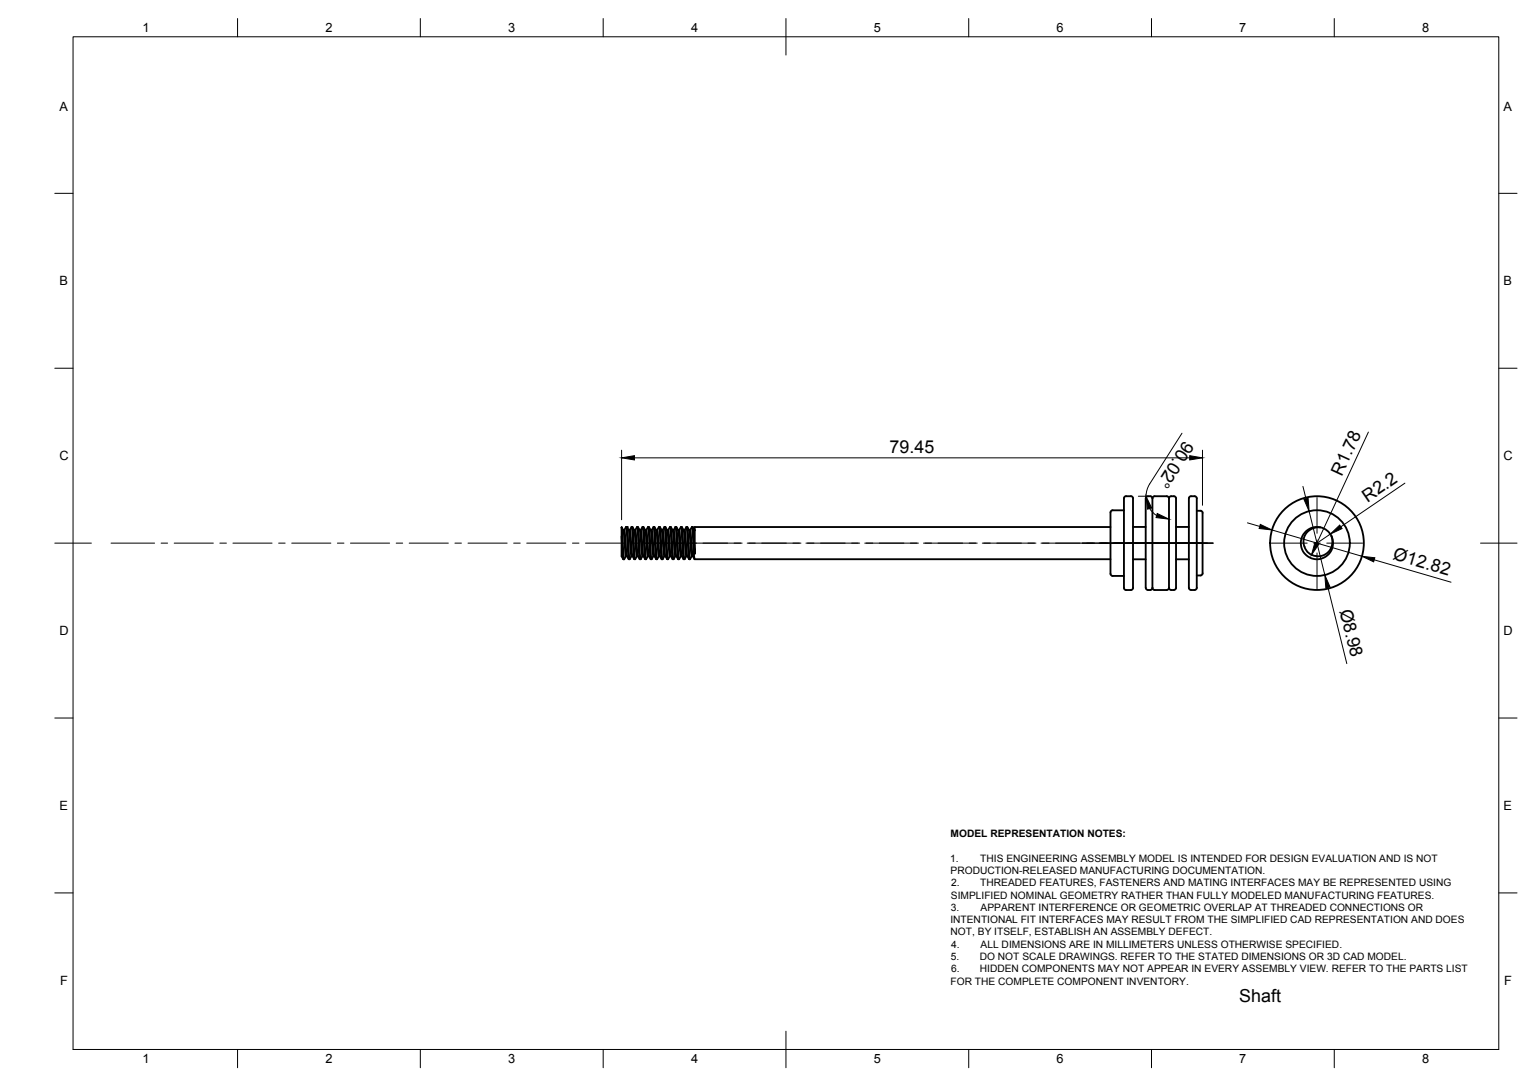
ISO-10303-21;
HEADER;
/* Generated by software containing ST-Developer
 * from STEP Tools, Inc. (www.steptools.com) 
 */

FILE_DESCRIPTION(
/* description */ (''),
/* implementation_level */ '2;1');

FILE_NAME(
/* name */ 'Shaft.step',
/* time_stamp */ '2026-10-06T13:05:37-07:00',
/* author */ (''),
/* organization */ (''),
/* preprocessor_version */ 'ST-DEVELOPER v20.2',
/* originating_system */ 'Autodesk Translation Framework v15.15.0.0',
/* authorisation */ '');

FILE_SCHEMA (('AUTOMOTIVE_DESIGN { 1 0 10303 214 3 1 1 }'));
ENDSEC;

DATA;
#10=MECHANICAL_DESIGN_GEOMETRIC_PRESENTATION_REPRESENTATION('',(#137),#28055);
#58=B_SPLINE_SURFACE_WITH_KNOTS('',3,3,((#14364,#14365,#14366,#14367,#14368,
#14369,#14370,#14371,#14372,#14373,#14374,#14375,#14376,#14377,#14378,#14379,
#14380,#14381,#14382,#14383,#14384,#14385,#14386,#14387,#14388,#14389,#14390,
#14391,#14392,#14393,#14394,#14395,#14396,#14397,#14398,#14399,#14400,#14401,
#14402,#14403,#14404,#14405,#14406,#14407,#14408,#14409,#14410,#14411,#14412,
#14413,#14414,#14415,#14416,#14417,#14418,#14419,#14420,#14421,#14422,#14423,
#14424,#14425,#14426,#14427,#14428,#14429,#14430,#14431,#14432,#14433,#14434,
#14435,#14436,#14437,#14438,#14439,#14440,#14441,#14442,#14443,#14444,#14445,
#14446,#14447,#14448,#14449,#14450,#14451,#14452),(#14453,#14454,#14455,
#14456,#14457,#14458,#14459,#14460,#14461,#14462,#14463,#14464,#14465,#14466,
#14467,#14468,#14469,#14470,#14471,#14472,#14473,#14474,#14475,#14476,#14477,
#14478,#14479,#14480,#14481,#14482,#14483,#14484,#14485,#14486,#14487,#14488,
#14489,#14490,#14491,#14492,#14493,#14494,#14495,#14496,#14497,#14498,#14499,
#14500,#14501,#14502,#14503,#14504,#14505,#14506,#14507,#14508,#14509,#14510,
#14511,#14512,#14513,#14514,#14515,#14516,#14517,#14518,#14519,#14520,#14521,
#14522,#14523,#14524,#14525,#14526,#14527,#14528,#14529,#14530,#14531,#14532,
#14533,#14534,#14535,#14536,#14537,#14538,#14539,#14540,#14541),(#14542,
#14543,#14544,#14545,#14546,#14547,#14548,#14549,#14550,#14551,#14552,#14553,
#14554,#14555,#14556,#14557,#14558,#14559,#14560,#14561,#14562,#14563,#14564,
#14565,#14566,#14567,#14568,#14569,#14570,#14571,#14572,#14573,#14574,#14575,
#14576,#14577,#14578,#14579,#14580,#14581,#14582,#14583,#14584,#14585,#14586,
#14587,#14588,#14589,#14590,#14591,#14592,#14593,#14594,#14595,#14596,#14597,
#14598,#14599,#14600,#14601,#14602,#14603,#14604,#14605,#14606,#14607,#14608,
#14609,#14610,#14611,#14612,#14613,#14614,#14615,#14616,#14617,#14618,#14619,
#14620,#14621,#14622,#14623,#14624,#14625,#14626,#14627,#14628,#14629,#14630),
(#14631,#14632,#14633,#14634,#14635,#14636,#14637,#14638,#14639,#14640,
#14641,#14642,#14643,#14644,#14645,#14646,#14647,#14648,#14649,#14650,#14651,
#14652,#14653,#14654,#14655,#14656,#14657,#14658,#14659,#14660,#14661,#14662,
#14663,#14664,#14665,#14666,#14667,#14668,#14669,#14670,#14671,#14672,#14673,
#14674,#14675,#14676,#14677,#14678,#14679,#14680,#14681,#14682,#14683,#14684,
#14685,#14686,#14687,#14688,#14689,#14690,#14691,#14692,#14693,#14694,#14695,
#14696,#14697,#14698,#14699,#14700,#14701,#14702,#14703,#14704,#14705,#14706,
#14707,#14708,#14709,#14710,#14711,#14712,#14713,#14714,#14715,#14716,#14717,
#14718,#14719)),.UNSPECIFIED.,.F.,.F.,.F.,(4,4),(4,1,1,1,1,1,1,1,1,1,1,
1,1,1,1,1,1,1,1,1,1,1,1,1,1,1,1,1,1,1,1,1,1,1,1,1,1,1,1,1,1,1,1,1,1,1,1,
1,1,1,1,1,1,1,1,1,1,1,1,1,1,1,1,1,1,1,1,1,1,1,1,1,1,1,1,1,1,1,1,1,1,1,1,
1,1,1,4),(-0.000373179544599254,0.0497114942005783),(13.3942556087771,14.3924503130856,
15.3906450173941,16.3888397217026,17.3870344260111,18.3852291303196,19.3834238346281,
20.3816185389366,21.3798132432451,22.3780079475536,23.3762026518621,24.3743973561706,
25.3725920604791,26.3707867647876,27.3689814690961,28.3671761734046,29.365370877713,
30.3635655820215,31.36176028633,32.3599549906385,33.358149694947,34.3563443992555,
35.354539103564,36.3527338078725,37.350928512181,38.3491232164895,39.347317920798,
40.3455126251065,41.343707329415,42.3419020337235,43.340096738032,44.3382914423405,
45.336486146649,46.3346808509575,47.332875555266,48.3310702595745,49.329264963883,
50.3274596681915,51.3256543725,52.3238490768085,53.322043781117,54.3202384854255,
55.318433189734,56.3166278940425,57.314822598351,58.3130173026595,59.311212006968,
60.3094067112765,61.307601415585,62.3057961198935,63.303990824202,64.3021855285105,
65.300380232819,66.2985749371275,67.296769641436,68.2949643457444,69.2931590500529,
70.2913537543614,71.2895484586699,72.2877431629784,73.2859378672869,74.2841325715954,
75.2823272759039,76.2805219802124,77.2787166845209,78.2769113888294,79.2751060931379,
80.2733007974464,81.2714955017549,82.2696902060634,83.2678849103719,84.2660796146804,
85.2642743189889,86.2624690232974,87.2606637276059,88.2588584319144,89.2570531362229,
90.2552478405314,91.2534425448399,92.2516372491484,93.2498319534569,94.2480266577654,
95.2462213620739,96.2444160663824,97.2426107706909,98.2408054749994,99.2393733588525),
 .UNSPECIFIED.);
#59=B_SPLINE_SURFACE_WITH_KNOTS('',3,3,((#14976,#14977,#14978,#14979,#14980,
#14981,#14982,#14983,#14984,#14985,#14986,#14987,#14988,#14989,#14990,#14991,
#14992,#14993,#14994,#14995,#14996,#14997,#14998,#14999,#15000,#15001,#15002,
#15003,#15004,#15005,#15006,#15007,#15008,#15009,#15010,#15011,#15012,#15013,
#15014,#15015,#15016,#15017,#15018,#15019,#15020,#15021,#15022,#15023,#15024,
#15025,#15026,#15027,#15028,#15029,#15030,#15031,#15032,#15033,#15034,#15035,
#15036,#15037,#15038,#15039,#15040,#15041,#15042,#15043,#15044,#15045,#15046,
#15047,#15048,#15049,#15050,#15051,#15052,#15053,#15054,#15055,#15056,#15057,
#15058,#15059,#15060,#15061,#15062,#15063,#15064),(#15065,#15066,#15067,
#15068,#15069,#15070,#15071,#15072,#15073,#15074,#15075,#15076,#15077,#15078,
#15079,#15080,#15081,#15082,#15083,#15084,#15085,#15086,#15087,#15088,#15089,
#15090,#15091,#15092,#15093,#15094,#15095,#15096,#15097,#15098,#15099,#15100,
#15101,#15102,#15103,#15104,#15105,#15106,#15107,#15108,#15109,#15110,#15111,
#15112,#15113,#15114,#15115,#15116,#15117,#15118,#15119,#15120,#15121,#15122,
#15123,#15124,#15125,#15126,#15127,#15128,#15129,#15130,#15131,#15132,#15133,
#15134,#15135,#15136,#15137,#15138,#15139,#15140,#15141,#15142,#15143,#15144,
#15145,#15146,#15147,#15148,#15149,#15150,#15151,#15152,#15153),(#15154,
#15155,#15156,#15157,#15158,#15159,#15160,#15161,#15162,#15163,#15164,#15165,
#15166,#15167,#15168,#15169,#15170,#15171,#15172,#15173,#15174,#15175,#15176,
#15177,#15178,#15179,#15180,#15181,#15182,#15183,#15184,#15185,#15186,#15187,
#15188,#15189,#15190,#15191,#15192,#15193,#15194,#15195,#15196,#15197,#15198,
#15199,#15200,#15201,#15202,#15203,#15204,#15205,#15206,#15207,#15208,#15209,
#15210,#15211,#15212,#15213,#15214,#15215,#15216,#15217,#15218,#15219,#15220,
#15221,#15222,#15223,#15224,#15225,#15226,#15227,#15228,#15229,#15230,#15231,
#15232,#15233,#15234,#15235,#15236,#15237,#15238,#15239,#15240,#15241,#15242),
(#15243,#15244,#15245,#15246,#15247,#15248,#15249,#15250,#15251,#15252,
#15253,#15254,#15255,#15256,#15257,#15258,#15259,#15260,#15261,#15262,#15263,
#15264,#15265,#15266,#15267,#15268,#15269,#15270,#15271,#15272,#15273,#15274,
#15275,#15276,#15277,#15278,#15279,#15280,#15281,#15282,#15283,#15284,#15285,
#15286,#15287,#15288,#15289,#15290,#15291,#15292,#15293,#15294,#15295,#15296,
#15297,#15298,#15299,#15300,#15301,#15302,#15303,#15304,#15305,#15306,#15307,
#15308,#15309,#15310,#15311,#15312,#15313,#15314,#15315,#15316,#15317,#15318,
#15319,#15320,#15321,#15322,#15323,#15324,#15325,#15326,#15327,#15328,#15329,
#15330,#15331)),.UNSPECIFIED.,.F.,.F.,.F.,(4,4),(4,1,1,1,1,1,1,1,1,1,1,
1,1,1,1,1,1,1,1,1,1,1,1,1,1,1,1,1,1,1,1,1,1,1,1,1,1,1,1,1,1,1,1,1,1,1,1,
1,1,1,1,1,1,1,1,1,1,1,1,1,1,1,1,1,1,1,1,1,1,1,1,1,1,1,1,1,1,1,1,1,1,1,1,
1,1,1,4),(-0.000317322289268298,0.0497654761150975),(16.7016191235447,17.7001869884391,
18.6983816927476,19.6965763970561,20.6947711013646,21.6929658056731,22.6911605099816,
23.6893552142901,24.6875499185986,25.6857446229071,26.6839393272156,27.6821340315241,
28.6803287358326,29.6785234401411,30.6767181444496,31.6749128487581,32.6731075530666,
33.6713022573751,34.6694969616836,35.6676916659921,36.6658863703006,37.6640810746091,
38.6622757789176,39.6604704832261,40.6586651875346,41.6568598918431,42.6550545961516,
43.65324930046,44.6514440047685,45.6496387090771,46.6478334133855,47.646028117694,
48.6442228220025,49.642417526311,50.6406122306195,51.638806934928,52.6370016392365,
53.635196343545,54.6333910478535,55.631585752162,56.6297804564705,57.627975160779,
58.6261698650875,59.624364569396,60.6225592737045,61.620753978013,62.6189486823215,
63.61714338663,64.6153380909385,65.613532795247,66.6117274995555,67.609922203864,
68.6081169081725,69.606311612481,70.6045063167895,71.602701021098,72.6008957254065,
73.599090429715,74.5972851340235,75.595479838332,76.5936745426405,77.591869246949,
78.5900639512575,79.588258655566,80.5864533598745,81.584648064183,82.5828427684915,
83.5810374728,84.5792321771085,85.577426881417,86.5756215857255,87.573816290034,
88.5720109943425,89.570205698651,90.5684004029595,91.566595107268,92.5647898115765,
93.562984515885,94.5611792201935,95.559373924502,96.5575686288105,97.555763333119,
98.5539580374275,99.552152741736,100.550347446044,101.548542150353,102.546736854661),
 .UNSPECIFIED.);
#98=TOROIDAL_SURFACE('',#3875,6.10845002480549,0.3);
#99=TOROIDAL_SURFACE('',#3881,6.107959450045,0.3);
#100=TOROIDAL_SURFACE('',#3887,4.18902817623056,0.3);
#101=TOROIDAL_SURFACE('',#3894,6.1096023907077,0.3);
#102=TOROIDAL_SURFACE('',#3901,6.10941276264524,0.3);
#103=TOROIDAL_SURFACE('',#3906,6.1087216021292,0.3);
#104=TOROIDAL_SURFACE('',#3914,6.1086273903848,0.3);
#105=TOROIDAL_SURFACE('',#3916,6.10778208446569,0.3);
#106=TOROIDAL_SURFACE('',#3921,6.10767319978801,0.3);
#107=TOROIDAL_SURFACE('',#3926,6.1069775362949,0.3);
#108=TOROIDAL_SURFACE('',#3934,6.10683442041659,0.3);
#109=TOROIDAL_SURFACE('',#3939,4.12329516333974,0.3);
#117=SHAPE_REPRESENTATION_RELATIONSHIP('SRR','None',#28094,#127);
#127=ADVANCED_BREP_SHAPE_REPRESENTATION('',(#147),#28046);
#137=STYLED_ITEM('',(#28152),#147);
#147=MANIFOLD_SOLID_BREP('Body1',#3678);
#164=CONICAL_SURFACE('',#3879,6.40820475053297,0.000295609290233083);
#165=CONICAL_SURFACE('',#3898,6.40950758978419,0.000295609290232241);
#166=CONICAL_SURFACE('',#3910,6.40867450936473,0.000295609290232273);
#167=CONICAL_SURFACE('',#3919,6.40772765523458,0.000295609290232245);
#168=CONICAL_SURFACE('',#3930,6.40690599146347,0.000295609290233429);
#181=FACE_BOUND('',#632,.T.);
#182=FACE_BOUND('',#635,.T.);
#183=FACE_BOUND('',#640,.T.);
#184=FACE_BOUND('',#648,.T.);
#185=FACE_BOUND('',#652,.T.);
#186=FACE_BOUND('',#655,.T.);
#187=FACE_BOUND('',#659,.T.);
#188=FACE_BOUND('',#665,.T.);
#189=FACE_BOUND('',#669,.T.);
#190=FACE_BOUND('',#672,.T.);
#209=PLANE('',#3872);
#210=PLANE('',#3883);
#211=PLANE('',#3885);
#212=PLANE('',#3886);
#213=PLANE('',#3893);
#214=PLANE('',#3900);
#215=PLANE('',#3904);
#216=PLANE('',#3912);
#217=PLANE('',#3924);
#218=PLANE('',#3932);
#219=PLANE('',#3937);
#220=PLANE('',#3943);
#280=CIRCLE('',#3853,1.77625);
#281=CIRCLE('',#3867,2.204);
#282=CIRCLE('',#3868,2.204);
#283=CIRCLE('',#3869,2.204);
#284=CIRCLE('',#3871,1.77625);
#285=CIRCLE('',#3873,6.107959450045);
#286=CIRCLE('',#3874,6.10778208446569);
#287=CIRCLE('',#3876,6.10845002480549);
#288=CIRCLE('',#3877,0.3);
#289=CIRCLE('',#3878,6.40845001169777);
#290=CIRCLE('',#3880,6.40795943693727);
#291=CIRCLE('',#3882,0.3);
#292=CIRCLE('',#3884,6.1086273903848);
#293=CIRCLE('',#3888,4.18902817623056);
#294=CIRCLE('',#3889,0.3);
#295=CIRCLE('',#3890,4.48902817623056);
#296=CIRCLE('',#3892,4.48902817623056);
#297=CIRCLE('',#3895,6.1096023907077);
#298=CIRCLE('',#3896,0.3);
#299=CIRCLE('',#3897,6.40960237759997);
#300=CIRCLE('',#3899,6.40941274953751);
#301=CIRCLE('',#3902,0.3);
#302=CIRCLE('',#3903,6.10941276264524);
#303=CIRCLE('',#3905,2.21164758166987);
#304=CIRCLE('',#3907,6.1087216021292);
#305=CIRCLE('',#3908,0.3);
#306=CIRCLE('',#3909,6.40872158902147);
#307=CIRCLE('',#3911,6.40862737727707);
#308=CIRCLE('',#3913,2.21164758166987);
#309=CIRCLE('',#3915,0.3);
#310=CIRCLE('',#3917,0.3);
#311=CIRCLE('',#3918,6.40778207135796);
#312=CIRCLE('',#3920,6.40767318668028);
#313=CIRCLE('',#3922,0.3);
#314=CIRCLE('',#3923,6.10767319978801);
#315=CIRCLE('',#3925,2.21164758166987);
#316=CIRCLE('',#3927,6.1069775362949);
#317=CIRCLE('',#3928,0.3);
#318=CIRCLE('',#3929,6.40697752318717);
#319=CIRCLE('',#3931,6.40683440730886);
#320=CIRCLE('',#3933,2.21164758166987);
#321=CIRCLE('',#3935,0.3);
#322=CIRCLE('',#3936,6.10683442041659);
#323=CIRCLE('',#3938,4.42329516333974);
#324=CIRCLE('',#3940,4.42329516333974);
#325=CIRCLE('',#3941,0.3);
#326=CIRCLE('',#3942,4.12329516333974);
#404=FACE_OUTER_BOUND('',#618,.T.);
#405=FACE_OUTER_BOUND('',#619,.T.);
#406=FACE_OUTER_BOUND('',#620,.T.);
#407=FACE_OUTER_BOUND('',#621,.T.);
#408=FACE_OUTER_BOUND('',#622,.T.);
#409=FACE_OUTER_BOUND('',#623,.T.);
#410=FACE_OUTER_BOUND('',#624,.T.);
#411=FACE_OUTER_BOUND('',#625,.T.);
#412=FACE_OUTER_BOUND('',#626,.T.);
#413=FACE_OUTER_BOUND('',#627,.T.);
#414=FACE_OUTER_BOUND('',#628,.T.);
#415=FACE_OUTER_BOUND('',#629,.T.);
#416=FACE_OUTER_BOUND('',#630,.T.);
#417=FACE_OUTER_BOUND('',#631,.T.);
#418=FACE_OUTER_BOUND('',#633,.T.);
#419=FACE_OUTER_BOUND('',#634,.T.);
#420=FACE_OUTER_BOUND('',#636,.T.);
#421=FACE_OUTER_BOUND('',#637,.T.);
#422=FACE_OUTER_BOUND('',#638,.T.);
#423=FACE_OUTER_BOUND('',#639,.T.);
#424=FACE_OUTER_BOUND('',#641,.T.);
#425=FACE_OUTER_BOUND('',#642,.T.);
#426=FACE_OUTER_BOUND('',#643,.T.);
#427=FACE_OUTER_BOUND('',#644,.T.);
#428=FACE_OUTER_BOUND('',#645,.T.);
#429=FACE_OUTER_BOUND('',#646,.T.);
#430=FACE_OUTER_BOUND('',#647,.T.);
#431=FACE_OUTER_BOUND('',#649,.T.);
#432=FACE_OUTER_BOUND('',#650,.T.);
#433=FACE_OUTER_BOUND('',#651,.T.);
#434=FACE_OUTER_BOUND('',#653,.T.);
#435=FACE_OUTER_BOUND('',#654,.T.);
#436=FACE_OUTER_BOUND('',#656,.T.);
#437=FACE_OUTER_BOUND('',#657,.T.);
#438=FACE_OUTER_BOUND('',#658,.T.);
#439=FACE_OUTER_BOUND('',#660,.T.);
#440=FACE_OUTER_BOUND('',#661,.T.);
#441=FACE_OUTER_BOUND('',#662,.T.);
#442=FACE_OUTER_BOUND('',#663,.T.);
#443=FACE_OUTER_BOUND('',#664,.T.);
#444=FACE_OUTER_BOUND('',#666,.T.);
#445=FACE_OUTER_BOUND('',#667,.T.);
#446=FACE_OUTER_BOUND('',#668,.T.);
#447=FACE_OUTER_BOUND('',#670,.T.);
#448=FACE_OUTER_BOUND('',#671,.T.);
#449=FACE_OUTER_BOUND('',#673,.T.);
#450=FACE_OUTER_BOUND('',#674,.T.);
#451=FACE_OUTER_BOUND('',#675,.T.);
#452=FACE_OUTER_BOUND('',#676,.T.);
#453=FACE_OUTER_BOUND('',#677,.T.);
#618=EDGE_LOOP('',(#2404,#2405,#2406,#2407,#2408));
#619=EDGE_LOOP('',(#2409,#2410,#2411,#2412,#2413));
#620=EDGE_LOOP('',(#2414,#2415,#2416,#2417,#2418,#2419));
#621=EDGE_LOOP('',(#2420,#2421,#2422,#2423,#2424,#2425));
#622=EDGE_LOOP('',(#2426,#2427,#2428,#2429,#2430));
#623=EDGE_LOOP('',(#2431,#2432,#2433,#2434,#2435));
#624=EDGE_LOOP('',(#2436,#2437,#2438,#2439,#2440));
#625=EDGE_LOOP('',(#2441,#2442,#2443,#2444,#2445));
#626=EDGE_LOOP('',(#2446,#2447,#2448,#2449,#2450));
#627=EDGE_LOOP('',(#2451,#2452,#2453,#2454,#2455));
#628=EDGE_LOOP('',(#2456,#2457,#2458,#2459,#2460));
#629=EDGE_LOOP('',(#2461,#2462,#2463,#2464,#2465));
#630=EDGE_LOOP('',(#2466,#2467,#2468,#2469,#2470,#2471));
#631=EDGE_LOOP('',(#2472));
#632=EDGE_LOOP('',(#2473,#2474,#2475,#2476,#2477,#2478,#2479,#2480,#2481,
#2482,#2483,#2484,#2485,#2486,#2487,#2488,#2489,#2490,#2491,#2492,#2493,
#2494,#2495,#2496,#2497,#2498,#2499,#2500,#2501,#2502,#2503));
#633=EDGE_LOOP('',(#2504,#2505,#2506,#2507,#2508,#2509));
#634=EDGE_LOOP('',(#2510));
#635=EDGE_LOOP('',(#2511));
#636=EDGE_LOOP('',(#2512,#2513,#2514,#2515));
#637=EDGE_LOOP('',(#2516,#2517,#2518,#2519));
#638=EDGE_LOOP('',(#2520,#2521,#2522,#2523));
#639=EDGE_LOOP('',(#2524));
#640=EDGE_LOOP('',(#2525));
#641=EDGE_LOOP('',(#2526,#2527,#2528,#2529,#2530,#2531,#2532,#2533,#2534,
#2535,#2536,#2537,#2538,#2539,#2540,#2541,#2542,#2543,#2544,#2545,#2546,
#2547,#2548,#2549,#2550,#2551,#2552,#2553,#2554,#2555,#2556,#2557,#2558,
#2559,#2560,#2561,#2562,#2563,#2564));
#642=EDGE_LOOP('',(#2565,#2566,#2567,#2568));
#643=EDGE_LOOP('',(#2569,#2570,#2571,#2572,#2573,#2574,#2575,#2576,#2577,
#2578,#2579,#2580,#2581,#2582,#2583,#2584,#2585,#2586,#2587,#2588,#2589,
#2590,#2591,#2592,#2593,#2594,#2595,#2596,#2597,#2598,#2599,#2600,#2601,
#2602,#2603,#2604,#2605,#2606,#2607,#2608));
#644=EDGE_LOOP('',(#2609,#2610,#2611,#2612));
#645=EDGE_LOOP('',(#2613,#2614,#2615,#2616));
#646=EDGE_LOOP('',(#2617,#2618,#2619,#2620));
#647=EDGE_LOOP('',(#2621));
#648=EDGE_LOOP('',(#2622));
#649=EDGE_LOOP('',(#2623,#2624,#2625,#2626));
#650=EDGE_LOOP('',(#2627,#2628,#2629,#2630));
#651=EDGE_LOOP('',(#2631));
#652=EDGE_LOOP('',(#2632));
#653=EDGE_LOOP('',(#2633,#2634,#2635,#2636));
#654=EDGE_LOOP('',(#2637));
#655=EDGE_LOOP('',(#2638));
#656=EDGE_LOOP('',(#2639,#2640,#2641,#2642));
#657=EDGE_LOOP('',(#2643,#2644,#2645,#2646));
#658=EDGE_LOOP('',(#2647));
#659=EDGE_LOOP('',(#2648));
#660=EDGE_LOOP('',(#2649,#2650,#2651,#2652));
#661=EDGE_LOOP('',(#2653,#2654,#2655,#2656));
#662=EDGE_LOOP('',(#2657,#2658,#2659,#2660));
#663=EDGE_LOOP('',(#2661,#2662,#2663,#2664));
#664=EDGE_LOOP('',(#2665));
#665=EDGE_LOOP('',(#2666));
#666=EDGE_LOOP('',(#2667,#2668,#2669,#2670));
#667=EDGE_LOOP('',(#2671,#2672,#2673,#2674));
#668=EDGE_LOOP('',(#2675));
#669=EDGE_LOOP('',(#2676));
#670=EDGE_LOOP('',(#2677,#2678,#2679,#2680));
#671=EDGE_LOOP('',(#2681));
#672=EDGE_LOOP('',(#2682));
#673=EDGE_LOOP('',(#2683,#2684,#2685,#2686));
#674=EDGE_LOOP('',(#2687));
#675=EDGE_LOOP('',(#2688,#2689,#2690,#2691));
#676=EDGE_LOOP('',(#2692,#2693,#2694,#2695));
#677=EDGE_LOOP('',(#2696,#2697,#2698,#2699));
#840=LINE('',#5074,#998);
#841=LINE('',#5346,#999);
#842=LINE('',#5736,#1000);
#843=LINE('',#5862,#1001);
#844=LINE('',#6173,#1002);
#845=LINE('',#6561,#1003);
#846=LINE('',#6960,#1004);
#847=LINE('',#7347,#1005);
#848=LINE('',#7748,#1006);
#849=LINE('',#8143,#1007);
#850=LINE('',#8552,#1008);
#851=LINE('',#8955,#1009);
#852=LINE('',#9337,#1010);
#853=LINE('',#14357,#1011);
#854=LINE('',#15429,#1012);
#855=LINE('',#15440,#1013);
#856=LINE('',#15458,#1014);
#857=LINE('',#15471,#1015);
#858=LINE('',#15488,#1016);
#859=LINE('',#15508,#1017);
#860=LINE('',#15510,#1018);
#861=LINE('',#15512,#1019);
#998=VECTOR('',#4239,1.77625);
#999=VECTOR('',#4244,1.77625);
#1000=VECTOR('',#4247,1.77625);
#1001=VECTOR('',#4250,1.77625);
#1002=VECTOR('',#4253,1.77625);
#1003=VECTOR('',#4256,1.77625);
#1004=VECTOR('',#4259,1.77625);
#1005=VECTOR('',#4262,1.77625);
#1006=VECTOR('',#4265,1.77625);
#1007=VECTOR('',#4268,1.77625);
#1008=VECTOR('',#4271,1.77625);
#1009=VECTOR('',#4274,1.77625);
#1010=VECTOR('',#4277,1.77625);
#1011=VECTOR('',#4306,6.40820475053297);
#1012=VECTOR('',#4331,4.48902817623056);
#1013=VECTOR('',#4346,6.40950758978419);
#1014=VECTOR('',#4371,6.40867450936473);
#1015=VECTOR('',#4390,6.40772765523458);
#1016=VECTOR('',#4413,6.40690599146347);
#1017=VECTOR('',#4442,4.42329516333974);
#1018=VECTOR('',#4445,2.21164758166987);
#1019=VECTOR('',#4448,2.21164758166987);
#1141=B_SPLINE_CURVE_WITH_KNOTS('',3,(#5076,#5077,#5078,#5079,#5080,#5081,
#5082,#5083,#5084,#5085,#5086,#5087,#5088,#5089,#5090,#5091,#5092,#5093,
#5094,#5095,#5096,#5097,#5098,#5099,#5100,#5101,#5102,#5103,#5104,#5105,
#5106,#5107,#5108,#5109,#5110,#5111,#5112,#5113,#5114,#5115,#5116,#5117,
#5118,#5119,#5120,#5121,#5122,#5123,#5124,#5125,#5126,#5127,#5128,#5129,
#5130,#5131,#5132,#5133,#5134,#5135,#5136,#5137,#5138,#5139,#5140,#5141,
#5142,#5143,#5144,#5145,#5146,#5147,#5148,#5149,#5150,#5151,#5152,#5153,
#5154,#5155,#5156,#5157,#5158,#5159,#5160,#5161,#5162,#5163,#5164,#5165,
#5166,#5167,#5168,#5169,#5170,#5171,#5172,#5173,#5174,#5175,#5176,#5177,
#5178,#5179,#5180,#5181,#5182,#5183,#5184,#5185,#5186,#5187,#5188,#5189,
#5190,#5191,#5192,#5193,#5194,#5195,#5196,#5197,#5198,#5199,#5200,#5201,
#5202,#5203,#5204,#5205,#5206,#5207,#5208,#5209,#5210,#5211,#5212,#5213,
#5214,#5215,#5216,#5217,#5218,#5219,#5220,#5221,#5222,#5223),
 .UNSPECIFIED.,.F.,.F.,(4,2,2,2,2,2,2,2,2,2,2,2,2,2,2,2,2,2,2,2,2,2,2,2,
2,2,2,2,2,2,2,2,2,2,2,2,2,2,2,2,2,2,2,2,2,2,2,2,2,2,2,2,2,2,2,2,2,2,2,2,
2,2,2,2,2,2,2,2,2,2,2,2,2,4),(-0.835356566537246,-0.834179578002919,-0.832057305629885,
-0.82934175770569,-0.823544728796445,-0.815449054574031,-0.790979904521206,
-0.758630520976316,-0.751247845401951,-0.746562671739766,-0.7427957472337,
-0.738457675321842,-0.730730673891037,-0.705406951032464,-0.667022076483651,
-0.660027153413853,-0.657302375275477,-0.655127611169892,-0.652797944555009,
-0.648926745100182,-0.632840827180127,-0.581115393054966,-0.57367752973655,
-0.568973506689807,-0.565200732382815,-0.560865809230101,-0.55317110435513,
-0.528123923872481,-0.491328745297315,-0.482817000286532,-0.479581086366103,
-0.477413245958042,-0.475106128977813,-0.471268591582215,-0.455353920220774,
-0.406196234245469,-0.39585526201539,-0.391035642446638,-0.38727899810539,
-0.3830778783461,-0.375924745588849,-0.367161529927778,-0.347550182457797,
-0.318343151462567,-0.305702905197989,-0.302000513660807,-0.299719364921067,
-0.297497437811916,-0.294122055897232,-0.283819597360589,-0.265015419181205,
-0.224003622448924,-0.216331810091993,-0.211947796786676,-0.20854279480949,
-0.204038955946528,-0.195556237330191,-0.184620571805917,-0.155613520886967,
-0.130863977628998,-0.12539325974147,-0.12272421983817,-0.12056335417637,
-0.117801735198089,-0.111949409671634,-0.0861381627528235,-0.0532557845040427,
-0.0423421159714301,-0.0374256406153841,-0.0335867130961813,-0.0300163926963186,
-0.0258468770318152,-0.0165211006533095,-0.000528019587408642),
 .UNSPECIFIED.);
#1142=B_SPLINE_CURVE_WITH_KNOTS('',3,(#5225,#5226,#5227,#5228,#5229,#5230,
#5231),.UNSPECIFIED.,.F.,.F.,(4,3,4),(15.4636264665944,15.5857948670228,
15.7079632674512),.UNSPECIFIED.);
#1143=B_SPLINE_CURVE_WITH_KNOTS('',3,(#5234,#5235,#5236,#5237,#5238,#5239,
#5240,#5241,#5242,#5243,#5244,#5245,#5246,#5247,#5248,#5249,#5250,#5251,
#5252,#5253,#5254,#5255,#5256,#5257,#5258,#5259,#5260,#5261,#5262,#5263,
#5264,#5265,#5266,#5267,#5268,#5269,#5270,#5271,#5272,#5273,#5274,#5275,
#5276,#5277,#5278,#5279,#5280,#5281,#5282,#5283,#5284,#5285,#5286,#5287,
#5288,#5289,#5290,#5291,#5292,#5293,#5294,#5295,#5296,#5297,#5298,#5299,
#5300,#5301,#5302,#5303,#5304,#5305,#5306,#5307,#5308,#5309,#5310,#5311,
#5312,#5313,#5314,#5315,#5316,#5317,#5318,#5319,#5320,#5321,#5322,#5323,
#5324,#5325,#5326,#5327,#5328,#5329,#5330,#5331,#5332,#5333,#5334,#5335,
#5336,#5337,#5338,#5339,#5340,#5341,#5342),.UNSPECIFIED.,.F.,.F.,(4,3,3,
3,3,3,3,3,3,3,3,3,3,3,3,3,3,3,3,3,3,3,3,3,3,3,3,3,3,3,3,3,3,3,3,3,4),(16.7019922841306,
16.8124544772726,16.9234210411684,17.033796869599,17.1441744311209,17.2545854631975,
17.3659858445079,17.4766375907132,17.5884122895762,17.7001869884391,17.8072802155964,
17.9186679002403,18.0254288144202,18.1321132984658,18.2387615669814,18.3454137772225,
18.4521802784855,18.5590147146697,18.6660336585631,18.6983816927476,18.8065090728564,
18.9177674883813,19.025595407644,19.1333563054358,19.2410888397907,19.3488316227747,
19.4566913005886,19.5646218816293,19.6727314597256,19.6965763970561,19.8047706499335,
19.912813978709,20.0207451306855,20.1286177204737,20.2364557658273,20.3443346961532,
20.3930532338378),.UNSPECIFIED.);
#1144=B_SPLINE_CURVE_WITH_KNOTS('',3,(#5347,#5348,#5349,#5350,#5351,#5352,
#5353,#5354,#5355,#5356,#5357,#5358,#5359,#5360,#5361,#5362,#5363,#5364,
#5365,#5366,#5367,#5368,#5369,#5370,#5371,#5372,#5373,#5374,#5375,#5376,
#5377,#5378,#5379,#5380,#5381,#5382,#5383,#5384,#5385,#5386,#5387,#5388,
#5389,#5390,#5391,#5392,#5393,#5394,#5395,#5396,#5397,#5398,#5399,#5400,
#5401,#5402,#5403,#5404,#5405,#5406,#5407,#5408,#5409,#5410,#5411,#5412,
#5413,#5414,#5415,#5416,#5417,#5418,#5419,#5420,#5421,#5422,#5423,#5424,
#5425,#5426,#5427,#5428,#5429,#5430,#5431,#5432,#5433,#5434,#5435,#5436,
#5437,#5438,#5439,#5440,#5441,#5442,#5443,#5444,#5445,#5446,#5447,#5448,
#5449,#5450,#5451,#5452,#5453,#5454,#5455,#5456,#5457,#5458,#5459,#5460,
#5461,#5462,#5463,#5464,#5465,#5466,#5467,#5468,#5469,#5470,#5471,#5472,
#5473,#5474,#5475,#5476,#5477,#5478,#5479,#5480,#5481,#5482,#5483,#5484,
#5485,#5486,#5487,#5488,#5489,#5490,#5491,#5492,#5493,#5494,#5495,#5496,
#5497,#5498,#5499,#5500,#5501,#5502,#5503,#5504,#5505,#5506,#5507,#5508,
#5509,#5510,#5511,#5512,#5513,#5514,#5515,#5516,#5517,#5518,#5519,#5520,
#5521,#5522,#5523,#5524,#5525,#5526,#5527,#5528,#5529,#5530,#5531,#5532,
#5533,#5534,#5535,#5536,#5537,#5538,#5539,#5540),.UNSPECIFIED.,.F.,.F.,
(4,2,2,2,2,2,2,2,2,2,2,2,2,2,2,2,2,2,2,2,2,2,2,2,2,2,2,2,2,2,2,2,2,2,2,
2,2,2,2,2,2,2,2,2,2,2,2,2,2,2,2,2,2,2,2,2,2,2,2,2,2,2,2,2,2,2,2,2,2,2,2,
2,2,2,2,2,2,2,2,2,2,2,2,2,2,2,2,2,2,2,2,2,2,2,2,2,4),(-1.95454507750439,
-1.92969887688555,-1.90700587487671,-1.90284449273311,-1.90045698570642,
-1.89829258749123,-1.89520508387779,-1.88936360059004,-1.85017890081121,
-1.82470793213726,-1.81696215744342,-1.81262184818882,-1.80885764965132,
-1.80418199299687,-1.79682683246125,-1.76279416764177,-1.73956966484566,
-1.73169570283323,-1.72601764868932,-1.72332439775519,-1.72120226710614,
-1.71856614706167,-1.7131897934261,-1.68420858229177,-1.66980886534623,
-1.65294595377729,-1.64134625560956,-1.63629734544878,-1.63249199363362,
-1.62836280128111,-1.62163051869468,-1.59092369606964,-1.5680581423284,
-1.55098317581711,-1.54705937226041,-1.54472310228857,-1.54256020421295,
-1.53987248019897,-1.53309414208251,-1.49446663046274,-1.46909648525411,
-1.46136459634652,-1.45702729073491,-1.45326306026007,-1.44858395184908,
-1.44121641047095,-1.40788434579373,-1.3841471969067,-1.37618087956058,
-1.37045355392296,-1.3677512422959,-1.36562903738565,-1.3630016479163,-1.35767008544244,
-1.3177711925292,-1.29148760005246,-1.28363221952914,-1.27926932868241,
-1.27550681445262,-1.27086060774184,-1.26360717745568,-1.22625306573836,
-1.2053446946898,-1.19438739470466,-1.19094604449721,-1.18871382456224,
-1.18643941074527,-1.18280332363237,-1.17100933713551,-1.13755203671263,
-1.12000271682831,-1.10834732008514,-1.10366159282688,-1.09980654930369,
-1.09585161550517,-1.08996582836221,-1.07189826280532,-1.03983979736194,
-1.01808202486886,-1.01388329213852,-1.01148758987828,-1.00932756295218,
-1.00626130276856,-0.998311944972997,-0.985704858969611,-0.961762341328657,
-0.933727639097285,-0.927057916080415,-0.922943834088199,-0.919137263230214,
-0.914064099371912,-0.902299995493179,-0.885082792620805,-0.873876918369987,
-0.842062810475459,-0.836793926929779,-0.835356566537246),.UNSPECIFIED.);
#1145=B_SPLINE_CURVE_WITH_KNOTS('',3,(#5542,#5543,#5544,#5545,#5546,#5547,
#5548,#5549,#5550,#5551,#5552,#5553,#5554,#5555,#5556,#5557,#5558,#5559,
#5560,#5561,#5562,#5563,#5564,#5565,#5566,#5567,#5568,#5569,#5570,#5571,
#5572,#5573,#5574,#5575,#5576,#5577,#5578,#5579,#5580,#5581,#5582,#5583,
#5584,#5585,#5586,#5587,#5588,#5589,#5590),.UNSPECIFIED.,.F.,.F.,(4,3,3,
3,3,3,3,3,3,3,3,3,3,3,3,3,4),(20.3930532338378,20.5010566943853,20.6092613750708,
20.6947711013646,20.8026970972416,20.9139806857955,21.0216059003609,21.1291641701826,
21.2366944839657,21.3442357847572,21.4518963786598,21.5596290516459,21.6675442181706,
21.6929658056731,21.8250574021607,21.9552551911513,21.9911485745994),
 .UNSPECIFIED.);
#1146=B_SPLINE_CURVE_WITH_KNOTS('',3,(#5591,#5592,#5593,#5594,#5595,#5596,
#5597,#5598,#5599,#5600,#5601,#5602,#5603,#5604,#5605,#5606,#5607,#5608,
#5609,#5610,#5611,#5612,#5613,#5614,#5615,#5616,#5617,#5618,#5619,#5620,
#5621,#5622,#5623,#5624,#5625,#5626,#5627,#5628,#5629,#5630,#5631,#5632,
#5633,#5634,#5635,#5636,#5637,#5638,#5639,#5640,#5641,#5642,#5643,#5644,
#5645,#5646,#5647,#5648,#5649,#5650,#5651,#5652,#5653,#5654,#5655,#5656,
#5657,#5658,#5659,#5660,#5661,#5662,#5663,#5664,#5665,#5666,#5667,#5668,
#5669,#5670,#5671,#5672,#5673,#5674,#5675,#5676,#5677,#5678,#5679,#5680,
#5681,#5682,#5683,#5684,#5685,#5686,#5687,#5688,#5689,#5690,#5691,#5692,
#5693,#5694,#5695,#5696,#5697,#5698,#5699,#5700,#5701,#5702,#5703,#5704,
#5705,#5706,#5707,#5708,#5709,#5710,#5711,#5712,#5713,#5714,#5715,#5716,
#5717,#5718,#5719,#5720,#5721,#5722,#5723,#5724,#5725,#5726,#5727,#5728,
#5729,#5730,#5731,#5732),.UNSPECIFIED.,.F.,.F.,(4,3,3,3,3,3,3,3,3,3,3,3,
3,3,3,3,3,3,3,3,3,3,3,3,3,3,3,3,3,3,3,3,3,3,3,3,3,3,3,3,3,3,3,3,3,3,3,4),
(21.9911485751285,22.0981765274336,22.2051623507136,22.3121457608551,22.4192405673634,
22.5263967550779,22.6337465274261,22.6911605099816,22.7992205091258,22.9104873472713,
23.0182513855477,23.1259498862704,23.2336216180078,23.3413053050867,23.4491088121582,
23.5569848760485,23.6650428436122,23.6893552142901,23.7973810979624,23.9086522005419,
24.0163805862326,24.1240429630528,24.2316781568489,24.3393249487448,24.4470912677292,
24.5549299286194,24.6629505155869,24.6875499185986,24.7955941221079,24.9068629347078,
25.0146102076539,25.1222916298659,25.2299459967969,25.3376120593305,25.4453976697339,
25.5532556566589,25.6612954465704,25.6857446229071,25.7937879777517,25.904155195045,
26.0119016507377,26.1195817394621,26.2272342594645,26.3396071236228,26.4473901517118,
26.5552467306643,26.6632787454227,26.6767257160977),.UNSPECIFIED.);
#1147=B_SPLINE_CURVE_WITH_KNOTS('',3,(#5738,#5739,#5740,#5741,#5742,#5743,
#5744,#5745,#5746),.UNSPECIFIED.,.F.,.F.,(4,1,1,1,1,1,4),(28.274333882308,
28.3671761734046,29.365370877713,30.3635655820215,31.36176028633,32.3599549906385,
32.9594405895371),.UNSPECIFIED.);
#1148=B_SPLINE_CURVE_WITH_KNOTS('',3,(#5747,#5748,#5749,#5750,#5751,#5752,
#5753,#5754,#5755,#5756,#5757,#5758,#5759,#5760,#5761,#5762,#5763,#5764,
#5765,#5766,#5767,#5768,#5769,#5770,#5771,#5772,#5773,#5774,#5775,#5776,
#5777,#5778,#5779,#5780,#5781,#5782,#5783,#5784,#5785,#5786,#5787,#5788,
#5789,#5790,#5791,#5792,#5793,#5794,#5795,#5796),.UNSPECIFIED.,.F.,.F.,
(4,2,2,2,2,2,2,2,2,2,2,2,2,2,2,2,2,2,2,2,2,2,2,2,4),(-2.23915986394093,
-2.20592704873654,-2.18032577745133,-2.17256259015734,-2.16821888680587,
-2.16445526260495,-2.15978487840366,-2.15244732829037,-2.1175945351571,
-2.09496188142004,-2.08719720497901,-2.08157791702537,-2.07889578751457,
-2.07677406554045,-2.0741280407893,-2.06869901710893,-2.04323247885477,
-2.02010812726836,-1.99943956922362,-1.99331541844904,-1.98931322858529,
-1.98549354859668,-1.98011485708538,-1.96718673212748,-1.95454507750439),
 .UNSPECIFIED.);
#1149=B_SPLINE_CURVE_WITH_KNOTS('',3,(#5798,#5799,#5800,#5801,#5802,#5803,
#5804,#5805,#5806,#5807,#5808,#5809,#5810,#5811,#5812,#5813,#5814,#5815,
#5816,#5817,#5818,#5819,#5820,#5821,#5822,#5823,#5824,#5825,#5826,#5827,
#5828,#5829,#5830,#5831,#5832,#5833,#5834,#5835,#5836,#5837,#5838,#5839,
#5840,#5841,#5842,#5843,#5844,#5845,#5846,#5847,#5848,#5849),
 .UNSPECIFIED.,.F.,.F.,(4,3,3,3,3,3,3,3,3,3,3,3,3,3,3,3,3,4),(26.6767257160977,
26.6839393272156,26.7919782863231,26.9032477544733,27.0109896752984,27.1186657202993,
27.2263146935872,27.3339753546827,27.4417555868768,27.5496082029795,27.6576426811105,
27.6821340315241,27.7919683102848,27.9016171368834,28.0110886501516,28.1204564526687,
28.2297536032295,28.274333882308),.UNSPECIFIED.);
#1150=B_SPLINE_CURVE_WITH_KNOTS('',3,(#5850,#5851,#5852,#5853,#5854,#5855,
#5856,#5857,#5858),.UNSPECIFIED.,.F.,.F.,(4,1,1,1,1,1,4),(28.2743402347403,
28.6803287358326,29.6785234401411,30.6767181444496,31.6749128487581,32.6731075530666,
32.9608271762519),.UNSPECIFIED.);
#1151=B_SPLINE_CURVE_WITH_KNOTS('',3,(#5864,#5865,#5866,#5867,#5868,#5869,
#5870,#5871,#5872,#5873,#5874,#5875,#5876,#5877,#5878,#5879,#5880,#5881,
#5882,#5883,#5884,#5885,#5886,#5887,#5888,#5889,#5890,#5891,#5892,#5893,
#5894,#5895,#5896,#5897,#5898,#5899,#5900,#5901,#5902,#5903,#5904,#5905,
#5906,#5907,#5908,#5909,#5910,#5911,#5912,#5913,#5914,#5915,#5916,#5917,
#5918,#5919,#5920,#5921,#5922,#5923,#5924,#5925,#5926,#5927,#5928,#5929,
#5930,#5931,#5932,#5933,#5934,#5935,#5936,#5937,#5938,#5939,#5940,#5941,
#5942,#5943,#5944,#5945,#5946,#5947,#5948,#5949,#5950,#5951,#5952,#5953,
#5954,#5955,#5956,#5957,#5958,#5959,#5960,#5961,#5962,#5963,#5964,#5965,
#5966,#5967,#5968,#5969,#5970,#5971,#5972,#5973,#5974,#5975,#5976,#5977,
#5978,#5979,#5980,#5981,#5982,#5983,#5984,#5985,#5986,#5987,#5988,#5989,
#5990,#5991,#5992,#5993,#5994,#5995,#5996,#5997,#5998,#5999,#6000,#6001,
#6002,#6003,#6004,#6005),.UNSPECIFIED.,.F.,.F.,(4,3,3,3,3,3,3,3,3,3,3,3,
3,3,3,3,3,3,3,3,3,3,3,3,3,3,3,3,3,3,3,3,3,3,3,3,3,3,3,3,3,3,3,3,3,3,3,4),
(34.5575193977698,34.6637962689209,34.7699803795124,34.8761126116981,34.9822337650756,
35.088455256206,35.194732459932,35.3011944966565,35.354539103564,35.4625799721229,
35.5738492015916,35.681593103219,35.7892711499964,35.8969221428487,36.0045848381315,
36.112367113131,36.2202217794645,36.3282583002447,36.3527338078725,36.4607746770588,
36.5720439064491,36.6797878087295,36.7874658561678,36.8951168496875,37.0027795456435,
37.1105618213201,37.2184164883337,37.3264530097926,37.350928512181,37.4589693811155,
37.5702386105372,37.6779825125593,37.7856605597373,37.8933115529956,38.000974248689,
38.1087565241035,38.216611190855,38.324647712054,38.3491232164895,38.4608178024709,
38.568667102327,38.6764084850113,38.7840808451954,38.8917229858393,38.9994241461165,
39.1071616534688,39.2150320522313,39.2426799043403),.UNSPECIFIED.);
#1152=B_SPLINE_CURVE_WITH_KNOTS('',3,(#6006,#6007,#6008,#6009,#6010,#6011),
 .UNSPECIFIED.,.F.,.F.,(4,1,1,4),(32.9594405895371,33.358149694947,34.3563443992555,
34.5575191894877),.UNSPECIFIED.);
#1153=B_SPLINE_CURVE_WITH_KNOTS('',3,(#6013,#6014,#6015,#6016,#6017),
 .UNSPECIFIED.,.F.,.F.,(4,1,4),(32.9608271762519,33.6713022573751,34.5575102647709),
 .UNSPECIFIED.);
#1154=B_SPLINE_CURVE_WITH_KNOTS('',3,(#6018,#6019,#6020,#6021,#6022,#6023,
#6024,#6025,#6026,#6027,#6028,#6029,#6030,#6031,#6032,#6033,#6034,#6035,
#6036,#6037,#6038,#6039,#6040,#6041,#6042,#6043,#6044,#6045,#6046,#6047,
#6048,#6049,#6050,#6051,#6052,#6053,#6054,#6055,#6056,#6057,#6058,#6059,
#6060,#6061,#6062,#6063,#6064,#6065,#6066,#6067,#6068,#6069,#6070,#6071,
#6072,#6073,#6074,#6075,#6076,#6077,#6078,#6079,#6080,#6081,#6082,#6083,
#6084,#6085,#6086,#6087,#6088,#6089,#6090,#6091,#6092,#6093,#6094,#6095,
#6096,#6097,#6098,#6099,#6100,#6101,#6102,#6103,#6104,#6105,#6106,#6107,
#6108,#6109,#6110,#6111,#6112,#6113,#6114,#6115,#6116,#6117,#6118,#6119,
#6120,#6121,#6122,#6123,#6124,#6125,#6126,#6127,#6128,#6129,#6130,#6131,
#6132,#6133,#6134,#6135,#6136,#6137,#6138,#6139,#6140,#6141,#6142,#6143,
#6144,#6145,#6146,#6147,#6148,#6149,#6150,#6151,#6152,#6153,#6154,#6155,
#6156,#6157,#6158,#6159,#6160,#6161,#6162,#6163,#6164,#6165,#6166,#6167,
#6168,#6169),.UNSPECIFIED.,.F.,.F.,(4,2,2,2,2,2,2,2,2,2,2,2,2,2,2,2,2,2,
2,2,2,2,2,2,2,2,2,2,2,2,2,2,2,2,2,2,2,2,2,2,2,2,2,2,2,2,2,2,2,2,2,2,2,2,
2,2,2,2,2,2,2,2,2,2,2,2,2,2,2,2,2,2,2,2,2,4),(-2.23888494972284,-2.22991776855793,
-2.22447064320661,-2.22191829216988,-2.21989477343009,-2.21776847377992,
-2.21502874476971,-2.20893402279126,-2.18787843436243,-2.16966634347861,
-2.14385238080136,-2.13606038366673,-2.13171077947681,-2.12794768118234,
-2.12328524358438,-2.11390205737419,-2.07246864712722,-2.05027458125105,
-2.04489827929598,-2.04226229222838,-2.04035089005686,-2.03776646712269,
-2.0328105326407,-1.99791659798478,-1.96864883524523,-1.95927121403217,
-1.95460974539526,-1.95084658102242,-1.94649595728929,-1.93891035281729,
-1.89754680244139,-1.87904083706616,-1.86884897296706,-1.86549209633338,
-1.86327753791409,-1.86098243262719,-1.85724781425568,-1.84435404247657,
-1.80361547729748,-1.78470675362083,-1.77873969519656,-1.77476942506272,
-1.77092850577831,-1.76629564503759,-1.75480186338448,-1.71587013709037,
-1.69449471669221,-1.6892066322397,-1.68658769916922,-1.68467704547633,
-1.68207654389007,-1.67688276164301,-1.64448591367606,-1.63262573013931,
-1.61610562983729,-1.60466923401097,-1.59964695878773,-1.59584552599926,
-1.59170494698949,-1.5849177429812,-1.554669575998,-1.53244795233212,-1.51446840999572,
-1.51049555511708,-1.50814869586371,-1.50599106650872,-1.50332518743687,
-1.49656138600397,-1.45787430738769,-1.43249347062081,-1.42475990429867,
-1.42042205696215,-1.41665756715559,-1.4119784002815,-1.4046112824739,-1.40437359183403),
 .UNSPECIFIED.);
#1155=B_SPLINE_CURVE_WITH_KNOTS('',3,(#6175,#6176,#6177,#6178,#6179,#6180,
#6181,#6182,#6183,#6184,#6185,#6186,#6187,#6188,#6189,#6190,#6191,#6192,
#6193,#6194,#6195,#6196,#6197,#6198,#6199,#6200,#6201,#6202,#6203,#6204,
#6205,#6206,#6207,#6208,#6209,#6210,#6211,#6212,#6213,#6214,#6215,#6216,
#6217,#6218,#6219,#6220,#6221,#6222,#6223,#6224,#6225,#6226,#6227,#6228,
#6229,#6230,#6231,#6232,#6233,#6234,#6235,#6236,#6237,#6238,#6239,#6240,
#6241,#6242,#6243,#6244,#6245,#6246,#6247,#6248,#6249,#6250,#6251,#6252,
#6253,#6254,#6255,#6256,#6257,#6258,#6259,#6260,#6261,#6262,#6263,#6264,
#6265,#6266,#6267,#6268,#6269,#6270,#6271,#6272,#6273,#6274,#6275,#6276,
#6277,#6278,#6279,#6280,#6281,#6282,#6283,#6284,#6285,#6286,#6287,#6288,
#6289,#6290,#6291,#6292,#6293,#6294,#6295,#6296,#6297,#6298,#6299,#6300,
#6301,#6302,#6303,#6304,#6305,#6306,#6307,#6308,#6309,#6310,#6311,#6312,
#6313,#6314,#6315,#6316,#6317,#6318,#6319,#6320,#6321,#6322),
 .UNSPECIFIED.,.F.,.F.,(4,2,2,2,2,2,2,2,2,2,2,2,2,2,2,2,2,2,2,2,2,2,2,2,
2,2,2,2,2,2,2,2,2,2,2,2,2,2,2,2,2,2,2,2,2,2,2,2,2,2,2,2,2,2,2,2,2,2,2,2,
2,2,2,2,2,2,2,2,2,2,2,2,2,4),(-0.835099924428374,-0.810230319348001,-0.804896130565269,
-0.802268377014195,-0.800146299250092,-0.797444671956707,-0.791720718154825,
-0.783761495584802,-0.76005780011584,-0.726728468131525,-0.719363533194796,
-0.714685219878248,-0.71092110576457,-0.70658334156592,-0.69884901195783,
-0.673458960429975,-0.634756499650488,-0.627989293535211,-0.625322962005017,
-0.623165325271974,-0.620818865337488,-0.616847515854485,-0.59888758745142,
-0.576676092912076,-0.54644768251051,-0.539660204241827,-0.535519716308051,
-0.531718510580919,-0.526696749457739,-0.515262844600596,-0.498745486707646,
-0.487103824026872,-0.454413034292759,-0.449239542055546,-0.446643067818346,
-0.444732272546319,-0.442109216499667,-0.436799720433161,-0.415227032788622,
-0.375690485550125,-0.364600414407815,-0.359688848510703,-0.355891171960493,
-0.35173917187912,-0.344896737736136,-0.336636791651806,-0.318863385154281,
-0.284112077379857,-0.273620116100306,-0.270127168635037,-0.268106390492079,
-0.265898441440772,-0.262574397053666,-0.252664479586328,-0.234986866661226,
-0.19213003390502,-0.184740608673265,-0.180432716329455,-0.176701275542952,
-0.171998743506043,-0.16240040782514,-0.138024613707217,-0.10870919764151,
-0.0962332329690868,-0.0925351436016178,-0.0902480445649851,-0.0880276089129058,
-0.0846416658687451,-0.074190627067205,-0.0548973537364689,-0.0155466790190831,
-0.00753311737622712,-0.00341159348289976,-0.000525934153839705),
 .UNSPECIFIED.);
#1156=B_SPLINE_CURVE_WITH_KNOTS('',3,(#6323,#6324,#6325,#6326,#6327,#6328,
#6329,#6330,#6331,#6332,#6333,#6334,#6335,#6336,#6337,#6338,#6339,#6340,
#6341,#6342,#6343,#6344,#6345,#6346,#6347,#6348,#6349,#6350,#6351,#6352,
#6353,#6354,#6355,#6356,#6357,#6358,#6359,#6360,#6361,#6362,#6363,#6364,
#6365,#6366,#6367,#6368,#6369,#6370,#6371),.UNSPECIFIED.,.F.,.F.,(4,3,3,
3,3,3,3,3,3,3,3,3,3,3,3,3,4),(39.2426799043403,39.347317920798,39.4553587897862,
39.5666280192012,39.6743719212775,39.7820499685097,39.8897009618222,39.9973636575694,
40.1051459330372,40.2130005998416,40.3210371210927,40.3455126251065,40.4593059977434,
40.5727552393315,40.6859938246744,40.798974097679,40.8407044963078),
 .UNSPECIFIED.);
#1157=B_SPLINE_CURVE_WITH_KNOTS('',3,(#6372,#6373,#6374,#6375,#6376,#6377,
#6378,#6379,#6380,#6381,#6382,#6383,#6384,#6385,#6386,#6387,#6388,#6389,
#6390,#6391,#6392,#6393,#6394,#6395,#6396,#6397,#6398,#6399,#6400,#6401,
#6402,#6403,#6404,#6405,#6406,#6407,#6408,#6409,#6410,#6411,#6412,#6413,
#6414,#6415,#6416,#6417,#6418,#6419,#6420,#6421,#6422,#6423,#6424,#6425,
#6426,#6427,#6428,#6429,#6430,#6431,#6432,#6433,#6434,#6435,#6436,#6437,
#6438,#6439,#6440,#6441,#6442,#6443,#6444,#6445,#6446,#6447,#6448,#6449,
#6450,#6451,#6452,#6453,#6454,#6455,#6456,#6457,#6458,#6459,#6460,#6461,
#6462,#6463,#6464,#6465,#6466,#6467,#6468,#6469,#6470,#6471,#6472,#6473,
#6474,#6475,#6476,#6477,#6478,#6479,#6480,#6481,#6482,#6483,#6484,#6485,
#6486,#6487,#6488,#6489,#6490,#6491,#6492,#6493,#6494,#6495,#6496,#6497,
#6498,#6499,#6500,#6501,#6502,#6503,#6504,#6505,#6506,#6507,#6508,#6509,
#6510,#6511,#6512,#6513,#6514,#6515,#6516,#6517,#6518,#6519,#6520,#6521,
#6522,#6523,#6524,#6525,#6526,#6527,#6528,#6529,#6530,#6531,#6532,#6533,
#6534,#6535,#6536,#6537,#6538,#6539,#6540,#6541,#6542,#6543,#6544,#6545,
#6546,#6547,#6548,#6549,#6550,#6551,#6552,#6553,#6554,#6555,#6556,#6557),
 .UNSPECIFIED.,.F.,.F.,(4,2,2,2,2,2,2,2,2,2,2,2,2,2,2,2,2,2,2,2,2,2,2,2,
2,2,2,2,2,2,2,2,2,2,2,2,2,2,2,2,2,2,2,2,2,2,2,2,2,2,2,2,2,2,2,2,2,2,2,2,
2,2,2,2,2,2,2,2,2,2,2,2,2,2,2,2,2,2,2,2,2,2,2,2,2,2,2,2,2,2,2,2,4),(-1.40437359183403,
-1.37123442544774,-1.34752963779357,-1.33956894550668,-1.33384453706723,
-1.33114265739486,-1.32902037709875,-1.32639236697421,-1.32105767193388,
-1.28990184687834,-1.27710833130175,-1.26053819930053,-1.24907775154556,
-1.24405147443566,-1.24024940402294,-1.23611045005564,-1.22933132030553,
-1.1991424444891,-1.17718888992443,-1.16481053221377,-1.15695984650571,
-1.15390650964041,-1.15174763436364,-1.14934515565329,-1.14511413330171,
-1.1199654897537,-1.07619341358872,-1.06892966170554,-1.06464923613406,
-1.0612555821067,-1.05667875748375,-1.04774607909163,-1.0360187374714,-1.00243054455778,
-0.981420876710011,-0.977242959541184,-0.974851927051027,-0.972688952611354,
-0.969609890907095,-0.96158130833031,-0.948791070416998,-0.911037219829708,
-0.895295885708175,-0.889507924932764,-0.88596636520286,-0.882113005965861,
-0.876761106568744,-0.863143851728035,-0.841650542388842,-0.80749697430888,
-0.800992055473671,-0.798368262274408,-0.796220606248343,-0.793852062063708,
-0.789778743192625,-0.769603171631479,-0.724976386629526,-0.714953988896045,
-0.710174271931691,-0.706401887754161,-0.702133000275573,-0.694731715330455,
-0.662688812809577,-0.627098897825888,-0.622213482154788,-0.619643997664196,
-0.617538915753009,-0.614779745974369,-0.608740756103967,-0.600182111874869,
-0.572873372681339,-0.544179070275189,-0.536835062276827,-0.532162650611676,
-0.528398714254533,-0.524056114345843,-0.5162990981695,-0.490744904305246,
-0.451146436953167,-0.445598441642736,-0.44288337641325,-0.44071350468291,
-0.438389667197007,-0.434523083461308,-0.418400108311522,-0.366386013304921,
-0.358997698073502,-0.354312637345431,-0.350548095703286,-0.346215342549465,
-0.338505260339425,-0.310188566919195,-0.285073042962578),.UNSPECIFIED.);
#1158=B_SPLINE_CURVE_WITH_KNOTS('',3,(#6562,#6563,#6564,#6565,#6566,#6567,
#6568,#6569,#6570,#6571,#6572,#6573,#6574,#6575,#6576,#6577,#6578,#6579,
#6580,#6581,#6582,#6583,#6584,#6585,#6586,#6587,#6588,#6589,#6590,#6591,
#6592,#6593,#6594,#6595,#6596,#6597,#6598,#6599,#6600,#6601,#6602,#6603,
#6604,#6605,#6606,#6607,#6608,#6609,#6610,#6611,#6612,#6613,#6614,#6615,
#6616,#6617,#6618,#6619,#6620,#6621,#6622,#6623,#6624,#6625,#6626,#6627,
#6628,#6629,#6630,#6631,#6632,#6633,#6634,#6635,#6636,#6637,#6638,#6639,
#6640,#6641,#6642,#6643,#6644,#6645,#6646,#6647,#6648,#6649,#6650,#6651,
#6652,#6653,#6654,#6655,#6656,#6657,#6658,#6659,#6660,#6661,#6662,#6663,
#6664,#6665,#6666,#6667,#6668,#6669,#6670,#6671,#6672,#6673,#6674,#6675,
#6676,#6677,#6678,#6679,#6680,#6681,#6682,#6683,#6684,#6685,#6686,#6687,
#6688,#6689,#6690,#6691,#6692,#6693,#6694,#6695,#6696,#6697,#6698,#6699,
#6700,#6701,#6702,#6703,#6704,#6705,#6706,#6707,#6708,#6709,#6710,#6711,
#6712,#6713,#6714,#6715,#6716,#6717,#6718,#6719,#6720,#6721,#6722,#6723,
#6724,#6725,#6726,#6727,#6728,#6729,#6730,#6731,#6732,#6733,#6734,#6735,
#6736,#6737,#6738,#6739,#6740,#6741,#6742,#6743,#6744,#6745,#6746,#6747,
#6748,#6749,#6750,#6751),.UNSPECIFIED.,.F.,.F.,(4,2,2,2,2,2,2,2,2,2,2,2,
2,2,2,2,2,2,2,2,2,2,2,2,2,2,2,2,2,2,2,2,2,2,2,2,2,2,2,2,2,2,2,2,2,2,2,2,
2,2,2,2,2,2,2,2,2,2,2,2,2,2,2,2,2,2,2,2,2,2,2,2,2,2,2,2,2,2,2,2,2,2,2,2,
2,2,2,2,2,2,2,2,2,2,4),(-1.95419705041876,-1.95099509657436,-1.94335603423285,
-1.89991425942924,-1.87506559070961,-1.87085029414465,-1.86845141700778,
-1.86629169624077,-1.86323154906988,-1.85589494163826,-1.80915527702303,
-1.78941037574571,-1.78336666657204,-1.77938126023139,-1.77555177097439,
-1.77011478780303,-1.75687520202681,-1.71971687152613,-1.69894795789413,
-1.69372753446967,-1.69112204521488,-1.68899928354412,-1.6862729303428,
-1.68061920244923,-1.64560251554659,-1.62383557245409,-1.61010952998578,
-1.60474301590359,-1.60088747043224,-1.59734954579938,-1.59158053314671,
-1.57599794538798,-1.53805844930273,-1.5252395640355,-1.51719964584465,
-1.51411912755031,-1.51195609974106,-1.50956606370411,-1.50539209599044,
-1.48448455657626,-1.45085051616374,-1.43911885055448,-1.43018312798703,
-1.42560600193481,-1.42221257001728,-1.41793303258227,-1.41067227172661,
-1.36685718427406,-1.34377191808452,-1.33830282624568,-1.33564914858626,
-1.33352753047315,-1.3308533889611,-1.32527638798234,-1.28500681146791,
-1.25934693277238,-1.25157594831113,-1.24723074868244,-1.24346741272986,
-1.23879943896024,-1.2314698664428,-1.1962869213581,-1.17389058740369,-1.16617028239694,
-1.16057494815006,-1.15789737507523,-1.15577576095328,-1.15312549402477,
-1.14767412692595,-1.11976092188052,-1.08198674324006,-1.07476016775468,
-1.07012217598063,-1.06636070172582,-1.06199273348142,-1.05411036107367,
-1.02761652170471,-1.00975943176876,-0.986126109116485,-0.981905770012072,
-0.979505779977728,-0.977346392827614,-0.974288562634894,-0.966405257133201,
-0.953952236184314,-0.930399287942635,-0.901801161853786,-0.89511851665121,
-0.891000170280617,-0.887191963350469,-0.882119951237423,-0.870373676231296,
-0.853196610132522,-0.841453580091553,-0.835099924428374),.UNSPECIFIED.);
#1159=B_SPLINE_CURVE_WITH_KNOTS('',3,(#6753,#6754,#6755,#6756,#6757,#6758,
#6759,#6760,#6761,#6762,#6763,#6764,#6765,#6766,#6767,#6768,#6769,#6770,
#6771,#6772,#6773,#6774,#6775,#6776,#6777,#6778,#6779,#6780,#6781,#6782,
#6783,#6784,#6785,#6786,#6787,#6788,#6789,#6790,#6791,#6792,#6793,#6794,
#6795,#6796,#6797,#6798,#6799,#6800,#6801,#6802,#6803,#6804,#6805,#6806,
#6807,#6808),.UNSPECIFIED.,.F.,.F.,(4,2,2,2,2,2,2,2,2,2,2,2,2,2,2,2,2,2,
2,2,2,2,2,2,2,2,2,4),(-0.285073042962578,-0.279553666108781,-0.268860677228453,
-0.265344191924806,-0.263318928126342,-0.261115262971523,-0.257812524684666,
-0.248081258600964,-0.230913628765321,-0.187069317157601,-0.179816393831322,
-0.175538464730903,-0.172144677675042,-0.167564926100631,-0.1586163724922,
-0.1468608393431,-0.113089336365138,-0.0923072130143463,-0.0881367138826751,
-0.0857473423440587,-0.0835838714087559,-0.0805013269290881,-0.072447874665844,
-0.0595990213919607,-0.0169573151041265,-0.00623282049412229,-0.002812104231931,
-0.000526075114705878),.UNSPECIFIED.);
#1160=B_SPLINE_CURVE_WITH_KNOTS('',3,(#6809,#6810,#6811,#6812,#6813,#6814,
#6815,#6816,#6817,#6818,#6819,#6820,#6821,#6822,#6823,#6824,#6825,#6826,
#6827,#6828,#6829,#6830,#6831,#6832,#6833,#6834,#6835,#6836,#6837,#6838,
#6839,#6840,#6841,#6842,#6843,#6844,#6845,#6846,#6847,#6848,#6849,#6850,
#6851,#6852,#6853,#6854,#6855,#6856,#6857,#6858,#6859,#6860,#6861,#6862,
#6863,#6864,#6865,#6866,#6867,#6868,#6869,#6870,#6871,#6872,#6873,#6874,
#6875,#6876,#6877,#6878,#6879,#6880,#6881,#6882,#6883,#6884,#6885,#6886,
#6887,#6888,#6889,#6890,#6891,#6892,#6893,#6894,#6895,#6896,#6897,#6898,
#6899,#6900,#6901,#6902,#6903,#6904,#6905,#6906,#6907,#6908,#6909,#6910,
#6911,#6912,#6913,#6914,#6915,#6916,#6917,#6918,#6919,#6920,#6921,#6922,
#6923,#6924,#6925,#6926,#6927,#6928,#6929,#6930,#6931,#6932,#6933,#6934,
#6935,#6936,#6937,#6938,#6939,#6940,#6941,#6942,#6943,#6944,#6945,#6946,
#6947,#6948,#6949,#6950,#6951,#6952,#6953,#6954,#6955,#6956),
 .UNSPECIFIED.,.F.,.F.,(4,2,2,2,2,2,2,2,2,2,2,2,2,2,2,2,2,2,2,2,2,2,2,2,
2,2,2,2,2,2,2,2,2,2,2,2,2,2,2,2,2,2,2,2,2,2,2,2,2,2,2,2,2,2,2,2,2,2,2,2,
2,2,2,2,2,2,2,2,2,2,2,2,2,4),(-2.23857561374812,-2.23666385583856,-2.2340934120843,
-2.23009258721063,-2.22419325848768,-2.20619608151607,-2.19090605687411,
-2.17043683124224,-2.15225191817315,-2.14826971816482,-2.14592139942912,
-2.14376573100267,-2.14110559550224,-2.13449203871347,-2.09568856819996,
-2.07029326499371,-2.06255934505371,-2.05822247095775,-2.05445947610837,
-2.04978301278047,-2.04242188441953,-2.00865447681867,-1.98525790756218,
-1.97735400463938,-1.97166046700269,-1.96896494610926,-1.96684359883701,
-1.96421168899267,-1.95885368261893,-1.92912983707482,-1.89155161913244,
-1.88436917889393,-1.8801467846608,-1.87636772192449,-1.87151344137471,
-1.86352917809948,-1.81252018407983,-1.79646904009444,-1.7926075584725,
-1.79028526412203,-1.78811549736986,-1.78539927151285,-1.77844064281174,
-1.74003635299827,-1.71471290957797,-1.70698834410922,-1.70265308793857,
-1.69888948105043,-1.6942096348079,-1.68683780154111,-1.65393798808469,
-1.62989527272789,-1.62187564888924,-1.61612027753882,-1.6134131074963,
-1.61129123618027,-1.60866939319371,-1.60336428715806,-1.57241511393776,
-1.54749150698952,-1.53258949837975,-1.52706691580707,-1.52318358899077,
-1.51967589277267,-1.51497195103688,-1.50319238607423,-1.46462085528223,
-1.44336862512482,-1.43809465985453,-1.43547879772472,-1.43356863123409,
-1.43096621393663,-1.42576103694743,-1.40411156028844),.UNSPECIFIED.);
#1161=B_SPLINE_CURVE_WITH_KNOTS('',3,(#6962,#6963,#6964,#6965,#6966,#6967,
#6968,#6969,#6970,#6971,#6972,#6973,#6974,#6975,#6976,#6977,#6978,#6979,
#6980,#6981,#6982,#6983,#6984,#6985,#6986,#6987,#6988,#6989,#6990,#6991,
#6992,#6993,#6994,#6995,#6996,#6997,#6998,#6999,#7000,#7001,#7002,#7003,
#7004,#7005,#7006,#7007,#7008,#7009,#7010,#7011,#7012,#7013,#7014,#7015,
#7016,#7017,#7018,#7019,#7020,#7021,#7022,#7023,#7024,#7025,#7026,#7027,
#7028,#7029,#7030,#7031,#7032,#7033,#7034,#7035,#7036,#7037,#7038,#7039,
#7040,#7041,#7042,#7043,#7044,#7045,#7046,#7047,#7048,#7049,#7050,#7051,
#7052,#7053,#7054,#7055,#7056,#7057,#7058,#7059,#7060,#7061,#7062,#7063,
#7064,#7065,#7066,#7067,#7068,#7069,#7070,#7071,#7072,#7073,#7074,#7075,
#7076,#7077,#7078,#7079,#7080,#7081,#7082,#7083,#7084,#7085,#7086,#7087,
#7088,#7089,#7090,#7091,#7092,#7093,#7094,#7095,#7096,#7097),
 .UNSPECIFIED.,.F.,.F.,(4,2,2,2,2,2,2,2,2,2,2,2,2,2,2,2,2,2,2,2,2,2,2,2,
2,2,2,2,2,2,2,2,2,2,2,2,2,2,2,2,2,2,2,2,2,2,2,2,2,2,2,2,2,2,2,2,2,2,2,2,
2,2,2,2,2,2,2,4),(-0.83510473565426,-0.807059091250157,-0.794248944238828,
-0.788888281898605,-0.785072276945066,-0.781065979555653,-0.774919202696639,
-0.753969699442934,-0.731087482698737,-0.705729883148012,-0.700270175960026,
-0.697618575084768,-0.69549732017242,-0.692822002462581,-0.687237232275534,
-0.679536961050213,-0.657240309233987,-0.621967947033965,-0.614643791100851,
-0.609977772140206,-0.606215108268336,-0.601869681911633,-0.594095560427073,
-0.568407118507129,-0.527431822374366,-0.522306693016003,-0.519720011857097,
-0.517809058982425,-0.515176404745292,-0.509816001002867,-0.487766096186353,
-0.446763188010461,-0.437032466896656,-0.43230609171582,-0.428538863753342,
-0.424236117433176,-0.41666977793013,-0.385854931560725,-0.351305194221669,
-0.345096691777328,-0.34233722111936,-0.340209517527547,-0.337667515641714,
-0.332765712758342,-0.303531750266518,-0.266259382527087,-0.259006079374804,
-0.254360551254719,-0.250598995790071,-0.246237674293427,-0.238386499891509,
-0.212124957649786,-0.172168692303313,-0.166846565800831,-0.164221259453316,
-0.162099263379596,-0.15939533519259,-0.153658354972325,-0.145674488158747,
-0.121830870754642,-0.0886967464382455,-0.0813294240915939,-0.0766505948237803,
-0.0728866835996491,-0.0685498339497959,-0.0608190313853347,-0.0354526272559785,
-0.000526495403762602),.UNSPECIFIED.);
#1162=B_SPLINE_CURVE_WITH_KNOTS('',3,(#7098,#7099,#7100,#7101,#7102,#7103,
#7104,#7105,#7106,#7107,#7108,#7109,#7110,#7111,#7112,#7113,#7114,#7115,
#7116,#7117,#7118,#7119,#7120,#7121,#7122,#7123,#7124,#7125,#7126,#7127,
#7128,#7129,#7130,#7131,#7132,#7133,#7134,#7135,#7136,#7137,#7138,#7139,
#7140,#7141,#7142,#7143,#7144,#7145,#7146,#7147,#7148,#7149,#7150,#7151,
#7152,#7153),.UNSPECIFIED.,.F.,.F.,(4,2,2,2,2,2,2,2,2,2,2,2,2,2,2,2,2,2,
2,2,2,2,2,2,2,2,2,4),(-2.23859886574399,-2.23016997570174,-2.22724347696598,
-2.22509778038061,-2.22304729674188,-2.22064081803864,-2.21638940119625,
-2.19887690410067,-2.16438742506128,-2.1449527001157,-2.13893733858008,
-2.13495785335683,-2.13112475931472,-2.12652164794244,-2.11536814953201,
-2.07614378249324,-2.05467230085902,-2.04937433483211,-2.0467537992826,
-2.04484343810543,-2.04224546994443,-2.03722372250726,-2.00306363251165,
-1.97305660076362,-1.96376339585746,-1.95911833261462,-1.95535679587401,
-1.95419705041876),.UNSPECIFIED.);
#1163=B_SPLINE_CURVE_WITH_KNOTS('',3,(#7154,#7155,#7156,#7157,#7158,#7159,
#7160,#7161,#7162,#7163,#7164,#7165,#7166,#7167,#7168,#7169,#7170,#7171,
#7172,#7173,#7174,#7175,#7176,#7177,#7178,#7179,#7180,#7181,#7182,#7183,
#7184,#7185,#7186,#7187,#7188,#7189,#7190,#7191,#7192,#7193,#7194,#7195,
#7196,#7197,#7198,#7199,#7200,#7201,#7202,#7203,#7204,#7205,#7206,#7207,
#7208,#7209,#7210,#7211,#7212,#7213,#7214,#7215,#7216,#7217,#7218,#7219,
#7220,#7221,#7222,#7223,#7224,#7225,#7226,#7227,#7228,#7229,#7230,#7231,
#7232,#7233,#7234,#7235,#7236,#7237,#7238,#7239,#7240,#7241,#7242,#7243,
#7244,#7245,#7246,#7247,#7248,#7249,#7250,#7251,#7252,#7253,#7254,#7255,
#7256,#7257,#7258,#7259,#7260,#7261,#7262,#7263,#7264,#7265,#7266,#7267,
#7268,#7269,#7270,#7271,#7272,#7273,#7274,#7275,#7276,#7277,#7278,#7279,
#7280,#7281,#7282,#7283,#7284,#7285,#7286,#7287,#7288,#7289,#7290,#7291,
#7292,#7293,#7294,#7295,#7296,#7297,#7298,#7299,#7300,#7301,#7302,#7303,
#7304,#7305,#7306,#7307,#7308,#7309,#7310,#7311,#7312,#7313,#7314,#7315,
#7316,#7317,#7318,#7319,#7320,#7321,#7322,#7323,#7324,#7325,#7326,#7327,
#7328,#7329,#7330,#7331,#7332,#7333,#7334,#7335,#7336,#7337,#7338,#7339,
#7340,#7341,#7342,#7343),.UNSPECIFIED.,.F.,.F.,(4,2,2,2,2,2,2,2,2,2,2,2,
2,2,2,2,2,2,2,2,2,2,2,2,2,2,2,2,2,2,2,2,2,2,2,2,2,2,2,2,2,2,2,2,2,2,2,2,
2,2,2,2,2,2,2,2,2,2,2,2,2,2,2,2,2,2,2,2,2,2,2,2,2,2,2,2,2,2,2,2,2,2,2,2,
2,2,2,2,2,2,2,2,2,2,4),(-1.40411156028844,-1.39349542557748,-1.36935987545478,
-1.35473797928305,-1.34925131297417,-1.34537445729729,-1.34186020981609,
-1.33712872630781,-1.32517580104704,-1.28678083561332,-1.27108739193897,
-1.26481221899932,-1.26002549128862,-1.25750686692788,-1.25537609341367,
-1.25258406971052,-1.24618619485546,-1.20692794327319,-1.18144655746937,
-1.17370009162669,-1.16936012333648,-1.16559662849119,-1.16092238061841,
-1.15357054764298,-1.11942673560362,-1.08784664187256,-1.08254616461267,
-1.07992503533727,-1.07780287823297,-1.07509426121558,-1.0693320686284,
-1.06130086376561,-1.03718984474042,-1.00441413216787,-0.997041813059222,
-0.992361495680813,-0.988597433613231,-0.984261566797749,-0.976535753034919,
-0.951206572032963,-0.912829974784523,-0.905819434608511,-0.903095179753961,
-0.900923137884646,-0.898603804428527,-0.894757087456774,-0.878940018869739,
-0.83075013623136,-0.819907281922897,-0.815037208524472,-0.811245612843338,
-0.807073897687486,-0.800135930020867,-0.764276356933327,-0.732100216115735,
-0.726880331832764,-0.724274918542289,-0.722364713349845,-0.719751555505083,
-0.714492055170275,-0.693372844261857,-0.655183432209298,-0.64304735200466,
-0.638290363807922,-0.634769988408522,-0.630898851688508,-0.625444407383234,
-0.611070142823161,-0.587610459950588,-0.554188019843694,-0.549050425734941,
-0.546461192345198,-0.544550262122613,-0.541920076882484,-0.536572921944452,
-0.514648747427636,-0.474039109303757,-0.464077047169949,-0.4592416762617,
-0.455463939474107,-0.451229172488678,-0.443990541578409,-0.435104383296082,
-0.415083011447363,-0.384841681837122,-0.373635655274898,-0.370061264147062,
-0.367801128323677,-0.365558213430779,-0.362064012666355,-0.350585761782471,
-0.327888579904079,-0.293170013073975,-0.285831970878823,-0.285021347106446),
 .UNSPECIFIED.);
#1164=B_SPLINE_CURVE_WITH_KNOTS('',3,(#7348,#7349,#7350,#7351,#7352,#7353,
#7354,#7355,#7356,#7357,#7358,#7359,#7360,#7361,#7362,#7363,#7364,#7365,
#7366,#7367,#7368,#7369,#7370,#7371,#7372,#7373,#7374,#7375,#7376,#7377,
#7378,#7379,#7380,#7381,#7382,#7383,#7384,#7385,#7386,#7387,#7388,#7389,
#7390,#7391,#7392,#7393,#7394,#7395,#7396,#7397,#7398,#7399,#7400,#7401,
#7402,#7403,#7404,#7405,#7406,#7407,#7408,#7409,#7410,#7411,#7412,#7413,
#7414,#7415,#7416,#7417,#7418,#7419,#7420,#7421,#7422,#7423,#7424,#7425,
#7426,#7427,#7428,#7429,#7430,#7431,#7432,#7433,#7434,#7435,#7436,#7437,
#7438,#7439,#7440,#7441,#7442,#7443,#7444,#7445,#7446,#7447,#7448,#7449,
#7450,#7451,#7452,#7453,#7454,#7455,#7456,#7457,#7458,#7459,#7460,#7461,
#7462,#7463,#7464,#7465,#7466,#7467,#7468,#7469,#7470,#7471,#7472,#7473,
#7474,#7475,#7476,#7477,#7478,#7479,#7480,#7481,#7482,#7483,#7484,#7485,
#7486,#7487,#7488,#7489,#7490,#7491,#7492,#7493,#7494,#7495,#7496,#7497,
#7498,#7499,#7500,#7501,#7502,#7503,#7504,#7505,#7506,#7507,#7508,#7509,
#7510,#7511,#7512,#7513,#7514,#7515,#7516,#7517,#7518,#7519,#7520,#7521,
#7522,#7523,#7524,#7525,#7526,#7527,#7528,#7529,#7530,#7531,#7532,#7533,
#7534,#7535,#7536,#7537,#7538,#7539,#7540,#7541,#7542,#7543,#7544,#7545,
#7546,#7547),.UNSPECIFIED.,.F.,.F.,(4,2,2,2,2,2,2,2,2,2,2,2,2,2,2,2,2,2,
2,2,2,2,2,2,2,2,2,2,2,2,2,2,2,2,2,2,2,2,2,2,2,2,2,2,2,2,2,2,2,2,2,2,2,2,
2,2,2,2,2,2,2,2,2,2,2,2,2,2,2,2,2,2,2,2,2,2,2,2,2,2,2,2,2,2,2,2,2,2,2,2,
2,2,2,2,2,2,2,2,2,4),(-1.95389506130437,-1.94961407086964,-1.94435265691815,
-1.9417394763262,-1.93982967560218,-1.93722540144905,-1.93217238412767,
-1.89841999475128,-1.88910996699134,-1.87181659205363,-1.86001599820056,
-1.85493622470532,-1.8511276740487,-1.84701417635579,-1.84035134606648,
-1.81268413208584,-1.78850716862925,-1.77582103745545,-1.76783848349445,
-1.76476668612379,-1.76260547966791,-1.76021256979286,-1.75602354976164,
-1.73457015197743,-1.70139011953736,-1.68973132370297,-1.68083751565559,
-1.67626915432287,-1.67287722664734,-1.66859303510394,-1.66130810579235,
-1.61768751473044,-1.6003961500096,-1.59062264733991,-1.5873153830201,-1.58511126646256,
-1.58308774125901,-1.57957835825508,-1.5689401084213,-1.53829815592585,
-1.50969215678852,-1.50214984669414,-1.49785244116081,-1.49408511785598,
-1.48935228332671,-1.47958438212244,-1.43860450025514,-1.4165581110702,
-1.41119840668634,-1.4085660720675,-1.40665535200453,-1.40406895956547,
-1.39894437893211,-1.35800115287627,-1.33232428381637,-1.32455198038943,
-1.32020713893897,-1.31644471811796,-1.31177866222187,-1.30445369728431,
-1.26915912477824,-1.24685262501099,-1.23915004915792,-1.23356460720518,
-1.23088926696933,-1.22876815160177,-1.22611691801824,-1.22065857037651,
-1.19528125124984,-1.17267928575953,-1.15154607074122,-1.14538494328039,
-1.14137584354151,-1.13756178738194,-1.13221168315488,-1.11948299799636,
-1.0995854202924,-1.0696506914718,-1.05804258353884,-1.05442601881422,-1.05215697126489,
-1.04992271780096,-1.04646843229878,-1.03537755616004,-1.01401815355054,
-0.977397958580947,-0.970116091790745,-0.965462467500581,-0.961700727744027,
-0.957346288875495,-0.949527612400665,-0.923506871345019,-0.883134127625715,
-0.87789155775808,-0.875281862505312,-0.873372002991157,-0.870763717472937,
-0.865528363713152,-0.84462382045794,-0.83510473565426),.UNSPECIFIED.);
#1165=B_SPLINE_CURVE_WITH_KNOTS('',3,(#7549,#7550,#7551,#7552,#7553,#7554,
#7555,#7556,#7557,#7558,#7559,#7560,#7561,#7562,#7563,#7564,#7565,#7566,
#7567,#7568,#7569,#7570,#7571,#7572,#7573,#7574,#7575,#7576,#7577,#7578,
#7579,#7580,#7581,#7582,#7583,#7584,#7585,#7586,#7587,#7588,#7589,#7590,
#7591,#7592,#7593,#7594,#7595,#7596,#7597,#7598,#7599,#7600,#7601,#7602,
#7603,#7604),.UNSPECIFIED.,.F.,.F.,(4,2,2,2,2,2,2,2,2,2,2,2,2,2,2,2,2,2,
2,2,2,2,2,2,2,2,2,4),(-0.285021347106446,-0.281161663193334,-0.277398373222973,
-0.273055360378498,-0.26529436340703,-0.239706237843135,-0.199900284683521,
-0.193933541577183,-0.191187489861275,-0.189063723903572,-0.186474581453647,
-0.181337663102854,-0.161304723832711,-0.115050076035869,-0.107866320922798,
-0.103240961868744,-0.0994803599945839,-0.0951028654889191,-0.0871730377536201,
-0.0603159778932275,-0.0331866955665843,-0.018623391917416,-0.0147530662472885,
-0.0124287244048125,-0.0104203730523619,-0.00822868690897723,-0.00481396187852919,
-0.000525490636961181),.UNSPECIFIED.);
#1166=B_SPLINE_CURVE_WITH_KNOTS('',3,(#7605,#7606,#7607,#7608,#7609,#7610,
#7611,#7612,#7613,#7614,#7615,#7616,#7617,#7618,#7619,#7620,#7621,#7622,
#7623,#7624,#7625,#7626,#7627,#7628,#7629,#7630,#7631,#7632,#7633,#7634,
#7635,#7636,#7637,#7638,#7639,#7640,#7641,#7642,#7643,#7644,#7645,#7646,
#7647,#7648,#7649,#7650,#7651,#7652,#7653,#7654,#7655,#7656,#7657,#7658,
#7659,#7660,#7661,#7662,#7663,#7664,#7665,#7666,#7667,#7668,#7669,#7670,
#7671,#7672,#7673,#7674,#7675,#7676,#7677,#7678,#7679,#7680,#7681,#7682,
#7683,#7684,#7685,#7686,#7687,#7688,#7689,#7690,#7691,#7692,#7693,#7694,
#7695,#7696,#7697,#7698,#7699,#7700,#7701,#7702,#7703,#7704,#7705,#7706,
#7707,#7708,#7709,#7710,#7711,#7712,#7713,#7714,#7715,#7716,#7717,#7718,
#7719,#7720,#7721,#7722,#7723,#7724,#7725,#7726,#7727,#7728,#7729,#7730,
#7731,#7732,#7733,#7734,#7735,#7736,#7737,#7738,#7739,#7740,#7741,#7742,
#7743,#7744),.UNSPECIFIED.,.F.,.F.,(4,2,2,2,2,2,2,2,2,2,2,2,2,2,2,2,2,2,
2,2,2,2,2,2,2,2,2,2,2,2,2,2,2,2,2,2,2,2,2,2,2,2,2,2,2,2,2,2,2,2,2,2,2,2,
2,2,2,2,2,2,2,2,2,2,2,2,2,2,2,4),(-2.23873337236619,-2.20260153586138,-2.18290354736451,
-2.17410529702119,-2.16692151586359,-2.16269877503993,-2.15891966849369,
-2.15406570341143,-2.14361974126213,-2.10338553776005,-2.08158050601579,
-2.07624669828436,-2.07361939563287,-2.07170894832296,-2.0691179794163,
-2.06397009729765,-2.03082745801115,-2.00722841399602,-1.99280304483619,
-1.98734252780382,-1.98347075456529,-1.97995221815648,-1.97520141296699,
-1.96311026933505,-1.92485882536148,-1.90920460026644,-1.90293934496288,
-1.89815850660555,-1.89564126320214,-1.89351057571928,-1.89071729755099,
-1.88431088936225,-1.84997724502122,-1.81924544384307,-1.81169873693335,
-1.80740023942076,-1.80363277032895,-1.79890083745404,-1.78913895509525,
-1.7481469466383,-1.72609562974091,-1.72073516954654,-1.71810258222976,
-1.71619173394012,-1.71360526029047,-1.70848079994277,-1.66753023018797,
-1.64185225415164,-1.63407947481888,-1.62973435244094,-1.62597168549879,
-1.62130532605614,-1.61397990297146,-1.5786737489019,-1.55637030653304,
-1.54866800941179,-1.54308260875925,-1.54040716761905,-1.53828591523418,
-1.53563445127925,-1.53017546094156,-1.50476967412082,-1.48213862790443,
-1.46805288800406,-1.45783577156451,-1.45302172687808,-1.44924644613653,
-1.44499963097781,-1.437702390342,-1.40420841399148),.UNSPECIFIED.);
#1167=B_SPLINE_CURVE_WITH_KNOTS('',3,(#7750,#7751,#7752,#7753,#7754,#7755,
#7756,#7757,#7758,#7759,#7760,#7761,#7762,#7763,#7764,#7765,#7766,#7767,
#7768,#7769,#7770,#7771,#7772,#7773,#7774,#7775,#7776,#7777,#7778,#7779,
#7780,#7781,#7782,#7783,#7784,#7785,#7786,#7787,#7788,#7789,#7790,#7791,
#7792,#7793,#7794,#7795,#7796,#7797,#7798,#7799,#7800,#7801,#7802,#7803,
#7804,#7805,#7806,#7807,#7808,#7809,#7810,#7811,#7812,#7813,#7814,#7815,
#7816,#7817,#7818,#7819,#7820,#7821,#7822,#7823,#7824,#7825,#7826,#7827,
#7828,#7829,#7830,#7831,#7832,#7833,#7834,#7835,#7836,#7837,#7838,#7839,
#7840,#7841,#7842,#7843,#7844,#7845,#7846,#7847,#7848,#7849,#7850,#7851,
#7852,#7853,#7854,#7855,#7856,#7857,#7858,#7859,#7860,#7861,#7862,#7863,
#7864,#7865,#7866,#7867,#7868,#7869,#7870,#7871,#7872,#7873,#7874,#7875,
#7876,#7877,#7878,#7879,#7880,#7881,#7882,#7883,#7884,#7885,#7886,#7887,
#7888,#7889,#7890,#7891),.UNSPECIFIED.,.F.,.F.,(4,2,2,2,2,2,2,2,2,2,2,2,
2,2,2,2,2,2,2,2,2,2,2,2,2,2,2,2,2,2,2,2,2,2,2,2,2,2,2,2,2,2,2,2,2,2,2,2,
2,2,2,2,2,2,2,2,2,2,2,2,2,2,2,2,2,2,2,2,2,2,4),(-0.834941232871745,-0.819338014613434,
-0.780419456840186,-0.773876897628689,-0.771228350000444,-0.769075182262562,
-0.76672028489106,-0.762709008813453,-0.743935227528527,-0.719696160537062,
-0.692151444314202,-0.685491273255296,-0.681377889244008,-0.677568419768757,
-0.672485879720932,-0.660671654104035,-0.643348347957285,-0.634390608508764,
-0.600233948948421,-0.595207024521789,-0.592607904272523,-0.590697485827355,
-0.588077895921618,-0.582785190975061,-0.561363093112121,-0.522274883487837,
-0.511014445225283,-0.506393652155711,-0.502556064184696,-0.49858242784488,
-0.492596844588132,-0.473488659060427,-0.431526252182873,-0.41984652524168,
-0.416222493416279,-0.413951549150567,-0.411718154216969,-0.408269305484565,
-0.397234586843687,-0.376066447351619,-0.339149533468926,-0.331878451887984,
-0.327227489186553,-0.323465256407915,-0.319107300980184,-0.311273966591775,
-0.285149694537114,-0.244944364750276,-0.239667356677667,-0.237050648384628,
-0.234928128784792,-0.23221401927413,-0.226422854751299,-0.218337265924506,
-0.193916179048666,-0.161693698825526,-0.154241741883327,-0.149538166080894,
-0.145772111928063,-0.14169416235255,-0.134597951492617,-0.125762832492979,
-0.105932740980304,-0.0761709353257024,-0.0643122292258017,-0.0606708060663044,
-0.0583959850014676,-0.056165596692382,-0.0527316363869023,-0.041839504113066,
-0.000526393493502488),.UNSPECIFIED.);
#1168=B_SPLINE_CURVE_WITH_KNOTS('',3,(#7892,#7893,#7894,#7895,#7896,#7897,
#7898,#7899,#7900,#7901,#7902,#7903,#7904,#7905,#7906,#7907,#7908,#7909,
#7910,#7911,#7912,#7913,#7914,#7915,#7916,#7917,#7918,#7919,#7920,#7921,
#7922,#7923,#7924,#7925,#7926,#7927,#7928,#7929,#7930,#7931,#7932,#7933,
#7934,#7935,#7936,#7937,#7938,#7939,#7940,#7941),.UNSPECIFIED.,.F.,.F.,
(4,2,2,2,2,2,2,2,2,2,2,2,2,2,2,2,2,2,2,2,2,2,2,2,4),(-2.23848733616259,
-2.22485318200342,-2.21633320517607,-2.21215613460426,-2.20862493584771,
-2.20485000070879,-2.20003279176477,-2.19217956066984,-2.16197540421594,
-2.12745580410469,-2.12212413723587,-2.11949737154508,-2.11758708314289,
-2.11499597865043,-2.10984679614268,-2.07674844291394,-2.05312696383485,
-2.03869388648012,-2.03323263556511,-2.02936094762936,-2.02584288805889,
-2.02109333083917,-2.00900968516074,-1.97075663324338,-1.95389506130437),
 .UNSPECIFIED.);
#1169=B_SPLINE_CURVE_WITH_KNOTS('',3,(#7942,#7943,#7944,#7945,#7946,#7947,
#7948,#7949,#7950,#7951,#7952,#7953,#7954,#7955,#7956,#7957,#7958,#7959,
#7960,#7961,#7962,#7963,#7964,#7965,#7966,#7967,#7968,#7969,#7970,#7971,
#7972,#7973,#7974,#7975,#7976,#7977,#7978,#7979,#7980,#7981,#7982,#7983,
#7984,#7985,#7986,#7987,#7988,#7989,#7990,#7991,#7992,#7993,#7994,#7995,
#7996,#7997,#7998,#7999,#8000,#8001,#8002,#8003,#8004,#8005,#8006,#8007,
#8008,#8009,#8010,#8011,#8012,#8013,#8014,#8015,#8016,#8017,#8018,#8019,
#8020,#8021,#8022,#8023,#8024,#8025,#8026,#8027,#8028,#8029,#8030,#8031,
#8032,#8033,#8034,#8035,#8036,#8037,#8038,#8039,#8040,#8041,#8042,#8043,
#8044,#8045,#8046,#8047,#8048,#8049,#8050,#8051,#8052,#8053,#8054,#8055,
#8056,#8057,#8058,#8059,#8060,#8061,#8062,#8063,#8064,#8065,#8066,#8067,
#8068,#8069,#8070,#8071,#8072,#8073,#8074,#8075,#8076,#8077,#8078,#8079,
#8080,#8081,#8082,#8083,#8084,#8085,#8086,#8087,#8088,#8089,#8090,#8091,
#8092,#8093,#8094,#8095,#8096,#8097,#8098,#8099,#8100,#8101,#8102,#8103,
#8104,#8105,#8106,#8107,#8108,#8109,#8110,#8111,#8112,#8113,#8114,#8115,
#8116,#8117,#8118,#8119,#8120,#8121,#8122,#8123,#8124,#8125,#8126,#8127,
#8128,#8129,#8130,#8131,#8132,#8133,#8134,#8135,#8136,#8137,#8138,#8139),
 .UNSPECIFIED.,.F.,.F.,(4,2,2,2,2,2,2,2,2,2,2,2,2,2,2,2,2,2,2,2,2,2,2,2,
2,2,2,2,2,2,2,2,2,2,2,2,2,2,2,2,2,2,2,2,2,2,2,2,2,2,2,2,2,2,2,2,2,2,2,2,
2,2,2,2,2,2,2,2,2,2,2,2,2,2,2,2,2,2,2,2,2,2,2,2,2,2,2,2,2,2,2,2,2,2,2,2,
2,2,4),(-1.40420841399148,-1.39355085824773,-1.37068095745477,-1.36523429056841,
-1.36258503480482,-1.36046356537884,-1.35778535404069,-1.3521859982408,
-1.31194709694592,-1.28629339955214,-1.27852358256444,-1.27417885925728,
-1.27041584373649,-1.26574815358256,-1.25841880912706,-1.22324735169539,
-1.20084496528604,-1.19312375741313,-1.18752804544374,-1.18485054075049,
-1.18272911148411,-1.18007925110546,-1.17462928826426,-1.14659570558973,
-1.11979609484233,-1.10454601711322,-1.09881849975883,-1.09528795179867,
-1.09142627359652,-1.08602448626551,-1.07204197353568,-1.04961711990649,
-1.01439200502626,-1.00946749841059,-1.00688989526563,-1.00478570579984,
-1.00203736967785,-0.996057649487697,-0.987612828446478,-0.961027674378112,
-0.928995314272646,-0.922189678648912,-0.91804561900955,-0.914245962646039,
-0.909233395123018,-0.897854058863521,-0.881449779753469,-0.873478405681935,
-0.839723164020809,-0.832837778243438,-0.830132965077558,-0.827965937935453,
-0.825638057805196,-0.821751750741515,-0.805301727632524,-0.763004484872936,
-0.748692243702467,-0.743093060912541,-0.739584695251194,-0.735701591510242,
-0.730181270271251,-0.715299877918116,-0.690435483761497,-0.659378742363925,
-0.65405622901202,-0.651430864811441,-0.64930889866142,-0.646605118362785,
-0.640868842698541,-0.632886296918339,-0.609050309072773,-0.57590377349962,
-0.568536528569407,-0.563857748232123,-0.560093882171785,-0.555757095735888,
-0.548026454118691,-0.522661168402109,-0.484088335858775,-0.477248979051107,
-0.474551509223608,-0.472386317805916,-0.470055037896324,-0.466153132787228,
-0.449443075236179,-0.408967283228258,-0.393484502618362,-0.387727799103882,
-0.384192099958015,-0.380334802546535,-0.374958047900295,-0.361158432775706,
-0.33920333043169,-0.303099337412899,-0.298273233190325,-0.295716508079725,
-0.293590177778295,-0.290802973593218,-0.285157208614073),.UNSPECIFIED.);
#1170=B_SPLINE_CURVE_WITH_KNOTS('',3,(#8144,#8145,#8146,#8147,#8148,#8149,
#8150,#8151,#8152,#8153,#8154,#8155,#8156,#8157,#8158,#8159,#8160,#8161,
#8162,#8163,#8164,#8165,#8166,#8167,#8168,#8169,#8170,#8171,#8172,#8173,
#8174,#8175,#8176,#8177,#8178,#8179,#8180,#8181,#8182,#8183,#8184,#8185,
#8186,#8187,#8188,#8189,#8190,#8191,#8192,#8193,#8194,#8195,#8196,#8197,
#8198,#8199,#8200,#8201,#8202,#8203,#8204,#8205,#8206,#8207,#8208,#8209,
#8210,#8211,#8212,#8213,#8214,#8215,#8216,#8217,#8218,#8219,#8220,#8221,
#8222,#8223,#8224,#8225,#8226,#8227,#8228,#8229,#8230,#8231,#8232,#8233,
#8234,#8235,#8236,#8237,#8238,#8239,#8240,#8241,#8242,#8243,#8244,#8245,
#8246,#8247,#8248,#8249,#8250,#8251,#8252,#8253,#8254,#8255,#8256,#8257,
#8258,#8259,#8260,#8261,#8262,#8263,#8264,#8265,#8266,#8267,#8268,#8269,
#8270,#8271,#8272,#8273,#8274,#8275,#8276,#8277,#8278,#8279,#8280,#8281,
#8282,#8283,#8284,#8285,#8286,#8287,#8288,#8289,#8290,#8291,#8292,#8293,
#8294,#8295,#8296,#8297,#8298,#8299,#8300,#8301,#8302,#8303,#8304,#8305,
#8306,#8307,#8308,#8309,#8310,#8311,#8312,#8313,#8314,#8315,#8316,#8317,
#8318,#8319,#8320,#8321,#8322,#8323,#8324,#8325,#8326,#8327,#8328,#8329,
#8330,#8331,#8332,#8333,#8334,#8335,#8336,#8337,#8338,#8339,#8340,#8341),
 .UNSPECIFIED.,.F.,.F.,(4,2,2,2,2,2,2,2,2,2,2,2,2,2,2,2,2,2,2,2,2,2,2,2,
2,2,2,2,2,2,2,2,2,2,2,2,2,2,2,2,2,2,2,2,2,2,2,2,2,2,2,2,2,2,2,2,2,2,2,2,
2,2,2,2,2,2,2,2,2,2,2,2,2,2,2,2,2,2,2,2,2,2,2,2,2,2,2,2,2,2,2,2,2,2,2,2,
2,2,4),(-1.95382075976061,-1.93845052981756,-1.93070666029189,-1.9263675316077,
-1.92260441862345,-1.91793019017277,-1.91057744168998,-1.87653626945298,
-1.8533311845946,-1.84546181664684,-1.83978665309728,-1.83709442962286,
-1.83497298814602,-1.83233759939909,-1.82696219477251,-1.7979812412323,
-1.78360878890008,-1.76673997215926,-1.75513850476569,-1.75009033008937,
-1.74628608926052,-1.74215864511806,-1.7354304806649,-1.70570588671948,
-1.68167068743024,-1.664781094057,-1.66086882214523,-1.65853550021191,-1.65637184638938,
-1.65367981029778,-1.64687273748103,-1.60829409006462,-1.58293891903977,
-1.5752100522226,-1.57087391298388,-1.56711038473087,-1.5624317303758,-1.55506400416146,
-1.52187827217161,-1.49804835775141,-1.49006645882824,-1.4843311693325,
-1.48162771641708,-1.47950594603847,-1.47688072266254,-1.47155818798291,
-1.43163605391564,-1.40818843102222,-1.39862940882099,-1.39393482962389,
-1.39017024089405,-1.38584575380967,-1.37837749865787,-1.3361049276215,
-1.3181039628199,-1.30808392023966,-1.30474738504513,-1.30253728859641,
-1.30023722684789,-1.29647817865237,-1.28329662560233,-1.25451791384796,
-1.22774616453828,-1.21982779866319,-1.215452848043,-1.21169235392893,-1.20706448124509,
-1.1998714580494,-1.16155001968581,-1.1412710393405,-1.13050817446906,-1.12708839749912,
-1.12486126850819,-1.12285967406226,-1.11946664468586,-1.10894779060463,
-1.08944157058243,-1.04989373171123,-1.04211574409565,-1.0377242011372,
-1.03396476539228,-1.02935756144726,-1.02026350460516,-0.986049149790715,
-0.956172483798929,-0.950819091201227,-0.948187847482847,-0.946066168697338,
-0.943369124946128,-0.937668613180446,-0.92975293161244,-0.906289133856426,
-0.872640417009587,-0.865281885519018,-0.860605785529775,-0.856842305984083,
-0.85250400955929,-0.844765207762263,-0.834941232871745),.UNSPECIFIED.);
#1171=B_SPLINE_CURVE_WITH_KNOTS('',3,(#8343,#8344,#8345,#8346,#8347,#8348,
#8349,#8350,#8351,#8352,#8353,#8354,#8355,#8356,#8357,#8358,#8359,#8360,
#8361,#8362,#8363,#8364,#8365,#8366,#8367,#8368,#8369,#8370,#8371,#8372,
#8373,#8374,#8375,#8376,#8377,#8378,#8379,#8380,#8381,#8382,#8383,#8384,
#8385,#8386,#8387,#8388,#8389,#8390,#8391,#8392,#8393,#8394,#8395,#8396),
 .UNSPECIFIED.,.F.,.F.,(4,2,2,2,2,2,2,2,2,2,2,2,2,2,2,2,2,2,2,2,2,2,2,2,
2,2,4),(-0.285157208614073,-0.284605315737705,-0.275737691792264,-0.246338366236847,
-0.217633348387182,-0.210948205204423,-0.206829394393677,-0.203021468104304,
-0.197950906522848,-0.186213318125285,-0.169054758634776,-0.157029278777212,
-0.126021054712905,-0.120709481011801,-0.118086144868309,-0.11596398705953,
-0.113257637150128,-0.107508001161571,-0.0995005129755145,-0.0681711636269896,
-0.041713286785829,-0.0341178041145199,-0.0297652273629336,-0.0260024939904901,
-0.0223858321731088,-0.0178186478765722,-0.000525515565460478),
 .UNSPECIFIED.);
#1172=B_SPLINE_CURVE_WITH_KNOTS('',3,(#8397,#8398,#8399,#8400,#8401,#8402,
#8403,#8404,#8405,#8406,#8407,#8408,#8409,#8410,#8411,#8412,#8413,#8414,
#8415,#8416,#8417,#8418,#8419,#8420,#8421,#8422,#8423,#8424,#8425,#8426,
#8427,#8428,#8429,#8430,#8431,#8432,#8433,#8434,#8435,#8436,#8437,#8438,
#8439,#8440,#8441,#8442,#8443,#8444,#8445,#8446,#8447,#8448,#8449,#8450,
#8451,#8452,#8453,#8454,#8455,#8456,#8457,#8458,#8459,#8460,#8461,#8462,
#8463,#8464,#8465,#8466,#8467,#8468,#8469,#8470,#8471,#8472,#8473,#8474,
#8475,#8476,#8477,#8478,#8479,#8480,#8481,#8482,#8483,#8484,#8485,#8486,
#8487,#8488,#8489,#8490,#8491,#8492,#8493,#8494,#8495,#8496,#8497,#8498,
#8499,#8500,#8501,#8502,#8503,#8504,#8505,#8506,#8507,#8508,#8509,#8510,
#8511,#8512,#8513,#8514,#8515,#8516,#8517,#8518,#8519,#8520,#8521,#8522,
#8523,#8524,#8525,#8526,#8527,#8528,#8529,#8530,#8531,#8532,#8533,#8534,
#8535,#8536,#8537,#8538,#8539,#8540,#8541,#8542,#8543,#8544,#8545,#8546,
#8547,#8548),.UNSPECIFIED.,.F.,.F.,(4,2,2,2,2,2,2,2,2,2,2,2,2,2,2,2,2,2,
2,2,2,2,2,2,2,2,2,2,2,2,2,2,2,2,2,2,2,2,2,2,2,2,2,2,2,2,2,2,2,2,2,2,2,2,
2,2,2,2,2,2,2,2,2,2,2,2,2,2,2,2,2,2,2,2,2,4),(-2.23842674530037,-2.20180201490224,
-2.18966994179993,-2.18192756901689,-2.17889073702879,-2.1767349235105,
-2.17432599390694,-2.17006282288876,-2.14365978257604,-2.12285723952658,
-2.10716807487443,-2.09953432254986,-2.09323023706848,-2.09302700584519,
-2.09282456983365,-2.09262050856384,-2.09241219277337,-2.08866215051524,
-2.08482843299966,-2.08022266103576,-2.06905290959127,-2.02984685376578,
-2.00837808613535,-2.00308041128917,-2.00045994455024,-1.99854960340612,
-1.99595162979262,-1.99092979930649,-1.95674749436908,-1.94783644870737,
-1.93052176089478,-1.91871064319739,-1.91362873843839,-1.90981944432645,
-1.90570596167661,-1.89904502981321,-1.87151371487476,-1.84723891346056,
-1.83451667686,-1.82651825573437,-1.8234438934767,-1.82128203565596,-1.81888972428875,
-1.81470447929034,-1.79340993024457,-1.76009267369779,-1.74841109768661,
-1.7395040000213,-1.73493266790465,-1.73154005437192,-1.72725699531547,
-1.71997897385422,-1.67629271449942,-1.65902775150732,-1.64926296056025,
-1.64595642957898,-1.6437522395154,-1.64144330613434,-1.63764372435906,
-1.62428903489381,-1.58405022798349,-1.56522856919212,-1.55927063913065,
-1.55530274281241,-1.55146139176783,-1.54682467369087,-1.53775892958849,
-1.49709094362333,-1.4751436430194,-1.46979416645313,-1.4671636272084,-1.46525279678868,
-1.46266419502246,-1.45768717370014,-1.42300963777067,-1.40408768184211),
 .UNSPECIFIED.);
#1173=B_SPLINE_CURVE_WITH_KNOTS('',3,(#8554,#8555,#8556,#8557,#8558,#8559,
#8560,#8561,#8562,#8563,#8564,#8565,#8566,#8567,#8568,#8569,#8570,#8571,
#8572,#8573,#8574,#8575,#8576,#8577,#8578,#8579,#8580,#8581,#8582,#8583,
#8584,#8585,#8586,#8587,#8588,#8589,#8590,#8591,#8592,#8593,#8594,#8595,
#8596,#8597,#8598,#8599,#8600,#8601,#8602,#8603,#8604,#8605,#8606,#8607,
#8608,#8609,#8610,#8611,#8612,#8613,#8614,#8615,#8616,#8617,#8618,#8619,
#8620,#8621,#8622,#8623,#8624,#8625,#8626,#8627,#8628,#8629,#8630,#8631,
#8632,#8633,#8634,#8635,#8636,#8637,#8638,#8639,#8640,#8641,#8642,#8643,
#8644,#8645,#8646,#8647,#8648,#8649,#8650,#8651,#8652,#8653,#8654,#8655,
#8656,#8657,#8658,#8659,#8660,#8661,#8662,#8663,#8664,#8665,#8666,#8667,
#8668,#8669,#8670,#8671,#8672,#8673,#8674,#8675,#8676,#8677,#8678,#8679,
#8680,#8681,#8682,#8683,#8684,#8685,#8686,#8687,#8688,#8689,#8690,#8691),
 .UNSPECIFIED.,.F.,.F.,(4,2,2,2,2,2,2,2,2,2,2,2,2,2,2,2,2,2,2,2,2,2,2,2,
2,2,2,2,2,2,2,2,2,2,2,2,2,2,2,2,2,2,2,2,2,2,2,2,2,2,2,2,2,2,2,2,2,2,2,2,
2,2,2,2,2,2,2,2,4),(-0.835256000403932,-0.833903157656945,-0.812359280303279,
-0.772906016290568,-0.761742991407092,-0.756819852231102,-0.753020966189164,
-0.748875386505999,-0.742061750144066,-0.733846448660133,-0.716225295331351,
-0.682393038555207,-0.670960543256474,-0.667361518401213,-0.665096077698588,
-0.662858079276838,-0.659386957525091,-0.648136065023465,-0.626234021226254,
-0.590393904725122,-0.583084292388291,-0.578422273186637,-0.57465956001657,
-0.570310446477138,-0.562519521086389,-0.536709477564335,-0.495947463558973,
-0.490778944313391,-0.488183563551013,-0.486272866385113,-0.483649047011384,
-0.478335014037764,-0.45671853228855,-0.417047993935379,-0.406088929278421,
-0.401199285081014,-0.397404873973042,-0.393242635400209,-0.386350500761623,
-0.350929340560522,-0.318142757303684,-0.312975191761013,-0.310379966516739,
-0.308469219822453,-0.30584512450112,-0.300529844484094,-0.278902452756725,
-0.239199500931647,-0.228409066348316,-0.223473713458805,-0.219672820778468,
-0.215532442801598,-0.208744651543829,-0.172782084351853,-0.140380215201286,
-0.135184352332277,-0.132583528116008,-0.130672982466842,-0.128054645602272,
-0.123348883316926,-0.110283297282169,-0.0704009510092085,-0.0529433306947419,
-0.0469698863250932,-0.0433951641945868,-0.0395659255329625,-0.0357922251787191,
-0.030736217758438,-0.000525840699380102),.UNSPECIFIED.);
#1174=B_SPLINE_CURVE_WITH_KNOTS('',3,(#8692,#8693,#8694,#8695,#8696,#8697,
#8698,#8699,#8700,#8701,#8702,#8703,#8704,#8705,#8706,#8707,#8708,#8709,
#8710,#8711,#8712,#8713,#8714,#8715,#8716,#8717,#8718,#8719,#8720,#8721,
#8722,#8723,#8724,#8725,#8726,#8727,#8728,#8729,#8730,#8731,#8732,#8733,
#8734,#8735,#8736,#8737,#8738,#8739,#8740,#8741,#8742,#8743,#8744,#8745,
#8746,#8747,#8748,#8749,#8750,#8751,#8752,#8753,#8754,#8755,#8756,#8757,
#8758,#8759,#8760,#8761,#8762,#8763),.UNSPECIFIED.,.F.,.F.,(4,2,2,2,2,2,
2,2,2,2,2,2,2,2,2,2,2,2,2,2,2,2,2,2,2,2,2,2,2,2,2,2,2,2,2,4),(-2.23817129971403,
-2.20004353776308,-2.19641612000517,-2.19328204071144,-2.19111031208694,
-2.18874301483652,-2.18467310509577,-2.16661948324098,-2.13761835312644,
-2.11379425744401,-2.10749510880762,-2.10730306054185,-2.10710989232745,
-2.10691338764266,-2.10671107509834,-2.10650008085897,-2.1062769239631,
-2.10603721756826,-2.10577521164799,-2.10548305860718,-2.10514957058804,
-2.10489058491089,-2.10424380038591,-2.10048369441894,-2.0958552735416,
-2.08865934590121,-2.04245770713627,-2.02764573932396,-2.02159127472162,
-2.01693354826721,-2.01444164074152,-2.01230682513711,-2.0094754871114,
-2.00310539243814,-1.96391664450224,-1.95382075976061),.UNSPECIFIED.);
#1175=B_SPLINE_CURVE_WITH_KNOTS('',3,(#8764,#8765,#8766,#8767,#8768,#8769,
#8770,#8771,#8772,#8773,#8774,#8775,#8776,#8777,#8778,#8779,#8780,#8781,
#8782,#8783,#8784,#8785,#8786,#8787,#8788,#8789,#8790,#8791,#8792,#8793,
#8794,#8795,#8796,#8797,#8798,#8799,#8800,#8801,#8802,#8803,#8804,#8805,
#8806,#8807,#8808,#8809,#8810,#8811,#8812,#8813,#8814,#8815,#8816,#8817,
#8818,#8819,#8820,#8821,#8822,#8823,#8824,#8825,#8826,#8827,#8828,#8829,
#8830,#8831,#8832,#8833,#8834,#8835,#8836,#8837,#8838,#8839,#8840,#8841,
#8842,#8843,#8844,#8845,#8846,#8847,#8848,#8849,#8850,#8851,#8852,#8853,
#8854,#8855,#8856,#8857,#8858,#8859,#8860,#8861,#8862,#8863,#8864,#8865,
#8866,#8867,#8868,#8869,#8870,#8871,#8872,#8873,#8874,#8875,#8876,#8877,
#8878,#8879,#8880,#8881,#8882,#8883,#8884,#8885,#8886,#8887,#8888,#8889,
#8890,#8891,#8892,#8893,#8894,#8895,#8896,#8897,#8898,#8899,#8900,#8901,
#8902,#8903,#8904,#8905,#8906,#8907,#8908,#8909,#8910,#8911,#8912,#8913,
#8914,#8915,#8916,#8917,#8918,#8919,#8920,#8921,#8922,#8923,#8924,#8925,
#8926,#8927,#8928,#8929,#8930,#8931,#8932,#8933,#8934,#8935,#8936,#8937,
#8938,#8939,#8940,#8941,#8942,#8943,#8944,#8945,#8946,#8947,#8948,#8949,
#8950,#8951),.UNSPECIFIED.,.F.,.F.,(4,2,2,2,2,2,2,2,2,2,2,2,2,2,2,2,2,2,
2,2,2,2,2,2,2,2,2,2,2,2,2,2,2,2,2,2,2,2,2,2,2,2,2,2,2,2,2,2,2,2,2,2,2,2,
2,2,2,2,2,2,2,2,2,2,2,2,2,2,2,2,2,2,2,2,2,2,2,2,2,2,2,2,2,2,2,2,2,2,2,2,
2,2,2,4),(-1.40408768184211,-1.38957977527783,-1.38254760910776,-1.37835622038408,
-1.37456965438362,-1.36973754043997,-1.3591190653567,-1.31906290772079,
-1.29731495573317,-1.29198685823671,-1.2893604235364,-1.28744974902084,
-1.28485721287769,-1.27986161632148,-1.24537782625693,-1.21126940426693,
-1.20450717764904,-1.20037242202396,-1.1965702310934,-1.1916239938707,-1.18031973079987,
-1.14098594949752,-1.11947709763186,-1.11417486586332,-1.11155342246128,
-1.10943131033475,-1.10672313102682,-1.10096316874451,-1.09293611811218,
-1.06884840798944,-1.0360422700045,-1.02867043304112,-1.02399029516852,
-1.0202262993262,-1.01589042278099,-1.00816435230079,-0.982832809034957,
-0.944442070007762,-0.937444759403386,-0.934722432697565,-0.932550910248748,
-0.930230787290733,-0.926380329303665,-0.910504634429364,-0.861634803291888,
-0.851423795062694,-0.846593799721364,-0.842807469332458,-0.838614872327558,
-0.831577128402275,-0.798030270312757,-0.763460252719972,-0.758469500754523,
-0.755877960791643,-0.75396719045863,-0.751339592492114,-0.746005635888466,
-0.724203683294803,-0.683969226260979,-0.67353866940251,-0.6686868917186,
-0.664907439052627,-0.660682198025089,-0.653488882022884,-0.620090225590341,
-0.585684345425944,-0.580678345683627,-0.578083572752282,-0.576172914840194,
-0.573548641816458,-0.568232018779985,-0.546591071032606,-0.506847054563397,
-0.495957227979738,-0.491079219077355,-0.487286486230984,-0.483118639850554,
-0.476199400510116,-0.441314198016256,-0.408004105087279,-0.40286079443622,
-0.400270399084497,-0.398359485125245,-0.395730433497096,-0.390389313661894,
-0.368521952510856,-0.328087975161761,-0.317838832645986,-0.313018842471736,
-0.30924265359313,-0.304998730755654,-0.297716530745075,-0.288760759917401,
-0.284919832709406),.UNSPECIFIED.);
#1176=B_SPLINE_CURVE_WITH_KNOTS('',3,(#8956,#8957,#8958,#8959,#8960,#8961,
#8962,#8963,#8964,#8965,#8966,#8967,#8968,#8969,#8970,#8971,#8972,#8973,
#8974,#8975,#8976,#8977,#8978,#8979,#8980,#8981,#8982,#8983,#8984,#8985,
#8986,#8987,#8988,#8989,#8990,#8991,#8992,#8993,#8994,#8995,#8996,#8997,
#8998,#8999,#9000,#9001,#9002,#9003,#9004,#9005,#9006,#9007,#9008,#9009,
#9010,#9011,#9012,#9013,#9014,#9015,#9016,#9017,#9018,#9019,#9020,#9021,
#9022,#9023,#9024,#9025,#9026,#9027,#9028,#9029,#9030,#9031,#9032,#9033,
#9034,#9035,#9036,#9037,#9038,#9039,#9040,#9041,#9042,#9043,#9044,#9045,
#9046,#9047,#9048,#9049,#9050,#9051,#9052,#9053,#9054,#9055,#9056,#9057,
#9058,#9059,#9060,#9061,#9062,#9063,#9064,#9065,#9066,#9067,#9068,#9069,
#9070,#9071,#9072,#9073,#9074,#9075,#9076,#9077,#9078,#9079,#9080,#9081,
#9082,#9083,#9084,#9085,#9086,#9087,#9088,#9089,#9090,#9091,#9092,#9093,
#9094,#9095,#9096,#9097,#9098,#9099,#9100,#9101,#9102,#9103,#9104,#9105,
#9106,#9107,#9108,#9109,#9110,#9111,#9112,#9113,#9114,#9115,#9116,#9117,
#9118,#9119,#9120,#9121,#9122,#9123,#9124,#9125,#9126,#9127,#9128,#9129,
#9130,#9131,#9132,#9133,#9134,#9135,#9136,#9137,#9138,#9139,#9140,#9141,
#9142,#9143),.UNSPECIFIED.,.F.,.F.,(4,2,2,2,2,2,2,2,2,2,2,2,2,2,2,2,2,2,
2,2,2,2,2,2,2,2,2,2,2,2,2,2,2,2,2,2,2,2,2,2,2,2,2,2,2,2,2,2,2,2,2,2,2,2,
2,2,2,2,2,2,2,2,2,2,2,2,2,2,2,2,2,2,2,2,2,2,2,2,2,2,2,2,2,2,2,2,2,2,2,2,
2,2,2,4),(-1.95425084573748,-1.9488048353452,-1.9265034475259,-1.91880226621803,
-1.91321778982713,-1.91054292250933,-1.90842225940067,-1.90577172519139,
-1.90031504000988,-1.8750307949933,-1.85220842069598,-1.83119200737488,
-1.82504133564151,-1.82103505619071,-1.81722087565314,-1.81186587393905,
-1.80200383315236,-1.75851717974032,-1.73854180639263,-1.73447773956142,
-1.73211188553927,-1.72996434008032,-1.72684631381955,-1.71909579802802,
-1.68610940505473,-1.65630212209218,-1.64864835940714,-1.64432788703489,
-1.640563121571,-1.63586350133981,-1.62627648002117,-1.58509586145795,-1.56103132328574,
-1.55683423800556,-1.55443942553061,-1.55227861322663,-1.54921024303087,
-1.54179666366109,-1.5085179681387,-1.47679903864488,-1.47008918832085,
-1.46596571971358,-1.46216038813747,-1.45719065976957,-1.44620273467432,
-1.40669390553267,-1.38512791039511,-1.3798198289021,-1.37719743252561,
-1.3752871143026,-1.37269126461299,-1.36751898869572,-1.32681405945243,
-1.30100383799497,-1.29321337380989,-1.28886472298043,-1.28510249963056,
-1.2804412072163,-1.27136734789151,-1.22083982450515,-1.20482486924466,
-1.20096545513965,-1.19864348717774,-1.1964732106804,-1.19375553389689,
-1.18678848318401,-1.1396272115232,-1.11983545923122,-1.11378764292675,
-1.10980145032778,-1.1059283898753,-1.1004625781689,-1.08600083173267,-1.06230310826659,
-1.02927012023504,-1.02411505750058,-1.02152245033762,-1.01961178474448,
-1.01698545049361,-1.01165776158438,-0.98991279172966,-0.949850183639881,
-0.939263623961265,-0.934437007517011,-0.930651131653822,-0.926456766650751,
-0.919410460722941,-0.885650264324294,-0.851353532017681,-0.846338411659938,
-0.843741777320511,-0.841831267552231,-0.839209116342534,-0.835256000403932),
 .UNSPECIFIED.);
#1177=B_SPLINE_CURVE_WITH_KNOTS('',3,(#9145,#9146,#9147,#9148,#9149,#9150,
#9151,#9152,#9153,#9154,#9155,#9156,#9157,#9158,#9159,#9160,#9161,#9162,
#9163,#9164,#9165,#9166,#9167,#9168,#9169,#9170,#9171,#9172,#9173,#9174,
#9175,#9176,#9177,#9178,#9179,#9180,#9181,#9182,#9183,#9184,#9185,#9186,
#9187,#9188,#9189,#9190,#9191,#9192,#9193,#9194),.UNSPECIFIED.,.F.,.F.,
(4,2,2,2,2,2,2,2,2,2,2,2,2,2,2,2,2,2,2,2,2,2,2,2,4),(-0.284919832709406,
-0.268478615398321,-0.237573699351308,-0.22723363851388,-0.223759085365556,
-0.221741974625486,-0.219530950620218,-0.216190734162257,-0.206140542589294,
-0.188053575860309,-0.145918927656313,-0.138458189823389,-0.134135025753909,
-0.130369802853748,-0.125672100899879,-0.116422632003618,-0.103919850873366,
-0.0706983448033028,-0.0507324000467649,-0.0465906968120399,-0.0442076003520664,
-0.0420418358083735,-0.0389449114566336,-0.0353734051747675,-0.000526036917278915),
 .UNSPECIFIED.);
#1178=B_SPLINE_CURVE_WITH_KNOTS('',3,(#9195,#9196,#9197,#9198,#9199,#9200,
#9201,#9202,#9203,#9204,#9205,#9206,#9207,#9208,#9209,#9210,#9211,#9212,
#9213,#9214,#9215,#9216,#9217,#9218,#9219,#9220,#9221,#9222,#9223,#9224,
#9225,#9226,#9227,#9228,#9229,#9230,#9231,#9232,#9233,#9234,#9235,#9236,
#9237,#9238,#9239,#9240,#9241,#9242,#9243,#9244,#9245,#9246,#9247,#9248,
#9249,#9250,#9251,#9252,#9253,#9254,#9255,#9256,#9257,#9258,#9259,#9260,
#9261,#9262,#9263,#9264,#9265,#9266,#9267,#9268,#9269,#9270,#9271,#9272,
#9273,#9274,#9275,#9276,#9277,#9278,#9279,#9280,#9281,#9282,#9283,#9284,
#9285,#9286,#9287,#9288,#9289,#9290,#9291,#9292,#9293,#9294,#9295,#9296,
#9297,#9298,#9299,#9300,#9301,#9302,#9303,#9304,#9305,#9306,#9307,#9308,
#9309,#9310,#9311,#9312,#9313,#9314,#9315,#9316,#9317,#9318,#9319,#9320,
#9321,#9322,#9323,#9324,#9325,#9326,#9327,#9328,#9329,#9330,#9331,#9332,
#9333),.UNSPECIFIED.,.F.,.F.,(4,3,3,3,3,3,3,3,3,3,3,3,3,3,3,3,3,3,3,3,3,
3,3,3,3,3,3,3,3,3,3,3,3,3,3,3,3,3,3,3,3,3,3,3,3,3,4),(84.8230016469243,
84.9294800319919,85.035885845196,85.1422596419165,85.2510514517916,85.3575496036659,
85.4674882425415,85.577426881417,85.6854677190469,85.7967369523817,85.9044808232374,
86.0121588393832,86.1198098017914,86.2274724668646,86.3352547121903,86.443109349129,
86.5511458411805,86.5756215857255,86.683662473221,86.7949317003226,86.9026756201591,
87.0103536848308,87.1180046952373,87.2256674077084,87.3334496992533,87.4413043817755,
87.5493409180866,87.573816290034,87.6818572432399,87.7931264621277,87.9008704494791,
88.0085485821443,88.1161996609114,88.2238624419986,88.3316448020907,88.4394995531984,
88.54753615753,88.5720109943425,88.6800561759704,88.787908823887,88.8956535691258,
89.0033293074333,89.1109748434047,89.2186917097602,89.3264442868578,89.4343611966998,
89.5083060834268),.UNSPECIFIED.);
#1179=B_SPLINE_CURVE_WITH_KNOTS('',3,(#9339,#9340,#9341,#9342,#9343,#9344,
#9345,#9346,#9347),.UNSPECIFIED.,.F.,.F.,(4,1,1,1,1,1,4),(91.106186954104,
91.2534425448399,92.2516372491484,93.2498319534569,94.2480266577654,95.2462213620739,
95.7916382276144),.UNSPECIFIED.);
#1180=B_SPLINE_CURVE_WITH_KNOTS('',3,(#9348,#9349,#9350,#9351,#9352,#9353,
#9354,#9355,#9356,#9357,#9358,#9359,#9360,#9361,#9362,#9363,#9364,#9365,
#9366,#9367,#9368,#9369,#9370,#9371,#9372,#9373,#9374,#9375,#9376,#9377,
#9378,#9379,#9380,#9381,#9382,#9383,#9384,#9385,#9386,#9387,#9388,#9389,
#9390,#9391,#9392,#9393),.UNSPECIFIED.,.F.,.F.,(4,2,2,2,2,2,2,2,2,2,2,2,
2,2,2,2,2,2,2,2,2,2,4),(-2.23890486318736,-2.1921187183875,-2.18288919550491,
-2.17825630531376,-2.17449557784802,-2.17012462176104,-2.16244206011508,
-2.11530710916638,-2.10089665912402,-2.0949452096968,-2.09051708649427,
-2.08819902923615,-2.08628795447926,-2.08370254441095,-2.07858266815642,
-2.03764433987988,-2.01197095058656,-2.00419975052637,-1.99985546585281,
-1.99609348737935,-1.99142792657138,-1.98410364382918,-1.95425084573748),
 .UNSPECIFIED.);
#1181=B_SPLINE_CURVE_WITH_KNOTS('',3,(#9395,#9396,#9397,#9398,#9399,#9400,
#9401,#9402,#9403,#9404,#9405,#9406,#9407,#9408,#9409,#9410,#9411,#9412,
#9413,#9414,#9415,#9416,#9417,#9418,#9419,#9420,#9421,#9422,#9423,#9424,
#9425,#9426,#9427,#9428,#9429,#9430,#9431,#9432,#9433,#9434,#9435,#9436,
#9437,#9438,#9439,#9440,#9441,#9442,#9443),.UNSPECIFIED.,.F.,.F.,(4,3,3,
3,3,3,3,3,3,3,3,3,3,3,3,3,4),(89.5083060834268,89.570205698651,89.6782467845126,
89.7895159868185,89.8972601001135,90.0049383559305,90.1125895548881,90.2202524530328,
90.3280349248704,90.4358897847461,90.5439264925945,90.5684004029595,90.6802091645352,
90.7917344437616,90.9030923633481,91.0142725525455,91.106186954104),
 .UNSPECIFIED.);
#1182=B_SPLINE_CURVE_WITH_KNOTS('',3,(#9444,#9445,#9446,#9447,#9448,#9449,
#9450,#9451,#9452),.UNSPECIFIED.,.F.,.F.,(4,1,1,1,1,1,4),(91.106189856623,
91.566595107268,92.5647898115765,93.562984515885,94.5611792201935,95.559373924502,
95.7927227292494),.UNSPECIFIED.);
#1183=B_SPLINE_CURVE_WITH_KNOTS('',3,(#9460,#9461,#9462,#9463,#9464,#9465),
 .UNSPECIFIED.,.F.,.F.,(4,1,1,4),(0.,0.998194704308485,1.99638940861699,
2.31370279205594),.UNSPECIFIED.);
#1184=B_SPLINE_CURVE_WITH_KNOTS('',3,(#9467,#9468,#9469,#9470,#9471,#9472,
#9473,#9474,#9475,#9476,#9477,#9478,#9479,#9480,#9481,#9482,#9483,#9484,
#9485,#9486,#9487,#9488,#9489,#9490,#9491,#9492,#9493,#9494,#9495,#9496,
#9497,#9498,#9499,#9500,#9501,#9502,#9503,#9504,#9505,#9506,#9507,#9508,
#9509,#9510,#9511,#9512,#9513,#9514,#9515,#9516,#9517,#9518,#9519,#9520,
#9521,#9522,#9523,#9524,#9525,#9526,#9527,#9528,#9529,#9530,#9531,#9532,
#9533,#9534,#9535,#9536,#9537,#9538,#9539,#9540,#9541,#9542,#9543,#9544,
#9545,#9546,#9547,#9548,#9549,#9550,#9551,#9552,#9553,#9554,#9555,#9556,
#9557,#9558,#9559,#9560,#9561,#9562,#9563,#9564,#9565,#9566,#9567,#9568,
#9569,#9570,#9571,#9572,#9573,#9574,#9575,#9576,#9577,#9578,#9579,#9580,
#9581,#9582,#9583,#9584,#9585,#9586,#9587,#9588,#9589,#9590,#9591,#9592,
#9593,#9594,#9595,#9596,#9597,#9598,#9599,#9600,#9601,#9602,#9603,#9604,
#9605,#9606,#9607,#9608,#9609,#9610,#9611,#9612,#9613,#9614,#9615,#9616,
#9617,#9618,#9619,#9620,#9621,#9622,#9623,#9624,#9625,#9626,#9627,#9628,
#9629,#9630,#9631,#9632,#9633,#9634,#9635,#9636,#9637,#9638,#9639,#9640,
#9641,#9642,#9643,#9644,#9645,#9646,#9647,#9648,#9649,#9650,#9651,#9652,
#9653,#9654,#9655,#9656),.UNSPECIFIED.,.F.,.F.,(4,3,3,3,3,3,3,3,3,3,3,3,
3,3,3,3,3,3,3,3,3,3,3,3,3,3,3,3,3,3,3,3,3,3,3,3,3,3,3,3,3,3,3,3,3,3,3,3,
3,3,3,3,3,3,3,3,3,3,3,3,3,3,3,4),(2.31370765917172,2.41522060882339,2.51670184339182,
2.61818497064019,2.71977323634762,2.82141660228884,2.92324139570188,2.99458411292549,
3.09711859878378,3.19950611514853,3.30177834504594,3.40398832525274,3.50616880821478,
3.60835250643925,3.71064239648886,3.8129869464208,3.915514075849,3.99277881723399,
4.09503733104183,4.19714389723365,4.29912907287259,4.40104840137011,4.50293505561395,
4.60482216517742,4.70681324268719,4.80885727804268,4.91108450620713,4.99097352154248,
5.093358017046,5.19559212371012,5.29770656547786,5.3997561560771,5.5017738833334,
5.60379269269114,5.70591553066315,5.80809157024813,5.91044970192135,5.98916822585098,
6.09155363136855,6.19378903128511,6.29590533799785,6.39795714348975,6.49997743318058,
6.60199915045676,6.70412541657074,6.80630517836143,6.90866747705169,6.98736293015948,
7.08971603159645,7.19191852085989,7.2940011652135,7.39601886409793,7.49800465172254,
7.59999151984254,7.70208263861518,7.80422703225764,7.90655400033986,7.98555763446798,
8.08909372668814,8.19246919758474,8.29569493507905,8.39883155622788,8.50192254712059,
8.59689296635125),.UNSPECIFIED.);
#1185=B_SPLINE_CURVE_WITH_KNOTS('',3,(#9658,#9659,#9660,#9661,#9662,#9663,
#9664,#9665,#9666,#9667,#9668,#9669,#9670,#9671,#9672,#9673,#9674,#9675,
#9676,#9677,#9678,#9679,#9680,#9681,#9682,#9683,#9684,#9685,#9686,#9687,
#9688,#9689,#9690,#9691,#9692,#9693,#9694,#9695,#9696,#9697,#9698,#9699,
#9700,#9701,#9702,#9703,#9704,#9705,#9706,#9707,#9708,#9709,#9710,#9711,
#9712,#9713,#9714,#9715,#9716,#9717,#9718,#9719,#9720,#9721,#9722,#9723,
#9724,#9725,#9726,#9727,#9728,#9729,#9730,#9731,#9732,#9733,#9734,#9735,
#9736,#9737,#9738,#9739,#9740,#9741,#9742,#9743,#9744,#9745,#9746,#9747,
#9748,#9749,#9750,#9751,#9752,#9753,#9754,#9755,#9756,#9757,#9758,#9759,
#9760,#9761,#9762,#9763,#9764,#9765,#9766,#9767,#9768,#9769,#9770,#9771,
#9772,#9773,#9774,#9775,#9776,#9777,#9778,#9779,#9780,#9781,#9782,#9783,
#9784,#9785,#9786,#9787,#9788,#9789,#9790,#9791,#9792,#9793,#9794,#9795,
#9796,#9797,#9798,#9799,#9800,#9801,#9802,#9803,#9804,#9805,#9806,#9807,
#9808,#9809,#9810,#9811,#9812,#9813,#9814,#9815,#9816,#9817,#9818,#9819,
#9820,#9821,#9822,#9823,#9824,#9825,#9826,#9827,#9828,#9829,#9830,#9831,
#9832,#9833,#9834,#9835,#9836,#9837,#9838,#9839,#9840,#9841,#9842,#9843,
#9844,#9845,#9846,#9847),.UNSPECIFIED.,.F.,.F.,(4,3,3,3,3,3,3,3,3,3,3,3,
3,3,3,3,3,3,3,3,3,3,3,3,3,3,3,3,3,3,3,3,3,3,3,3,3,3,3,3,3,3,3,3,3,3,3,3,
3,3,3,3,3,3,3,3,3,3,3,3,3,3,3,4),(8.59689296679312,8.71065869504464,8.82488625940654,
8.93970254030743,8.98375233877648,9.08612148663761,9.18834028109337,9.2904395402446,
9.39247403555406,9.49447677718119,9.59648073300154,9.69858902871033,9.80075067590721,
9.90309482774171,9.98194704308498,10.0843125227032,10.1865275760404,10.2886230026925,
10.3906536113638,10.4926524177611,10.5946523952558,10.6967566731526,10.7989142742985,
10.9012543794308,10.9801417473935,11.0825095487835,11.1847269570185,11.2868247768608,
11.3888578010099,11.4908590416982,11.5928614688437,11.6949682032125,11.7971282684864,
11.8994708223271,11.978336451702,12.0807039145387,12.1829209845634,12.2850184683913,
12.3870511580443,12.4890520662475,12.5910541634126,12.6931605740422,12.7953203185295,
12.8976625601372,12.9765311560105,13.0788982177589,13.1811148781567,13.2832119415084,
13.3852442042399,13.4872446796843,13.5892463388556,13.691352306376,13.7935116042178,
13.8958533984137,13.974725860319,14.0758680560039,14.1768398940109,14.2777162292637,
14.3785316339025,14.4793205993077,14.5801813237648,14.6810738307868,14.7821341386101,
14.8800782730761),.UNSPECIFIED.);
#1186=B_SPLINE_CURVE_WITH_KNOTS('',3,(#9849,#9850,#9851,#9852,#9853,#9854,
#9855,#9856,#9857,#9858,#9859,#9860,#9861,#9862,#9863,#9864,#9865,#9866,
#9867,#9868,#9869,#9870,#9871,#9872,#9873,#9874,#9875,#9876,#9877,#9878,
#9879,#9880,#9881,#9882,#9883,#9884,#9885,#9886,#9887,#9888,#9889,#9890,
#9891,#9892,#9893,#9894,#9895,#9896,#9897,#9898,#9899,#9900,#9901,#9902,
#9903,#9904,#9905,#9906,#9907,#9908,#9909,#9910,#9911,#9912,#9913,#9914,
#9915,#9916,#9917,#9918,#9919,#9920,#9921,#9922,#9923,#9924,#9925,#9926,
#9927,#9928,#9929,#9930,#9931,#9932,#9933,#9934,#9935,#9936,#9937,#9938,
#9939,#9940,#9941,#9942,#9943,#9944,#9945,#9946,#9947,#9948,#9949,#9950,
#9951,#9952,#9953,#9954,#9955,#9956,#9957,#9958,#9959,#9960,#9961,#9962,
#9963,#9964,#9965,#9966,#9967,#9968,#9969,#9970,#9971,#9972,#9973,#9974,
#9975,#9976,#9977,#9978,#9979,#9980,#9981,#9982,#9983,#9984,#9985,#9986,
#9987,#9988,#9989,#9990,#9991,#9992,#9993,#9994,#9995,#9996,#9997,#9998,
#9999,#10000,#10001,#10002,#10003,#10004,#10005,#10006,#10007,#10008,#10009,
#10010,#10011,#10012,#10013,#10014,#10015,#10016,#10017,#10018,#10019,#10020,
#10021,#10022,#10023,#10024,#10025,#10026,#10027,#10028,#10029,#10030,#10031,
#10032,#10033,#10034,#10035,#10036,#10037,#10038),.UNSPECIFIED.,.F.,.F.,
(4,3,3,3,3,3,3,3,3,3,3,3,3,3,3,3,3,3,3,3,3,3,3,3,3,3,3,3,3,3,3,3,3,3,3,
3,3,3,3,3,3,3,3,3,3,3,3,3,3,3,3,3,3,3,3,3,3,3,3,3,3,3,3,4),(14.8800782735309,
14.9729205646275,15.0752878658831,15.1775047700189,15.2796020822822,15.3816345969743,
15.4836353270675,15.5856372432181,15.6877434695587,15.78990302765,15.8922450814957,
15.971115268936,16.0734825285195,16.1756993900125,16.27779665838,16.3798291284296,
16.4818298131971,16.5838316834012,16.685937863147,16.7880973742104,16.8904393808467,
16.9693099732445,17.0716772716465,17.1738941725689,17.2759914810917,17.3780239917218,
17.4800247174366,17.5820266288971,17.684132850093,17.7862924027791,17.8886344508497,
17.967504677553,18.0698719653397,18.1720888555592,18.2741861533,18.376218653105,
18.4782193679672,18.5802212685635,18.6823274789533,18.7844870208486,18.8868290582766,
18.9656993818615,19.0680666656384,19.1702835517416,19.2723808452264,19.3744133406915,
19.4764140511363,19.5784159472436,19.6805221530641,19.7826816903382,19.8850237231117,
19.96389408617,20.0662613748044,20.1684782658453,20.2705755643636,20.3726080649186,
20.4746087805025,20.5766106817907,20.6787168928212,20.7808764353296,20.8832184733183,
20.9620887904785,21.1082185625857,21.1632635807104),.UNSPECIFIED.);
#1187=B_SPLINE_CURVE_WITH_KNOTS('',3,(#10040,#10041,#10042,#10043,#10044,
#10045,#10046,#10047,#10048,#10049,#10050,#10051,#10052,#10053,#10054,#10055,
#10056,#10057,#10058,#10059,#10060,#10061,#10062,#10063,#10064,#10065,#10066,
#10067,#10068,#10069,#10070,#10071,#10072,#10073,#10074,#10075,#10076,#10077,
#10078,#10079,#10080,#10081,#10082,#10083,#10084,#10085,#10086,#10087,#10088,
#10089,#10090,#10091,#10092,#10093,#10094,#10095,#10096,#10097,#10098,#10099,
#10100,#10101,#10102,#10103,#10104,#10105,#10106,#10107,#10108,#10109,#10110,
#10111,#10112,#10113,#10114,#10115,#10116,#10117,#10118,#10119,#10120,#10121,
#10122,#10123,#10124,#10125,#10126,#10127,#10128,#10129,#10130,#10131,#10132,
#10133,#10134,#10135,#10136,#10137,#10138,#10139,#10140,#10141,#10142,#10143,
#10144,#10145,#10146,#10147,#10148,#10149,#10150,#10151,#10152,#10153,#10154,
#10155,#10156,#10157,#10158,#10159,#10160,#10161,#10162,#10163,#10164,#10165,
#10166,#10167,#10168,#10169,#10170,#10171,#10172,#10173,#10174,#10175,#10176,
#10177,#10178,#10179,#10180,#10181,#10182,#10183,#10184,#10185,#10186,#10187,
#10188,#10189,#10190,#10191,#10192,#10193,#10194,#10195,#10196,#10197,#10198,
#10199,#10200,#10201,#10202,#10203,#10204,#10205,#10206,#10207,#10208,#10209,
#10210,#10211,#10212,#10213,#10214,#10215,#10216,#10217,#10218,#10219,#10220,
#10221,#10222,#10223,#10224,#10225,#10226,#10227,#10228,#10229),
 .UNSPECIFIED.,.F.,.F.,(4,3,3,3,3,3,3,3,3,3,3,3,3,3,3,3,3,3,3,3,3,3,3,3,
3,3,3,3,3,3,3,3,3,3,3,3,3,3,3,3,3,3,3,3,3,3,3,3,3,3,3,3,3,3,3,3,3,3,3,3,
3,3,3,4),(21.1632635810437,21.263959503826,21.3645711896956,21.4651334149979,
21.5656808869542,21.6663176644117,21.7669966867001,21.8678573289293,21.960283494787,
22.0626507814528,22.1648676704972,22.2669649669871,22.3689974654954,22.4709981790168,
22.5730000782296,22.6751062871795,22.7772658276012,22.8796078635165,22.9584781990955,
23.0608454863558,23.1630623760049,23.265159673112,23.3671921722446,23.4691928863969,
23.5711947862462,23.6733009958367,23.7754605369021,23.8778025734595,23.9566729034039,
24.0590401904257,24.1612570798335,24.2633543766963,24.3653868755827,24.4673875894877,
24.5693894890889,24.6714956984312,24.7736552392482,24.8759972755595,24.9548676077125,
25.0572348947143,25.159451784101,25.2615490809412,25.3635815798042,25.4655822936845,
25.5675841932602,25.669690402576,25.7718499433661,25.8741919796494,25.9530623120209,
26.0554295990936,26.1576464885526,26.2597437854665,26.3617762844044,26.4637769983603,
26.5657788980125,26.6678851074053,26.7700446482726,26.8723866846331,26.9512570163294,
27.0590747241359,27.166577316323,27.2738896157367,27.3809590622594,27.4464488875614),
 .UNSPECIFIED.);
#1188=B_SPLINE_CURVE_WITH_KNOTS('',3,(#10231,#10232,#10233,#10234,#10235,
#10236,#10237,#10238,#10239,#10240,#10241,#10242,#10243,#10244,#10245,#10246,
#10247,#10248,#10249,#10250,#10251,#10252,#10253,#10254,#10255,#10256,#10257,
#10258,#10259,#10260,#10261,#10262,#10263,#10264,#10265,#10266,#10267,#10268,
#10269,#10270,#10271,#10272,#10273,#10274,#10275,#10276,#10277,#10278,#10279,
#10280,#10281,#10282,#10283,#10284,#10285,#10286,#10287,#10288,#10289,#10290,
#10291,#10292,#10293,#10294,#10295,#10296,#10297,#10298,#10299,#10300,#10301,
#10302,#10303,#10304,#10305,#10306,#10307,#10308,#10309,#10310,#10311,#10312,
#10313,#10314,#10315,#10316,#10317,#10318,#10319,#10320,#10321,#10322,#10323,
#10324,#10325,#10326,#10327,#10328,#10329,#10330,#10331,#10332,#10333,#10334,
#10335,#10336,#10337,#10338,#10339,#10340,#10341,#10342,#10343,#10344,#10345,
#10346,#10347,#10348,#10349,#10350,#10351,#10352,#10353,#10354,#10355,#10356,
#10357,#10358,#10359,#10360,#10361,#10362,#10363,#10364,#10365,#10366,#10367,
#10368,#10369,#10370,#10371,#10372,#10373,#10374,#10375,#10376,#10377,#10378,
#10379,#10380,#10381,#10382,#10383,#10384,#10385,#10386,#10387,#10388,#10389,
#10390,#10391,#10392,#10393,#10394,#10395,#10396,#10397,#10398,#10399,#10400,
#10401,#10402,#10403,#10404,#10405,#10406,#10407,#10408,#10409,#10410,#10411,
#10412,#10413,#10414,#10415,#10416,#10417,#10418,#10419,#10420),
 .UNSPECIFIED.,.F.,.F.,(4,3,3,3,3,3,3,3,3,3,3,3,3,3,3,3,3,3,3,3,3,3,3,3,
3,3,3,3,3,3,3,3,3,3,3,3,3,3,3,3,3,3,3,3,3,3,3,3,3,3,3,3,3,3,3,3,3,3,3,3,
3,3,3,4),(27.4464488878901,27.5531138465415,27.660065161629,27.7671651353967,
27.8745554203971,27.9494517206379,28.0518190076774,28.1540358971027,28.2561331939824,
28.3581656928855,28.4601664068066,28.5621683064235,28.6642745157809,28.7664340566127,
28.8687760929379,28.9476464249464,29.0500137119942,29.1522306014279,29.2543278983162,
29.3563603972281,29.458361111158,29.5603630107837,29.66246922015,29.7646287609908,
29.866970797325,29.9458411292549,30.0482084162981,30.1504253057272,30.2525226026107,
30.3545551015178,30.4565558154429,30.5585577150636,30.6606639244251,30.7628234652611,
30.8651655015904,30.9440358335634,31.046403120607,31.1486200100365,31.2507173069205,
31.3527498058281,31.4547505197536,31.5567524193752,31.658858628737,31.7610181695735,
31.8633602059032,31.9422305378719,32.0445978249165,32.146814714347,32.2489120112319,
32.3509445101405,32.452945224067,32.5549471236892,32.6570533330521,32.7592128738895,
32.8615549102202,32.9404252421804,33.0413151814097,33.1420721870169,33.2427311845129,
33.3433269635466,33.443934512472,33.5445428291212,33.6452590321507,33.7296341948134),
 .UNSPECIFIED.);
#1189=B_SPLINE_CURVE_WITH_KNOTS('',3,(#10422,#10423,#10424,#10425,#10426,
#10427,#10428,#10429,#10430,#10431,#10432,#10433,#10434,#10435,#10436,#10437,
#10438,#10439,#10440,#10441,#10442,#10443,#10444,#10445,#10446,#10447,#10448,
#10449,#10450,#10451,#10452,#10453,#10454,#10455,#10456,#10457,#10458,#10459,
#10460,#10461,#10462,#10463,#10464,#10465,#10466,#10467,#10468,#10469,#10470,
#10471,#10472,#10473,#10474,#10475,#10476,#10477,#10478,#10479,#10480,#10481,
#10482,#10483,#10484,#10485,#10486,#10487,#10488,#10489,#10490,#10491,#10492,
#10493,#10494,#10495,#10496,#10497,#10498,#10499,#10500,#10501,#10502,#10503,
#10504,#10505,#10506,#10507,#10508,#10509,#10510,#10511,#10512,#10513,#10514,
#10515,#10516,#10517,#10518,#10519,#10520,#10521,#10522,#10523,#10524,#10525,
#10526,#10527,#10528,#10529,#10530,#10531,#10532,#10533,#10534,#10535,#10536,
#10537,#10538,#10539,#10540,#10541,#10542,#10543,#10544,#10545,#10546,#10547,
#10548,#10549,#10550,#10551,#10552,#10553,#10554,#10555,#10556,#10557,#10558,
#10559,#10560,#10561,#10562,#10563,#10564,#10565,#10566,#10567,#10568,#10569,
#10570,#10571,#10572,#10573,#10574,#10575,#10576,#10577,#10578,#10579,#10580,
#10581,#10582,#10583,#10584,#10585,#10586,#10587,#10588,#10589,#10590,#10591,
#10592,#10593,#10594,#10595,#10596,#10597,#10598,#10599,#10600,#10601,#10602,
#10603,#10604,#10605,#10606,#10607,#10608,#10609,#10610,#10611),
 .UNSPECIFIED.,.F.,.F.,(4,3,3,3,3,3,3,3,3,3,3,3,3,3,3,3,3,3,3,3,3,3,3,3,
3,3,3,3,3,3,3,3,3,3,3,3,3,3,3,3,3,3,3,3,3,3,3,3,3,3,3,3,3,3,3,3,3,3,3,3,
3,3,3,4),(33.7296341950697,33.8730565221767,33.9386199464889,34.040987233533,
34.1432041229628,34.2453014198472,34.3473339187553,34.4493346326813,34.5513365323031,
34.6534427416655,34.7556022825025,34.8579443188328,34.9368146507974,35.0391819378415,
35.1413988272715,35.243496124156,35.345528623064,35.44752933699,35.5495312366119,
35.6516374459743,35.7537969868112,35.8561390231415,35.9350093551059,36.0373766421499,
36.1395935315798,36.2416908284642,36.3437233273722,36.4457240412981,36.5477259409199,
36.6498321502822,36.751991691119,36.8543337274492,36.9332040594144,37.0355713464585,
37.1377882358883,37.2398855327728,37.3419180316808,37.4439187456068,37.5459206452285,
37.6480268545909,37.7501863954277,37.852528431758,37.9313987637229,38.0337660507669,
38.1359829401969,38.2380802370813,38.3401127359893,38.4421134499153,38.5441153495371,
38.6462215588994,38.7483810997363,38.8507231360665,38.9295934680314,39.0319607550755,
39.1341776445054,39.2362749413898,39.3383074402978,39.4403081542238,39.5423100538456,
39.644416263208,39.7465758040449,39.8489178403751,39.9277881723399,40.0128195022493),
 .UNSPECIFIED.);
#1190=B_SPLINE_CURVE_WITH_KNOTS('',3,(#10613,#10614,#10615,#10616,#10617,
#10618,#10619,#10620,#10621,#10622,#10623,#10624,#10625,#10626,#10627,#10628,
#10629,#10630,#10631,#10632,#10633,#10634,#10635,#10636,#10637,#10638,#10639,
#10640,#10641,#10642,#10643,#10644,#10645,#10646,#10647,#10648,#10649,#10650,
#10651,#10652,#10653,#10654,#10655,#10656,#10657,#10658,#10659,#10660,#10661,
#10662,#10663,#10664,#10665,#10666,#10667,#10668,#10669,#10670,#10671,#10672,
#10673,#10674,#10675,#10676,#10677,#10678,#10679,#10680,#10681,#10682,#10683,
#10684,#10685,#10686,#10687,#10688,#10689,#10690,#10691,#10692,#10693,#10694,
#10695,#10696,#10697,#10698,#10699,#10700,#10701,#10702,#10703,#10704,#10705,
#10706,#10707,#10708,#10709,#10710,#10711,#10712,#10713,#10714,#10715,#10716,
#10717,#10718,#10719,#10720,#10721,#10722,#10723,#10724,#10725,#10726,#10727,
#10728,#10729,#10730,#10731,#10732,#10733,#10734,#10735,#10736,#10737,#10738,
#10739,#10740,#10741,#10742,#10743,#10744,#10745,#10746,#10747,#10748,#10749,
#10750,#10751,#10752,#10753,#10754,#10755,#10756,#10757,#10758,#10759,#10760,
#10761,#10762,#10763,#10764,#10765,#10766,#10767,#10768,#10769,#10770,#10771,
#10772,#10773,#10774,#10775,#10776,#10777,#10778,#10779,#10780,#10781,#10782,
#10783,#10784,#10785,#10786,#10787,#10788,#10789,#10790,#10791,#10792,#10793,
#10794,#10795,#10796,#10797,#10798,#10799,#10800,#10801,#10802),
 .UNSPECIFIED.,.F.,.F.,(4,3,3,3,3,3,3,3,3,3,3,3,3,3,3,3,3,3,3,3,3,3,3,3,
3,3,3,3,3,3,3,3,3,3,3,3,3,3,3,3,3,3,3,3,3,3,3,3,3,3,3,3,3,3,3,3,3,3,3,3,
3,3,3,4),(40.0128195026877,40.1139820971137,40.2154821945556,40.3164051406739,
40.4172771797015,40.518132722457,40.6200952610048,40.7210806437024,40.8235317601754,
40.9259828766484,41.0283501636925,41.1305670531224,41.2326643500069,41.334696848915,
41.436697562841,41.5386994624629,41.6408056718253,41.7429652126622,41.8453072489925,
41.9241775809569,42.026544868001,42.1287617574309,42.2308590543154,42.3328915532235,
42.4348922671494,42.5368941667711,42.6390003761335,42.7411599169704,42.8435019533007,
42.9223722852654,43.0247395723094,43.1269564617393,43.2290537586237,43.3310862575318,
43.4330869714578,43.5350888710796,43.6371950804419,43.7393546212787,43.841696657609,
43.9205669895739,44.0229342766178,44.1251511660479,44.2272484629323,44.3292809618403,
44.4312816757661,44.5332835753881,44.6353897847504,44.7375493255873,44.8398913619175,
44.9187616938824,45.0211289809264,45.1233458703563,45.2254431672408,45.3274756661487,
45.4294763800745,45.5314782796963,45.6335844890586,45.7357440298954,45.8380860662257,
45.9169563981909,46.0323952952073,46.1474006819053,46.2616798898559,46.2960048092023),
 .UNSPECIFIED.);
#1191=B_SPLINE_CURVE_WITH_KNOTS('',3,(#10804,#10805,#10806,#10807,#10808,
#10809,#10810,#10811,#10812,#10813,#10814,#10815,#10816,#10817,#10818,#10819,
#10820,#10821,#10822,#10823,#10824,#10825,#10826,#10827,#10828,#10829,#10830,
#10831,#10832,#10833,#10834,#10835,#10836,#10837,#10838,#10839,#10840,#10841,
#10842,#10843,#10844,#10845,#10846,#10847,#10848,#10849,#10850,#10851,#10852,
#10853,#10854,#10855,#10856,#10857,#10858,#10859,#10860,#10861,#10862,#10863,
#10864,#10865,#10866,#10867,#10868,#10869,#10870,#10871,#10872,#10873,#10874,
#10875,#10876,#10877,#10878,#10879,#10880,#10881,#10882,#10883,#10884,#10885,
#10886,#10887,#10888,#10889,#10890,#10891,#10892,#10893,#10894,#10895,#10896,
#10897,#10898,#10899,#10900,#10901,#10902,#10903,#10904,#10905,#10906,#10907,
#10908,#10909,#10910,#10911,#10912,#10913,#10914,#10915,#10916,#10917,#10918,
#10919,#10920,#10921,#10922,#10923,#10924,#10925,#10926,#10927,#10928,#10929,
#10930,#10931,#10932,#10933,#10934,#10935,#10936,#10937,#10938,#10939,#10940,
#10941,#10942,#10943,#10944,#10945,#10946,#10947,#10948,#10949,#10950,#10951,
#10952,#10953,#10954,#10955,#10956,#10957,#10958,#10959,#10960,#10961,#10962,
#10963,#10964,#10965,#10966,#10967,#10968,#10969,#10970,#10971,#10972,#10973,
#10974,#10975,#10976,#10977,#10978,#10979,#10980,#10981,#10982,#10983,#10984,
#10985,#10986,#10987,#10988,#10989,#10990,#10991,#10992,#10993),
 .UNSPECIFIED.,.F.,.F.,(4,3,3,3,3,3,3,3,3,3,3,3,3,3,3,3,3,3,3,3,3,3,3,3,
3,3,3,3,3,3,3,3,3,3,3,3,3,3,3,3,3,3,3,3,3,3,3,3,3,3,3,3,3,3,3,3,3,3,3,3,
3,3,3,4),(46.2960048094288,46.3988769004328,46.5017666821123,46.6051127872091,
46.7081987950647,46.8116749487821,46.9151511024994,47.0175183895434,47.1197352789733,
47.2218325758577,47.3238650747657,47.4258657886916,47.5278676883137,47.629973897676,
47.7321334385129,47.8344754748431,47.9133458068079,48.015713093852,48.1179299832817,
48.2200272801661,48.3220597790741,48.424060493,48.5260623926216,48.628168601984,
48.7303281428208,48.832670179151,48.9115405111164,49.0139077981605,49.1161246875906,
49.218221984475,49.3202544833829,49.4222551973089,49.5242570969307,49.626363306293,
49.7285228471298,49.83086488346,49.9097352154249,50.012102502469,50.1143193918989,
50.2164166887834,50.3184491876915,50.4204499016175,50.5224518012394,50.6245580106018,
50.7267175514387,50.829059587769,50.9079299197334,51.0102972067774,51.1125140962073,
51.2146113930918,51.3166438919998,51.4186446059257,51.5206465055475,51.6227527149098,
51.7249122557464,51.8272542920766,51.9061246240419,52.0082851131966,52.1103000971643,
52.2122030290474,52.3140344574652,52.415822866432,52.5176331112404,52.5791901166084),
 .UNSPECIFIED.);
#1192=B_SPLINE_CURVE_WITH_KNOTS('',3,(#10995,#10996,#10997,#10998,#10999,
#11000,#11001,#11002,#11003,#11004,#11005,#11006,#11007,#11008,#11009,#11010,
#11011,#11012,#11013,#11014,#11015,#11016,#11017,#11018,#11019,#11020,#11021,
#11022,#11023,#11024,#11025,#11026,#11027,#11028,#11029,#11030,#11031,#11032,
#11033,#11034,#11035,#11036,#11037,#11038,#11039,#11040,#11041,#11042,#11043,
#11044,#11045,#11046,#11047,#11048,#11049,#11050,#11051,#11052,#11053,#11054,
#11055,#11056,#11057,#11058,#11059,#11060,#11061,#11062,#11063,#11064,#11065,
#11066,#11067,#11068,#11069,#11070,#11071,#11072,#11073,#11074,#11075,#11076,
#11077,#11078,#11079,#11080,#11081,#11082,#11083,#11084,#11085,#11086,#11087,
#11088,#11089,#11090,#11091,#11092,#11093,#11094,#11095,#11096,#11097,#11098,
#11099,#11100,#11101,#11102,#11103,#11104,#11105,#11106,#11107,#11108,#11109,
#11110,#11111,#11112,#11113,#11114,#11115,#11116,#11117,#11118,#11119,#11120,
#11121,#11122,#11123,#11124,#11125,#11126,#11127,#11128,#11129,#11130,#11131,
#11132,#11133,#11134,#11135,#11136,#11137,#11138,#11139,#11140,#11141,#11142,
#11143,#11144,#11145,#11146,#11147,#11148,#11149,#11150,#11151,#11152,#11153,
#11154,#11155,#11156,#11157,#11158,#11159,#11160,#11161,#11162,#11163,#11164,
#11165,#11166,#11167,#11168,#11169,#11170,#11171,#11172,#11173,#11174,#11175,
#11176,#11177,#11178,#11179,#11180,#11181,#11182,#11183,#11184),
 .UNSPECIFIED.,.F.,.F.,(4,3,3,3,3,3,3,3,3,3,3,3,3,3,3,3,3,3,3,3,3,3,3,3,
3,3,3,3,3,3,3,3,3,3,3,3,3,3,3,3,3,3,3,3,3,3,3,3,3,3,3,3,3,3,3,3,3,3,3,3,
3,3,3,4),(52.5791901170213,52.6988577669334,52.8198639579863,52.9043193283504,
53.006686615395,53.1089035048254,53.2110008017104,53.3130333006189,53.4150340145453,
53.5170359141676,53.6191421235305,53.7213016643679,53.8236437006986,53.9025140326589,
54.0048813197024,54.1070982091317,54.2091955060156,54.3112280049231,54.4132287188485,
54.5152306184698,54.6173368278317,54.719496368668,54.8218384049978,54.9007087369673,
55.0030760240105,55.1052929134395,55.2073902103231,55.3094227092302,55.4114234231553,
55.5134253227762,55.6155315321377,55.7176910729737,55.8200331093031,55.8989034412759,
56.0012707283239,56.1034876177578,56.2055849146462,56.3076174135581,56.409618127488,
56.5116200271138,56.61372623648,56.7158857773207,56.8182278136547,56.8970981455844,
56.9994654326234,57.1016823220481,57.2037796189276,57.3058121178305,57.4078128317515,
57.5098147313683,57.6119209407259,57.714080481558,57.8164225178837,57.8952928498929,
57.9971392720394,58.0988357757483,58.200414347064,58.3019299646778,58.4034163422306,
58.5049071526749,58.6065015936108,58.7081536700367,58.8099768212806,58.8623754235586),
 .UNSPECIFIED.);
#1193=B_SPLINE_CURVE_WITH_KNOTS('',3,(#11186,#11187,#11188,#11189,#11190,
#11191,#11192,#11193,#11194,#11195,#11196,#11197,#11198,#11199,#11200,#11201,
#11202,#11203,#11204,#11205,#11206,#11207,#11208,#11209,#11210,#11211,#11212,
#11213,#11214,#11215,#11216,#11217,#11218,#11219,#11220,#11221,#11222,#11223,
#11224,#11225,#11226,#11227,#11228,#11229,#11230,#11231,#11232,#11233,#11234,
#11235,#11236,#11237,#11238,#11239,#11240,#11241,#11242,#11243,#11244,#11245,
#11246,#11247,#11248,#11249,#11250,#11251,#11252,#11253,#11254,#11255,#11256,
#11257,#11258,#11259,#11260,#11261,#11262,#11263,#11264,#11265,#11266,#11267,
#11268,#11269,#11270,#11271,#11272,#11273,#11274,#11275,#11276,#11277,#11278,
#11279,#11280,#11281,#11282,#11283,#11284,#11285,#11286,#11287,#11288,#11289,
#11290,#11291,#11292,#11293,#11294,#11295,#11296,#11297,#11298,#11299,#11300,
#11301,#11302,#11303,#11304,#11305,#11306,#11307,#11308,#11309,#11310,#11311,
#11312,#11313,#11314,#11315,#11316,#11317,#11318,#11319,#11320,#11321,#11322,
#11323,#11324,#11325,#11326,#11327,#11328,#11329,#11330,#11331,#11332,#11333,
#11334,#11335,#11336,#11337,#11338,#11339,#11340,#11341,#11342,#11343,#11344,
#11345,#11346,#11347,#11348,#11349,#11350,#11351,#11352,#11353,#11354,#11355,
#11356,#11357,#11358,#11359,#11360,#11361,#11362,#11363,#11364,#11365,#11366,
#11367,#11368,#11369,#11370,#11371,#11372,#11373,#11374,#11375),
 .UNSPECIFIED.,.F.,.F.,(4,3,3,3,3,3,3,3,3,3,3,3,3,3,3,3,3,3,3,3,3,3,3,3,
3,3,3,3,3,3,3,3,3,3,3,3,3,3,3,3,3,3,3,3,3,3,3,3,3,3,3,3,3,3,3,3,3,3,3,3,
3,3,3,4),(58.862375423788,58.8934875542014,58.9958548412757,59.0980717307357,
59.2001690276505,59.3022015265887,59.4042022405448,59.5062041401967,59.6083103495887,
59.710469890455,59.8128119268141,59.8916822585099,59.994049545507,60.0962664348901,
60.1983637317282,60.3003962305901,60.4023969444703,60.5043988440467,60.6065050533647,
60.7086645941575,60.811006630445,60.8898769628183,60.9922442498436,61.0944611392541,
61.1965584361184,61.2985909350059,61.4005916489109,61.5025935485113,61.6046997578518,
61.7068592986666,61.8092013349746,61.8880716671269,61.9904389543974,62.0926558440545,
62.1947531411662,62.2967856403013,62.398786354454,62.5007882543017,62.6028944638873,
62.7050540049462,62.8073960414941,62.8862663714353,62.9886336580651,63.0908505470813,
63.1929478435552,63.2949803420546,63.3969810555746,63.4989829547935,63.6010891637607,
63.703248704206,63.805590740155,63.8844610757438,63.9868283627835,64.0890452522045,
64.1911425490737,64.2931750479625,64.3951757618653,64.4971776614602,64.5992838707899,
64.7014434115909,64.8037854478806,64.8826557800523,65.0141082553449,65.1455607306376),
 .UNSPECIFIED.);
#1194=B_SPLINE_CURVE_WITH_KNOTS('',3,(#11377,#11378,#11379,#11380,#11381,
#11382,#11383,#11384,#11385,#11386,#11387,#11388,#11389,#11390,#11391,#11392,
#11393,#11394,#11395,#11396,#11397,#11398,#11399,#11400,#11401,#11402,#11403,
#11404,#11405,#11406,#11407,#11408,#11409,#11410,#11411,#11412,#11413,#11414,
#11415,#11416,#11417,#11418,#11419,#11420,#11421,#11422,#11423,#11424,#11425,
#11426,#11427,#11428,#11429,#11430,#11431,#11432,#11433,#11434,#11435,#11436,
#11437,#11438,#11439,#11440,#11441,#11442,#11443,#11444,#11445,#11446,#11447,
#11448,#11449,#11450,#11451,#11452,#11453,#11454,#11455,#11456,#11457,#11458,
#11459,#11460,#11461,#11462,#11463,#11464,#11465,#11466,#11467,#11468,#11469,
#11470,#11471,#11472,#11473,#11474,#11475,#11476,#11477,#11478,#11479,#11480,
#11481,#11482,#11483,#11484,#11485,#11486,#11487,#11488,#11489,#11490,#11491,
#11492,#11493,#11494,#11495,#11496,#11497,#11498,#11499,#11500,#11501,#11502,
#11503,#11504,#11505,#11506,#11507,#11508,#11509,#11510,#11511,#11512,#11513,
#11514,#11515,#11516,#11517,#11518,#11519,#11520,#11521,#11522,#11523,#11524,
#11525,#11526,#11527,#11528,#11529,#11530,#11531,#11532,#11533,#11534,#11535,
#11536,#11537,#11538,#11539,#11540,#11541,#11542,#11543,#11544,#11545,#11546,
#11547,#11548,#11549,#11550,#11551,#11552,#11553,#11554,#11555,#11556,#11557,
#11558,#11559,#11560,#11561,#11562,#11563,#11564,#11565,#11566,#11567,#11568,
#11569),.UNSPECIFIED.,.F.,.F.,(4,3,3,3,3,3,3,3,3,3,3,3,3,3,3,3,3,3,3,3,
3,3,3,3,3,3,3,3,3,3,3,3,3,3,3,3,3,3,3,3,3,3,3,3,3,3,3,3,3,3,3,3,3,3,3,3,
3,3,3,3,3,3,3,3,4),(65.1455607309676,65.2465970860342,65.3475764640722,
65.4485331628698,65.5495014454226,65.6505785552467,65.7517207397834,65.8530285697123,
65.8808504843608,65.9832177678549,66.0854346537376,66.1875319470962,66.2895644424929,
66.391565152927,66.4935670490809,66.5956732550371,66.6978327924965,66.8001748255344,
66.8790451886693,66.9814124768186,67.0836293673207,67.1857266652233,67.2877591651159,
67.3897598799921,67.4917617805283,67.593867990744,67.6960275324017,67.7983695694907,
67.8772398929778,67.9796071917191,68.0818240929058,68.1839214015799,68.2859539122919,
68.3879546380194,68.4899565494237,68.5920627704566,68.6942223229205,68.7965643706738,
68.8754345972863,68.9778018546988,69.0800187145001,69.1821159818993,69.284148451424,
69.3861491361093,69.4881510066736,69.5902571874619,69.6924166999477,69.7947587086134,
69.8736293015948,69.9759966061904,70.0782135129289,70.1803108266821,70.2823433421819,
70.384344072402,70.4863459879989,70.5884522127361,70.6906117686395,70.7929538193632,
70.8718240059033,70.9770412680876,71.0820752466858,71.1869128579018,71.2916343404495,
71.3962479390824,71.4287460381472),.UNSPECIFIED.);
#1195=B_SPLINE_CURVE_WITH_KNOTS('',3,(#11571,#11572,#11573,#11574,#11575,
#11576,#11577,#11578,#11579,#11580,#11581,#11582,#11583,#11584,#11585,#11586,
#11587,#11588,#11589,#11590,#11591,#11592,#11593,#11594,#11595,#11596,#11597,
#11598,#11599,#11600,#11601,#11602,#11603,#11604,#11605,#11606,#11607,#11608,
#11609,#11610,#11611,#11612,#11613,#11614,#11615,#11616,#11617,#11618,#11619,
#11620,#11621,#11622,#11623,#11624,#11625,#11626,#11627,#11628,#11629,#11630,
#11631,#11632,#11633,#11634,#11635,#11636,#11637,#11638,#11639,#11640,#11641,
#11642,#11643,#11644,#11645,#11646,#11647,#11648,#11649,#11650,#11651,#11652,
#11653,#11654,#11655,#11656,#11657,#11658,#11659,#11660,#11661,#11662,#11663,
#11664,#11665,#11666,#11667,#11668,#11669,#11670,#11671,#11672,#11673,#11674,
#11675,#11676,#11677,#11678,#11679,#11680,#11681,#11682,#11683,#11684,#11685,
#11686,#11687,#11688,#11689,#11690,#11691,#11692,#11693,#11694,#11695,#11696,
#11697,#11698,#11699,#11700,#11701,#11702,#11703,#11704,#11705,#11706,#11707,
#11708,#11709,#11710,#11711,#11712,#11713,#11714,#11715,#11716,#11717,#11718,
#11719,#11720,#11721,#11722,#11723,#11724,#11725,#11726,#11727,#11728,#11729,
#11730,#11731,#11732,#11733,#11734,#11735,#11736,#11737,#11738,#11739,#11740,
#11741,#11742,#11743,#11744,#11745,#11746,#11747,#11748,#11749,#11750,#11751,
#11752,#11753,#11754,#11755,#11756,#11757,#11758,#11759,#11760),
 .UNSPECIFIED.,.F.,.F.,(4,3,3,3,3,3,3,3,3,3,3,3,3,3,3,3,3,3,3,3,3,3,3,3,
3,3,3,3,3,3,3,3,3,3,3,3,3,3,3,3,3,3,3,3,3,3,3,3,3,3,3,3,3,3,3,3,3,3,3,3,
3,3,3,4),(71.4287460384322,71.5390642063771,71.6493304527982,71.7600455583879,
71.8700187102118,71.9723857556817,72.0746024033946,72.1766994594859,72.2787317182815,
72.3807321931089,72.4827338549799,72.5848398303166,72.6869991388247,72.7893409482387,
72.8682134145203,72.9705809069235,73.0727979999874,73.1748954970022,73.2769281938039,
73.3789291031275,73.4809311953892,73.583037591822,73.6851973169359,73.7875395309029,
73.8664081188288,73.9687759209844,74.070993329816,74.1730911499998,74.275124174334,
74.3771254150513,74.4791278420698,74.581234576071,74.6833946408433,74.7857371939683,
74.8646028231373,74.9669681838356,75.0691831445056,75.1712785181177,75.273309098035,
75.3753078999236,75.4773078971386,75.5794122321338,75.6815699111982,75.7839101275024,
75.8627975274458,75.9651669290334,76.0673859212011,76.1694852935143,76.2715198501672,
76.373522601406,76.4755265151415,76.5776346890152,76.6797961699537,76.7821400845837,
76.8609922317543,76.9618586074584,77.0625535278487,77.163152743669,77.2636910931968,
77.3642033289405,77.464774699641,77.5653792250282,77.6661163902905,77.7119313453268),
 .UNSPECIFIED.);
#1196=B_SPLINE_CURVE_WITH_KNOTS('',3,(#11762,#11763,#11764,#11765,#11766,
#11767,#11768,#11769,#11770,#11771),.UNSPECIFIED.,.F.,.F.,(4,1,1,1,1,1,
1,4),(77.7119313453268,77.8591869360628,78.8573816403713,79.8555763446798,
80.8537710489883,81.8519657532968,82.8501604576053,83.7753903812219),
 .UNSPECIFIED.);
#1197=B_SPLINE_CURVE_WITH_KNOTS('',3,(#11775,#11776,#11777,#11778,#11779,
#11780,#11781,#11782,#11783),.UNSPECIFIED.,.F.,.F.,(4,1,1,1,1,1,4),(-85.8447445705308,
-84.8465498662224,-83.8483551619139,-82.8501604576054,-81.8519657532969,
-80.8537710489884,-80.6873799771529),.UNSPECIFIED.);
#1198=B_SPLINE_CURVE_WITH_KNOTS('',3,(#11785,#11786,#11787,#11788,#11789,
#11790,#11791,#11792,#11793,#11794,#11795,#11796,#11797,#11798,#11799,#11800,
#11801,#11802,#11803,#11804,#11805,#11806,#11807,#11808,#11809,#11810,#11811,
#11812,#11813,#11814,#11815,#11816,#11817,#11818,#11819,#11820,#11821,#11822,
#11823,#11824,#11825,#11826,#11827,#11828,#11829,#11830,#11831,#11832,#11833,
#11834,#11835,#11836,#11837,#11838,#11839,#11840,#11841,#11842,#11843,#11844,
#11845,#11846,#11847,#11848,#11849,#11850,#11851,#11852,#11853,#11854,#11855,
#11856,#11857,#11858,#11859,#11860,#11861,#11862,#11863,#11864,#11865,#11866,
#11867,#11868,#11869,#11870,#11871,#11872,#11873,#11874,#11875,#11876,#11877,
#11878,#11879,#11880,#11881,#11882,#11883,#11884,#11885,#11886,#11887,#11888,
#11889,#11890,#11891,#11892,#11893,#11894,#11895,#11896,#11897,#11898,#11899,
#11900,#11901,#11902,#11903,#11904,#11905,#11906,#11907,#11908,#11909,#11910,
#11911,#11912,#11913,#11914,#11915,#11916,#11917,#11918,#11919,#11920,#11921,
#11922,#11923,#11924,#11925,#11926,#11927,#11928,#11929,#11930,#11931,#11932,
#11933,#11934,#11935,#11936,#11937,#11938,#11939,#11940,#11941,#11942,#11943,
#11944,#11945,#11946,#11947,#11948,#11949,#11950,#11951,#11952,#11953,#11954,
#11955,#11956,#11957,#11958,#11959,#11960,#11961,#11962,#11963,#11964,#11965,
#11966,#11967,#11968,#11969,#11970,#11971,#11972,#11973,#11974,#11975,#11976,
#11977),.UNSPECIFIED.,.F.,.F.,(4,3,3,3,3,3,3,3,3,3,3,3,3,3,3,3,3,3,3,3,
3,3,3,3,3,3,3,3,3,3,3,3,3,3,3,3,3,3,3,3,3,3,3,3,3,3,3,3,3,3,3,3,3,3,3,3,
3,3,3,3,3,3,3,3,4),(-80.6873799771529,-80.5834045230938,-80.4828226165599,
-80.3823020159699,-80.2818079446396,-80.1813056668607,-80.0806994109687,
-79.980030174353,-79.8792001208896,-79.8555763446799,-79.7531909320388,
-79.6509555248073,-79.5488392105263,-79.4467873973145,-79.3447670997625,
-79.2427453744942,-79.1406191002387,-79.0384393302107,-78.9360770232174,
-78.8573816403714,-78.7550285516865,-78.6528260753717,-78.5507434441998,
-78.4487257586336,-78.3467399844452,-78.2447531298611,-78.1426620246853,
-78.0405176446954,-77.9381906902025,-77.8591869360629,-77.7568164895759,
-77.65459642229,-77.5524959355451,-77.4504602410313,-77.348456330411,-77.2464512376597,
-77.1443418632008,-77.0421791678361,-76.9398340304818,-76.8609922317544,
-76.7586230828059,-76.6564042872302,-76.5543050269147,-76.4522705304144,
-76.3502677875718,-76.2482638305126,-76.146155533537,-76.0439938850559,
-75.9416497319229,-75.8627975274459,-75.7604320499599,-75.658216998789,
-75.5561215743442,-75.4540909679041,-75.352092163759,-75.2500921885347,
-75.1479879129198,-75.045830314066,-74.9434902112166,-74.8646028231374,
-74.7495007849462,-74.6402031683395,-74.5311448668227,-74.422403289531,
-74.4041946703725),.UNSPECIFIED.);
#1199=B_SPLINE_CURVE_WITH_KNOTS('',3,(#11979,#11980,#11981,#11982,#11983,
#11984,#11985,#11986,#11987,#11988,#11989,#11990,#11991,#11992,#11993,#11994,
#11995,#11996,#11997,#11998,#11999,#12000,#12001,#12002,#12003,#12004,#12005,
#12006,#12007,#12008,#12009,#12010,#12011,#12012,#12013,#12014,#12015,#12016,
#12017,#12018,#12019,#12020,#12021,#12022,#12023,#12024,#12025,#12026,#12027,
#12028,#12029,#12030,#12031,#12032,#12033,#12034,#12035,#12036,#12037,#12038,
#12039,#12040,#12041,#12042,#12043,#12044,#12045,#12046,#12047,#12048,#12049,
#12050,#12051,#12052,#12053,#12054,#12055,#12056,#12057,#12058,#12059,#12060,
#12061,#12062,#12063,#12064,#12065,#12066,#12067,#12068,#12069,#12070,#12071,
#12072,#12073,#12074,#12075,#12076,#12077,#12078,#12079,#12080,#12081,#12082,
#12083,#12084,#12085,#12086,#12087,#12088,#12089,#12090,#12091,#12092,#12093,
#12094,#12095,#12096,#12097,#12098,#12099,#12100,#12101,#12102,#12103,#12104,
#12105,#12106,#12107,#12108,#12109,#12110,#12111,#12112,#12113,#12114,#12115,
#12116,#12117,#12118,#12119,#12120,#12121,#12122,#12123,#12124,#12125,#12126,
#12127,#12128,#12129,#12130,#12131,#12132,#12133,#12134,#12135,#12136,#12137,
#12138,#12139,#12140,#12141,#12142,#12143,#12144,#12145,#12146,#12147,#12148,
#12149,#12150,#12151,#12152,#12153,#12154,#12155,#12156,#12157,#12158,#12159,
#12160,#12161,#12162,#12163,#12164,#12165,#12166,#12167,#12168),
 .UNSPECIFIED.,.F.,.F.,(4,3,3,3,3,3,3,3,3,3,3,3,3,3,3,3,3,3,3,3,3,3,3,3,
3,3,3,3,3,3,3,3,3,3,3,3,3,3,3,3,3,3,3,3,3,3,3,3,3,3,3,3,3,3,3,3,3,3,3,3,
3,3,3,4),(-74.4041946699734,-74.2989154700527,-74.1907886322468,-74.0851817966569,
-73.9757949577429,-73.8664081188289,-73.7640406558711,-73.6618235857204,
-73.5597261017602,-73.4576934119709,-73.3556925036279,-73.2536904063192,
-73.1515839955417,-73.0494242509036,-72.9470820091423,-72.8682134145204,
-72.7658463531009,-72.6636296930376,-72.5615326300271,-72.4595003676406,
-72.3574998925447,-72.2554982337247,-72.1533922665579,-72.0512329690712,
-71.9488911752294,-71.8700187102119,-71.7676513447524,-71.665434376083,
-71.5633369991085,-71.4613044196293,-71.3593036247673,-71.2573016439608,
-71.1551953535957,-71.0530357317292,-70.9506936152493,-70.8718240059034,
-70.7694567046396,-70.6672398004949,-70.565142488222,-70.4631099735199,
-70.3611092434162,-70.2591073272548,-70.1570011009025,-70.0548415427991,
-69.9524994889408,-69.8736293015949,-69.7712620420592,-69.6690451806148,
-69.566947912297,-69.4649154422974,-69.3629147575807,-69.2609128874278,
-69.1588067077335,-69.056647196722,-68.9543051901375,-68.8754345972864,
-68.7743268238781,-68.6733543158174,-68.5724823531886,-68.4716763501524,
-68.3708710416405,-68.2700671456386,-68.1691815073704,-68.1210093627937),
 .UNSPECIFIED.);
#1200=B_SPLINE_CURVE_WITH_KNOTS('',3,(#12170,#12171,#12172,#12173,#12174,
#12175,#12176,#12177,#12178,#12179,#12180,#12181,#12182,#12183,#12184,#12185,
#12186,#12187,#12188,#12189,#12190,#12191,#12192,#12193,#12194,#12195,#12196,
#12197,#12198,#12199,#12200,#12201,#12202,#12203,#12204,#12205,#12206,#12207,
#12208,#12209,#12210,#12211,#12212,#12213,#12214,#12215,#12216,#12217,#12218,
#12219,#12220,#12221,#12222,#12223,#12224,#12225,#12226,#12227,#12228,#12229,
#12230,#12231,#12232,#12233,#12234,#12235,#12236,#12237,#12238,#12239,#12240,
#12241,#12242,#12243,#12244,#12245,#12246,#12247,#12248,#12249,#12250,#12251,
#12252,#12253,#12254,#12255,#12256,#12257,#12258,#12259,#12260,#12261,#12262,
#12263,#12264,#12265,#12266,#12267,#12268,#12269,#12270,#12271,#12272,#12273,
#12274,#12275,#12276,#12277,#12278,#12279,#12280,#12281,#12282,#12283,#12284,
#12285,#12286,#12287,#12288,#12289,#12290,#12291,#12292,#12293,#12294,#12295,
#12296,#12297,#12298,#12299,#12300,#12301,#12302,#12303,#12304,#12305,#12306,
#12307,#12308,#12309,#12310,#12311,#12312,#12313,#12314,#12315,#12316,#12317,
#12318,#12319,#12320,#12321,#12322,#12323,#12324,#12325,#12326,#12327,#12328,
#12329,#12330,#12331,#12332,#12333,#12334,#12335,#12336,#12337,#12338,#12339,
#12340,#12341,#12342,#12343,#12344,#12345,#12346,#12347,#12348,#12349,#12350,
#12351,#12352,#12353,#12354,#12355,#12356,#12357,#12358,#12359),
 .UNSPECIFIED.,.F.,.F.,(4,3,3,3,3,3,3,3,3,3,3,3,3,3,3,3,3,3,3,3,3,3,3,3,
3,3,3,3,3,3,3,3,3,3,3,3,3,3,3,3,3,3,3,3,3,3,3,3,3,3,3,3,3,3,3,3,3,3,3,3,
3,3,3,4),(-68.1210093625646,-67.9871254872857,-67.8772398929779,-67.7748726051917,
-67.6726557149727,-67.5705584172322,-67.4685259174276,-67.3665252025655,
-67.2645233019694,-67.1624170915797,-67.0602575496844,-66.9579155122564,
-66.8790451886694,-66.7766779048991,-66.6744610188026,-66.5723637253247,
-66.4703312298665,-66.3683305194287,-66.2663286233285,-66.1642224175153,
-66.0620628802484,-65.959720847482,-65.8808504843609,-65.7784831957226,
-65.676266304678,-65.5741690061558,-65.4721365055967,-65.3701357900088,
-65.2681338887165,-65.166027677682,-65.0638681351694,-64.9615260971768,
-64.8826557800524,-64.7802884930504,-64.6780716036587,-64.5759743068065,
-64.4739418079271,-64.371941094026,-64.2699391944252,-64.1678329850779,
-64.0656734442527,-63.9633314079284,-63.8844610757439,-63.7820937890789,
-63.6798769000354,-63.5777796035463,-63.4757471050391,-63.3737463915186,
-63.2717444923066,-63.1696382833577,-63.067478742937,-62.9651367070226,
-62.8862663714354,-62.7838990841745,-62.6816821945248,-62.579584897417,
-62.4775523982838,-62.3755516841309,-62.2735497842809,-62.1714435746897,
-62.0692840336235,-61.9669419970654,-61.8880716671269,-61.8378240556142),
 .UNSPECIFIED.);
#1201=B_SPLINE_CURVE_WITH_KNOTS('',3,(#12361,#12362,#12363,#12364,#12365,
#12366,#12367,#12368,#12369,#12370,#12371,#12372,#12373,#12374,#12375,#12376,
#12377,#12378,#12379,#12380,#12381,#12382,#12383,#12384,#12385,#12386,#12387,
#12388,#12389,#12390,#12391,#12392,#12393,#12394,#12395,#12396,#12397,#12398,
#12399,#12400,#12401,#12402,#12403,#12404,#12405,#12406,#12407,#12408,#12409,
#12410,#12411,#12412,#12413,#12414,#12415,#12416,#12417,#12418,#12419,#12420,
#12421,#12422,#12423,#12424,#12425,#12426,#12427,#12428,#12429,#12430,#12431,
#12432,#12433,#12434,#12435,#12436,#12437,#12438,#12439,#12440,#12441,#12442,
#12443,#12444,#12445,#12446,#12447,#12448,#12449,#12450,#12451,#12452,#12453,
#12454,#12455,#12456,#12457,#12458,#12459,#12460,#12461,#12462,#12463,#12464,
#12465,#12466,#12467,#12468,#12469,#12470,#12471,#12472,#12473,#12474,#12475,
#12476,#12477,#12478,#12479,#12480,#12481,#12482,#12483,#12484,#12485,#12486,
#12487,#12488,#12489,#12490,#12491,#12492,#12493,#12494,#12495,#12496,#12497,
#12498,#12499,#12500,#12501,#12502,#12503,#12504,#12505,#12506,#12507,#12508,
#12509,#12510,#12511,#12512,#12513,#12514,#12515,#12516,#12517,#12518,#12519,
#12520,#12521,#12522,#12523,#12524,#12525,#12526,#12527,#12528,#12529,#12530,
#12531,#12532,#12533,#12534,#12535,#12536,#12537,#12538,#12539,#12540,#12541,
#12542,#12543,#12544,#12545,#12546,#12547,#12548,#12549,#12550),
 .UNSPECIFIED.,.F.,.F.,(4,3,3,3,3,3,3,3,3,3,3,3,3,3,3,3,3,3,3,3,3,3,3,3,
3,3,3,3,3,3,3,3,3,3,3,3,3,3,3,3,3,3,3,3,3,3,3,3,3,3,3,3,3,3,3,3,3,3,3,3,
3,3,3,4),(-61.8378240552875,-61.7362592426383,-61.6304614576608,-61.5291566919834,
-61.4279088057521,-61.3266837808246,-61.2254476335928,-61.1241031222742,
-61.0226944346116,-60.9211196171127,-60.8898769628184,-60.7875096758169,
-60.6852927864304,-60.5831954895903,-60.4811629907274,-60.379162276847,
-60.2771603772715,-60.1750541679557,-60.0728946271658,-59.9705525908826,
-59.8916822585099,-59.7893149714371,-59.6870980819781,-59.585000785064,
-59.4829682861259,-59.3809675721698,-59.2789656725175,-59.1768594631247,
-59.0746999222572,-58.9723578858965,-58.8934875542014,-58.7911202671623,
-58.6889033777374,-58.5868060808579,-58.4847735819549,-58.3827728680338,
-58.2807709684166,-58.178664759059,-58.076505218227,-57.9741631819014,-57.8952928498929,
-57.7929255628534,-57.6907086734283,-57.5886113765486,-57.4865788776455,
-57.3845781637245,-57.2825762641079,-57.1804700547506,-57.078310513919,
-56.9759684775939,-56.8970981455844,-56.7947308585367,-56.6925139691031,
-56.5904166722148,-56.488384173303,-56.3863834593731,-56.284381559747,-56.1822753503807,
-56.0801158095398,-55.9777737732056,-55.8989034412759,-55.7799885722811,
-55.66215376343,-55.5546387488805),.UNSPECIFIED.);
#1202=B_SPLINE_CURVE_WITH_KNOTS('',3,(#12552,#12553,#12554,#12555,#12556,
#12557,#12558,#12559,#12560,#12561,#12562,#12563,#12564,#12565,#12566,#12567,
#12568,#12569,#12570,#12571,#12572,#12573,#12574,#12575,#12576,#12577,#12578,
#12579,#12580,#12581,#12582,#12583,#12584,#12585,#12586,#12587,#12588,#12589,
#12590,#12591,#12592,#12593,#12594,#12595,#12596,#12597,#12598,#12599,#12600,
#12601,#12602,#12603,#12604,#12605,#12606,#12607,#12608,#12609,#12610,#12611,
#12612,#12613,#12614,#12615,#12616,#12617,#12618,#12619,#12620,#12621,#12622,
#12623,#12624,#12625,#12626,#12627,#12628,#12629,#12630,#12631,#12632,#12633,
#12634,#12635,#12636,#12637,#12638,#12639,#12640,#12641,#12642,#12643,#12644,
#12645,#12646,#12647,#12648,#12649,#12650,#12651,#12652,#12653,#12654,#12655,
#12656,#12657,#12658,#12659,#12660,#12661,#12662,#12663,#12664,#12665,#12666,
#12667,#12668,#12669,#12670,#12671,#12672,#12673,#12674,#12675,#12676,#12677,
#12678,#12679,#12680,#12681,#12682,#12683,#12684,#12685,#12686,#12687,#12688,
#12689,#12690,#12691,#12692,#12693,#12694,#12695,#12696,#12697,#12698,#12699,
#12700,#12701,#12702,#12703,#12704,#12705,#12706,#12707,#12708,#12709,#12710,
#12711,#12712,#12713,#12714,#12715,#12716,#12717,#12718,#12719,#12720,#12721,
#12722,#12723,#12724,#12725,#12726,#12727,#12728,#12729,#12730,#12731,#12732,
#12733,#12734,#12735,#12736,#12737,#12738,#12739,#12740,#12741,#12742,#12743,
#12744),.UNSPECIFIED.,.F.,.F.,(4,3,3,3,3,3,3,3,3,3,3,3,3,3,3,3,3,3,3,3,
3,3,3,3,3,3,3,3,3,3,3,3,3,3,3,3,3,3,3,3,3,3,3,3,3,3,3,3,3,3,3,3,3,3,3,3,
3,3,3,3,3,3,3,3,4),(-55.5546387484345,-55.4524945919236,-55.3503595415392,
-55.2482010148576,-55.145916884721,-55.0435604152556,-54.9410225331627,
-54.9007087369674,-54.7983414499237,-54.6961245604944,-54.5940272636104,
-54.491994764703,-54.3899940507776,-54.2879921511563,-54.1858859417944,
-54.0837264009581,-53.9813843646284,-53.9025140326589,-53.8001467456144,
-53.697929856184,-53.595832559299,-53.4938000603905,-53.391799346464,-53.2897974468418,
-53.1876912374789,-53.0855316966414,-52.9831896603107,-52.9043193283504,
-52.8019520413066,-52.6997351518768,-52.5976378549925,-52.4956053560847,
-52.3936046421589,-52.2916027425373,-52.189496533175,-52.0873369923383,
-51.9849949560081,-51.9061246240419,-51.803757336998,-51.7015404475684,
-51.599443150684,-51.4974106517761,-51.3954099378501,-51.2934080382284,
-51.1913018288661,-51.0891422880293,-50.9868002516991,-50.9079299197334,
-50.8055626326894,-50.7033457432593,-50.6012484463748,-50.4992159474668,
-50.397215233541,-50.295213333919,-50.1931071245565,-50.0909475837196,-49.9886055473893,
-49.9097352154249,-49.8068704917154,-49.7041587195511,-49.6015675718968,
-49.499067717916,-49.3966196681602,-49.2941789169835,-49.271453441255),
 .UNSPECIFIED.);
#1203=B_SPLINE_CURVE_WITH_KNOTS('',3,(#12746,#12747,#12748,#12749,#12750,
#12751,#12752,#12753,#12754,#12755,#12756,#12757,#12758,#12759,#12760,#12761,
#12762,#12763,#12764,#12765,#12766,#12767,#12768,#12769,#12770,#12771,#12772,
#12773,#12774,#12775,#12776,#12777,#12778,#12779,#12780,#12781,#12782,#12783,
#12784,#12785,#12786,#12787,#12788,#12789,#12790,#12791,#12792,#12793,#12794,
#12795,#12796,#12797,#12798,#12799,#12800,#12801,#12802,#12803,#12804,#12805,
#12806,#12807,#12808,#12809,#12810,#12811,#12812,#12813,#12814,#12815,#12816,
#12817,#12818,#12819,#12820,#12821,#12822,#12823,#12824,#12825,#12826,#12827,
#12828,#12829,#12830,#12831,#12832,#12833,#12834,#12835,#12836,#12837,#12838,
#12839,#12840,#12841,#12842,#12843,#12844,#12845,#12846,#12847,#12848,#12849,
#12850,#12851,#12852,#12853,#12854,#12855,#12856,#12857,#12858,#12859,#12860,
#12861,#12862,#12863,#12864,#12865,#12866,#12867,#12868,#12869,#12870,#12871,
#12872,#12873,#12874,#12875,#12876,#12877,#12878,#12879,#12880,#12881,#12882,
#12883,#12884,#12885,#12886,#12887,#12888,#12889,#12890,#12891,#12892,#12893,
#12894,#12895,#12896,#12897,#12898,#12899,#12900,#12901,#12902,#12903,#12904,
#12905,#12906,#12907,#12908,#12909,#12910,#12911,#12912,#12913,#12914,#12915,
#12916,#12917,#12918,#12919,#12920,#12921,#12922,#12923,#12924,#12925,#12926,
#12927,#12928,#12929,#12930,#12931,#12932,#12933,#12934,#12935),
 .UNSPECIFIED.,.F.,.F.,(4,3,3,3,3,3,3,3,3,3,3,3,3,3,3,3,3,3,3,3,3,3,3,3,
3,3,3,3,3,3,3,3,3,3,3,3,3,3,3,3,3,3,3,3,3,3,3,3,3,3,3,3,3,3,3,3,3,3,3,3,
3,3,3,4),(-49.2714534410242,-49.1553637467566,-49.0334521289365,-48.9115405111164,
-48.8091732240723,-48.7069563346426,-48.6048590377581,-48.5028265388501,
-48.4008258249242,-48.2988239253026,-48.1967177159402,-48.0945581751034,
-47.9922161387732,-47.9133458068079,-47.8109785197638,-47.7087616303339,
-47.6066643334494,-47.5046318345414,-47.4026311206155,-47.3006292209937,
-47.1985230116313,-47.0963634707945,-46.9940214344642,-46.9151511024994,
-46.8127838154554,-46.7105669260255,-46.608469629141,-46.5064371302331,
-46.4044364163071,-46.3024345166853,-46.200328307323,-46.0981687664861,
-45.9958267301559,-45.9169563981909,-45.8145891111468,-45.712372221717,
-45.6102749248325,-45.5082424259245,-45.4062417119986,-45.3042398123768,
-45.2021336030144,-45.0999740621776,-44.9976320258473,-44.9187616938824,
-44.8163944068383,-44.7141775174084,-44.612080220524,-44.510047721616,-44.40804700769,
-44.3060451080683,-44.2039388987059,-44.101779357869,-43.9994373215388,
-43.9205669895739,-43.8191696623787,-43.7153069713905,-43.6141779904582,
-43.5131096780641,-43.4120678056774,-43.3061178878761,-43.2049654936796,
-43.1037498433122,-43.0023807665007,-42.9882681344725),.UNSPECIFIED.);
#1204=B_SPLINE_CURVE_WITH_KNOTS('',3,(#12937,#12938,#12939,#12940,#12941,
#12942,#12943,#12944,#12945,#12946,#12947,#12948,#12949,#12950,#12951,#12952,
#12953,#12954,#12955,#12956,#12957,#12958,#12959,#12960,#12961,#12962,#12963,
#12964,#12965,#12966,#12967,#12968,#12969,#12970,#12971,#12972,#12973,#12974,
#12975,#12976,#12977,#12978,#12979,#12980,#12981,#12982,#12983,#12984,#12985,
#12986,#12987,#12988,#12989,#12990,#12991,#12992,#12993,#12994,#12995,#12996,
#12997,#12998,#12999,#13000,#13001,#13002,#13003,#13004,#13005,#13006,#13007,
#13008,#13009,#13010,#13011,#13012,#13013,#13014,#13015,#13016,#13017,#13018,
#13019,#13020,#13021,#13022,#13023,#13024,#13025,#13026,#13027,#13028,#13029,
#13030,#13031,#13032,#13033,#13034,#13035,#13036,#13037,#13038,#13039,#13040,
#13041,#13042,#13043,#13044,#13045,#13046,#13047,#13048,#13049,#13050,#13051,
#13052,#13053,#13054,#13055,#13056,#13057,#13058,#13059,#13060,#13061,#13062,
#13063,#13064,#13065,#13066,#13067,#13068,#13069,#13070,#13071,#13072,#13073,
#13074,#13075,#13076,#13077,#13078,#13079,#13080,#13081,#13082,#13083,#13084,
#13085,#13086,#13087,#13088,#13089,#13090,#13091,#13092,#13093,#13094,#13095,
#13096,#13097,#13098,#13099,#13100,#13101,#13102,#13103,#13104,#13105,#13106,
#13107,#13108,#13109,#13110,#13111,#13112,#13113,#13114,#13115,#13116,#13117,
#13118,#13119,#13120,#13121,#13122,#13123,#13124,#13125,#13126),
 .UNSPECIFIED.,.F.,.F.,(4,3,3,3,3,3,3,3,3,3,3,3,3,3,3,3,3,3,3,3,3,3,3,3,
3,3,3,3,3,3,3,3,3,3,3,3,3,3,3,3,3,3,3,3,3,3,3,3,3,3,3,3,3,3,3,3,3,3,3,3,
3,3,3,4),(-42.9882681340755,-42.9223722852654,-42.8200049982217,-42.7177881087921,
-42.615690811908,-42.5136583130004,-42.4116575990748,-42.3096556994534,
-42.2075494900914,-42.105389949255,-42.0030479129251,-41.9241775809569,
-41.8218102939128,-41.719593404483,-41.6174961075985,-41.5154636086904,
-41.4134628947644,-41.3114609951426,-41.2093547857802,-41.1071952449433,
-41.004853208613,-40.9259828766484,-40.8236155896043,-40.7213987001744,
-40.61930140329,-40.517268904382,-40.415268190456,-40.3132662908342,-40.2111600814718,
-40.1090005406349,-40.0066585043046,-39.92778817234,-39.825420885296,-39.7232039958661,
-39.6211066989817,-39.5190742000737,-39.4170734861478,-39.315071586526,
-39.2129653771637,-39.1108058363269,-39.0084637999966,-38.9295934680314,
-38.8272261809873,-38.7250092915574,-38.622911994673,-38.5208794957649,
-38.4188787818389,-38.316876882217,-38.2147706728546,-38.1126111320177,
-38.0102690956874,-37.9313987637229,-37.8290314766789,-37.726814587249,
-37.6247172903646,-37.5226847914566,-37.4206840775307,-37.318682177909,
-37.2165759685467,-37.1144164277098,-37.0120743913795,-36.9332040594144,
-36.7954612711504,-36.7050828268958),.UNSPECIFIED.);
#1205=B_SPLINE_CURVE_WITH_KNOTS('',3,(#13128,#13129,#13130,#13131,#13132,
#13133,#13134,#13135,#13136,#13137,#13138,#13139,#13140,#13141,#13142,#13143,
#13144,#13145,#13146,#13147,#13148,#13149,#13150,#13151,#13152,#13153,#13154,
#13155,#13156,#13157,#13158,#13159,#13160,#13161,#13162,#13163,#13164,#13165,
#13166,#13167,#13168,#13169,#13170,#13171,#13172,#13173,#13174,#13175,#13176,
#13177,#13178,#13179,#13180,#13181,#13182,#13183,#13184,#13185,#13186,#13187,
#13188,#13189,#13190,#13191,#13192,#13193,#13194,#13195,#13196,#13197,#13198,
#13199,#13200,#13201,#13202,#13203,#13204,#13205,#13206,#13207,#13208,#13209,
#13210,#13211,#13212,#13213,#13214,#13215,#13216,#13217,#13218,#13219,#13220,
#13221,#13222,#13223,#13224,#13225,#13226,#13227,#13228,#13229,#13230,#13231,
#13232,#13233,#13234,#13235,#13236,#13237,#13238,#13239,#13240,#13241,#13242,
#13243,#13244,#13245,#13246,#13247,#13248,#13249,#13250,#13251,#13252,#13253,
#13254,#13255,#13256,#13257,#13258,#13259,#13260,#13261,#13262,#13263,#13264,
#13265,#13266,#13267,#13268,#13269,#13270,#13271,#13272,#13273,#13274,#13275,
#13276,#13277,#13278,#13279,#13280,#13281,#13282,#13283,#13284,#13285,#13286,
#13287,#13288,#13289,#13290,#13291,#13292,#13293,#13294,#13295,#13296,#13297,
#13298,#13299,#13300,#13301,#13302,#13303,#13304,#13305,#13306,#13307,#13308,
#13309,#13310,#13311,#13312,#13313,#13314,#13315,#13316,#13317),
 .UNSPECIFIED.,.F.,.F.,(4,3,3,3,3,3,3,3,3,3,3,3,3,3,3,3,3,3,3,3,3,3,3,3,
3,3,3,3,3,3,3,3,3,3,3,3,3,3,3,3,3,3,3,3,3,3,3,3,3,3,3,3,3,3,3,3,3,3,3,3,
3,3,3,4),(-36.7050828266525,-36.6042885945794,-36.5035674624096,-36.4028848059392,
-36.3022060553303,-36.2014299820177,-36.1006021640577,-35.999600330535,
-35.9350093551059,-35.8326420680619,-35.7304251786319,-35.6283278817475,
-35.5262953828395,-35.4242946689136,-35.3222927692918,-35.2201865599295,
-35.1180270190926,-35.0156849827623,-34.9368146507975,-34.8344473637536,
-34.7322304743239,-34.6301331774395,-34.5281006785315,-34.4260999646055,
-34.3240980649836,-34.2219918556213,-34.1198323147845,-34.0174902784543,
-33.9386199464889,-33.836252659445,-33.7340357700152,-33.6319384731309,
-33.5299059742231,-33.4279052602974,-33.3259033606756,-33.2237971513134,
-33.1216376104767,-33.0192955741466,-32.9404252421805,-32.838057955136,
-32.7358410657059,-32.633743768821,-32.5317112699125,-32.429710555986,-32.3277086563638,
-32.225602447001,-32.1234429061638,-32.0211008698331,-31.942230537872,-31.8398632508286,
-31.7376463613988,-31.6355490645148,-31.5335165656073,-31.4315158516818,
-31.3295139520605,-31.2274077426987,-31.1252482018621,-31.0229061655323,
-30.9440358335635,-30.8374542773428,-30.7311507425934,-30.6250112048688,
-30.5190642728785,-30.4218975197163),.UNSPECIFIED.);
#1206=B_SPLINE_CURVE_WITH_KNOTS('',3,(#13319,#13320,#13321,#13322,#13323,
#13324,#13325,#13326,#13327,#13328,#13329,#13330,#13331,#13332,#13333,#13334,
#13335,#13336,#13337,#13338,#13339,#13340,#13341,#13342,#13343,#13344,#13345,
#13346,#13347,#13348,#13349,#13350,#13351,#13352,#13353,#13354,#13355,#13356,
#13357,#13358,#13359,#13360,#13361,#13362,#13363,#13364,#13365,#13366,#13367,
#13368,#13369,#13370,#13371,#13372,#13373,#13374,#13375,#13376,#13377,#13378,
#13379,#13380,#13381,#13382,#13383,#13384,#13385,#13386,#13387,#13388,#13389,
#13390,#13391,#13392,#13393,#13394,#13395,#13396,#13397,#13398,#13399,#13400,
#13401,#13402,#13403,#13404,#13405,#13406,#13407,#13408,#13409,#13410,#13411,
#13412,#13413,#13414,#13415,#13416,#13417,#13418,#13419,#13420,#13421,#13422,
#13423,#13424,#13425,#13426,#13427,#13428,#13429,#13430,#13431,#13432,#13433,
#13434,#13435,#13436,#13437,#13438,#13439,#13440,#13441,#13442,#13443,#13444,
#13445,#13446,#13447,#13448,#13449,#13450,#13451,#13452,#13453,#13454,#13455,
#13456,#13457,#13458,#13459,#13460,#13461,#13462,#13463,#13464,#13465,#13466,
#13467,#13468,#13469,#13470,#13471,#13472,#13473,#13474,#13475,#13476,#13477,
#13478,#13479,#13480,#13481,#13482,#13483,#13484,#13485,#13486,#13487,#13488,
#13489,#13490,#13491,#13492,#13493,#13494,#13495,#13496,#13497,#13498,#13499,
#13500,#13501,#13502,#13503,#13504,#13505,#13506,#13507,#13508),
 .UNSPECIFIED.,.F.,.F.,(4,3,3,3,3,3,3,3,3,3,3,3,3,3,3,3,3,3,3,3,3,3,3,3,
3,3,3,3,3,3,3,3,3,3,3,3,3,3,3,3,3,3,3,3,3,3,3,3,3,3,3,3,3,3,3,3,3,3,3,3,
3,3,3,4),(-30.4218975194729,-30.3139822064023,-30.2057128646672,-30.0972539529647,
-29.98848589277,-29.945841129255,-29.843473842207,-29.7412569527731,-29.6391596558847,
-29.5371271569728,-29.4351264430428,-29.333124543417,-29.2310183340508,
-29.12885879321,-29.026516756876,-28.9476464249465,-28.8452791379076,-28.7430622484828,
-28.6409649516034,-28.5389324527004,-28.4369317387794,-28.3349298391625,
-28.2328236298049,-28.1306640889728,-28.0283220526472,-27.949451720638,
-27.8470844335986,-27.7448675441735,-27.6427702472938,-27.5407377483907,
-27.4387370344697,-27.3367351348528,-27.2346289254954,-27.1324693846636,
-27.0301273483383,-26.9512570163295,-26.8488897292551,-26.7466728397948,
-26.64457554288,-26.5425430439417,-26.4405423299855,-26.3385404303335,-26.2364342209414,
-26.134274680075,-26.0319326437158,-25.953062312021,-25.8506950250239,-25.7484781356409,
-25.6463808388029,-25.5443483399411,-25.442347626061,-25.3403457264847,
-25.2382395171668,-25.136079976374,-25.0337379400866,-24.9548676077125,
-24.8528481833478,-24.7521697733989,-24.6515876604174,-24.5510669891891,
-24.4479782950907,-24.347434160888,-24.2430731868416,-24.1387122127952),
 .UNSPECIFIED.);
#1207=B_SPLINE_CURVE_WITH_KNOTS('',3,(#13510,#13511,#13512,#13513,#13514,
#13515,#13516,#13517,#13518,#13519,#13520,#13521,#13522,#13523,#13524,#13525,
#13526,#13527,#13528,#13529,#13530,#13531,#13532,#13533,#13534,#13535,#13536,
#13537,#13538,#13539,#13540,#13541,#13542,#13543,#13544,#13545,#13546,#13547,
#13548,#13549,#13550,#13551,#13552,#13553,#13554,#13555,#13556,#13557,#13558,
#13559,#13560,#13561,#13562,#13563,#13564,#13565,#13566,#13567,#13568,#13569,
#13570,#13571,#13572,#13573,#13574,#13575,#13576,#13577,#13578,#13579,#13580,
#13581,#13582,#13583,#13584,#13585,#13586,#13587,#13588,#13589,#13590,#13591,
#13592,#13593,#13594,#13595,#13596,#13597,#13598,#13599,#13600,#13601,#13602,
#13603,#13604,#13605,#13606,#13607,#13608,#13609,#13610,#13611,#13612,#13613,
#13614,#13615,#13616,#13617,#13618,#13619,#13620,#13621,#13622,#13623,#13624,
#13625,#13626,#13627,#13628,#13629,#13630,#13631,#13632,#13633,#13634,#13635,
#13636,#13637,#13638,#13639,#13640,#13641,#13642,#13643,#13644,#13645,#13646,
#13647,#13648,#13649,#13650,#13651,#13652,#13653,#13654,#13655,#13656,#13657,
#13658,#13659,#13660,#13661,#13662,#13663,#13664,#13665,#13666,#13667,#13668,
#13669,#13670,#13671,#13672,#13673,#13674,#13675,#13676,#13677,#13678,#13679,
#13680,#13681,#13682,#13683,#13684,#13685,#13686,#13687,#13688,#13689,#13690,
#13691,#13692,#13693,#13694,#13695,#13696,#13697,#13698,#13699),
 .UNSPECIFIED.,.F.,.F.,(4,3,3,3,3,3,3,3,3,3,3,3,3,3,3,3,3,3,3,3,3,3,3,3,
3,3,3,3,3,3,3,3,3,3,3,3,3,3,3,3,3,3,3,3,3,3,3,3,3,3,3,3,3,3,3,3,3,3,3,3,
3,3,3,4),(-24.1387122125366,-23.9846718531693,-23.956672903404,-23.8543056161328,
-23.752088726475,-23.6499914293626,-23.5479589302269,-23.4459582160735,
-23.343956316225,-23.2418501066388,-23.1396905655791,-23.0373485290305,
-22.9584781990955,-22.8561109124667,-22.7538940234513,-22.6517967269784,
-22.5497642284799,-22.4477635149608,-22.3457616157428,-22.2436554067765,
-22.1414958663321,-22.0391538303839,-21.960283494787,-21.8579162077476,
-21.7556993183269,-21.653602021458,-21.5515695225696,-21.4495688086671,
-21.3475669090727,-21.2454606997433,-21.1433011589426,-21.0409591226533,
-20.9620887904785,-20.8597215017776,-20.7575046106841,-20.6554073121339,
-20.5533748115597,-20.4513740959694,-20.3493721946875,-20.247265983683,
-20.1451064412114,-20.0427644032773,-19.96389408617,-19.8615268026831,-19.7593099168074,
-19.6572126234559,-19.5551801280662,-19.4531794176392,-19.3511775214919,
-19.2490713155426,-19.14691177809,-19.0445697450586,-18.9656993818615,-18.8633320937121,
-18.7611152032101,-18.6590179053077,-18.5569854054153,-18.4549846905396,
-18.352982790004,-18.2508765797888,-18.1487170381317,-18.0463750010433,
-17.967504677553,-17.8555269053571),.UNSPECIFIED.);
#1208=B_SPLINE_CURVE_WITH_KNOTS('',3,(#13701,#13702,#13703,#13704,#13705,
#13706,#13707,#13708,#13709,#13710,#13711,#13712,#13713,#13714,#13715,#13716,
#13717,#13718,#13719,#13720,#13721,#13722,#13723,#13724,#13725,#13726,#13727,
#13728,#13729,#13730,#13731,#13732,#13733,#13734,#13735,#13736,#13737,#13738,
#13739,#13740,#13741,#13742,#13743,#13744,#13745,#13746,#13747,#13748,#13749,
#13750,#13751,#13752,#13753,#13754,#13755,#13756,#13757,#13758,#13759,#13760,
#13761,#13762,#13763,#13764,#13765,#13766,#13767,#13768,#13769,#13770,#13771,
#13772,#13773,#13774,#13775,#13776,#13777,#13778,#13779,#13780,#13781,#13782,
#13783,#13784,#13785,#13786,#13787,#13788,#13789,#13790,#13791,#13792,#13793,
#13794,#13795,#13796,#13797,#13798,#13799,#13800,#13801,#13802,#13803,#13804,
#13805,#13806,#13807,#13808,#13809,#13810,#13811,#13812,#13813,#13814,#13815,
#13816,#13817,#13818,#13819,#13820,#13821,#13822,#13823,#13824,#13825,#13826,
#13827,#13828,#13829,#13830,#13831,#13832,#13833,#13834,#13835,#13836,#13837,
#13838,#13839,#13840,#13841,#13842,#13843,#13844,#13845,#13846,#13847,#13848,
#13849,#13850,#13851,#13852,#13853,#13854,#13855,#13856,#13857,#13858,#13859,
#13860,#13861,#13862,#13863,#13864,#13865,#13866,#13867,#13868,#13869,#13870,
#13871,#13872,#13873,#13874,#13875,#13876,#13877,#13878,#13879,#13880,#13881,
#13882,#13883,#13884,#13885,#13886,#13887,#13888,#13889,#13890),
 .UNSPECIFIED.,.F.,.F.,(4,3,3,3,3,3,3,3,3,3,3,3,3,3,3,3,3,3,3,3,3,3,3,3,
3,3,3,3,3,3,3,3,3,3,3,3,3,3,3,3,3,3,3,3,3,3,3,3,3,3,3,3,3,3,3,3,3,3,3,3,
3,3,3,4),(-17.8555269049038,-17.7545911196499,-17.6537987523961,-17.5530852258919,
-17.4524158822442,-17.3517561249875,-17.2510031448081,-17.1502034731529,
-17.0492255787679,-16.9693099732445,-16.8669427158835,-16.7647258561339,
-16.6626285887859,-16.5605961193123,-16.458595434678,-16.3565935641645,
-16.2544873834259,-16.1523278709894,-16.0499858623717,-15.971115268936,
-15.868747964328,-15.7665310575775,-15.664433743813,-15.5624012283022,-15.4604004980717,
-15.3583985824649,-15.2562923577183,-15.1541328018062,-15.0517907510743,
-14.9729205646275,-14.8705531977598,-14.7683362279927,-14.6662388503901,
-14.5642062705704,-14.4622054756551,-14.3602034950823,-14.2580972053933,
-14.1559375844495,-14.0535954692861,-13.974725860319,-13.8723588152025,
-13.7701421678431,-13.6680451121038,-13.5660128536591,-13.4640123791809,
-13.3620107176574,-13.2599047426625,-13.1577454344935,-13.0554036254108,
-12.9765311560105,-12.8741636634534,-12.7719465702381,-12.6698490730764,
-12.5678163761306,-12.4658154666658,-12.3638133742659,-12.261706977701,
-12.1595472524578,-12.057205038368,-11.978336451702,-11.865143194293,-11.7522969553209,
-11.6400318303335,-11.572341598581),.UNSPECIFIED.);
#1209=B_SPLINE_CURVE_WITH_KNOTS('',3,(#13892,#13893,#13894,#13895,#13896,
#13897,#13898,#13899,#13900,#13901,#13902,#13903,#13904,#13905,#13906,#13907,
#13908,#13909,#13910,#13911,#13912,#13913,#13914,#13915,#13916,#13917,#13918,
#13919,#13920,#13921,#13922,#13923,#13924,#13925,#13926,#13927,#13928,#13929,
#13930,#13931,#13932,#13933,#13934,#13935,#13936,#13937,#13938,#13939,#13940,
#13941,#13942,#13943,#13944,#13945,#13946,#13947,#13948,#13949,#13950,#13951,
#13952,#13953,#13954,#13955,#13956,#13957,#13958,#13959,#13960,#13961,#13962,
#13963,#13964,#13965,#13966,#13967,#13968,#13969,#13970,#13971,#13972,#13973,
#13974,#13975,#13976,#13977,#13978,#13979,#13980,#13981,#13982,#13983,#13984,
#13985,#13986,#13987,#13988,#13989,#13990,#13991,#13992,#13993,#13994,#13995,
#13996,#13997,#13998,#13999,#14000,#14001,#14002,#14003,#14004,#14005,#14006,
#14007,#14008,#14009,#14010,#14011,#14012,#14013,#14014,#14015,#14016,#14017,
#14018,#14019,#14020,#14021,#14022,#14023,#14024,#14025,#14026,#14027,#14028,
#14029,#14030,#14031,#14032,#14033,#14034,#14035,#14036,#14037,#14038,#14039,
#14040,#14041,#14042,#14043,#14044,#14045,#14046,#14047,#14048,#14049,#14050,
#14051,#14052,#14053,#14054,#14055,#14056,#14057,#14058,#14059,#14060,#14061,
#14062,#14063,#14064,#14065,#14066,#14067,#14068,#14069,#14070,#14071,#14072,
#14073,#14074,#14075,#14076,#14077,#14078,#14079,#14080,#14081),
 .UNSPECIFIED.,.F.,.F.,(4,3,3,3,3,3,3,3,3,3,3,3,3,3,3,3,3,3,3,3,3,3,3,3,
3,3,3,3,3,3,3,3,3,3,3,3,3,3,3,3,3,3,3,3,3,3,3,3,3,3,3,3,3,3,3,3,3,3,3,3,
3,3,3,4),(-11.5723415981774,-11.4687871680508,-11.3651903770408,-11.2614377882717,
-11.1576027709896,-11.0535531293269,-10.9801417473935,-10.8777763889726,
-10.7755614305822,-10.6734660592423,-10.5714354815914,-10.4694366819606,
-10.3674366869917,-10.2653323542086,-10.1631746773412,-10.0608344631842,
-9.98194704308499,-9.87957764019733,-9.77735864674374,-9.67525927317135,
-9.57322471527629,-9.47122196281362,-9.36921804787462,-9.26710987283633,
-9.16494839075294,-9.06260447502326,-8.98375233877649,-8.88138196791595,
-8.77916195956028,-8.67706150654447,-8.57502583031432,-8.47302192255833,
-8.37101681726233,-8.26890740648803,-8.16674466156689,-8.06439945351,-7.98555763446799,
-7.88320538840778,-7.78100356872168,-7.67892131341409,-7.57690383165239,
-7.47491808949712,-7.37293109529183,-7.27083958565016,-7.1686946536896,
-7.06636691157338,-6.98736293015949,-6.88497539269428,-6.78273832980578,
-6.68062106799417,-6.57856874128089,-6.47654836352991,-6.374526991071,-6.27240173750569,
-6.17022336025357,-6.06786304006514,-5.98916822585099,-5.88745971193225,
-5.78589199605195,-5.68443102714422,-5.58302740004296,-5.4816616432721,
-5.38024993235094,-5.28915629099788),.UNSPECIFIED.);
#1210=B_SPLINE_CURVE_WITH_KNOTS('',3,(#14083,#14084,#14085,#14086,#14087,
#14088,#14089,#14090,#14091,#14092,#14093,#14094,#14095,#14096,#14097,#14098,
#14099,#14100,#14101,#14102,#14103,#14104,#14105,#14106,#14107,#14108,#14109,
#14110,#14111,#14112,#14113,#14114,#14115,#14116,#14117,#14118,#14119,#14120,
#14121,#14122,#14123,#14124,#14125,#14126,#14127,#14128,#14129,#14130,#14131,
#14132,#14133,#14134,#14135,#14136,#14137,#14138,#14139,#14140,#14141,#14142,
#14143,#14144,#14145,#14146,#14147,#14148,#14149,#14150,#14151,#14152,#14153,
#14154,#14155,#14156,#14157,#14158,#14159,#14160,#14161,#14162,#14163,#14164,
#14165,#14166,#14167,#14168,#14169,#14170,#14171,#14172,#14173,#14174,#14175,
#14176,#14177,#14178,#14179),.UNSPECIFIED.,.F.,.F.,(4,3,3,3,3,3,3,3,3,3,
3,3,3,3,3,3,3,3,3,3,3,3,3,3,3,3,3,3,3,3,3,3,4),(-5.2891562906822,-5.16592202403009,
-5.0409071101405,-4.99097352154249,-4.8887207823386,-4.78661873310371,-4.68463617498642,
-4.58271830049947,-4.48083193862712,-4.37894396049634,-4.27695022114797,
-4.17490252616154,-4.07267004030852,-3.99277881723399,-3.89022667007414,
-3.78782539108402,-3.68554527959923,-3.58333102513057,-3.48114986928111,
-3.37896909715953,-3.27668767666928,-3.17435468887112,-3.0718440432757,
-2.99458411292549,-2.89325038855348,-2.79021171641803,-2.68914057287426,
-2.58812832611143,-2.48714069765389,-2.38259077610789,-2.28148996903811,
-2.175215490254,-2.06894101146989),.UNSPECIFIED.);
#1211=B_SPLINE_CURVE_WITH_KNOTS('',3,(#14180,#14181,#14182,#14183),
 .UNSPECIFIED.,.F.,.F.,(4,4),(-0.0402655477269185,0.),.UNSPECIFIED.);
#1212=B_SPLINE_CURVE_WITH_KNOTS('',3,(#14186,#14187,#14188,#14189,#14190),
 .UNSPECIFIED.,.F.,.F.,(4,1,4),(95.7927227292494,96.5575686288105,97.3893656654685),
 .UNSPECIFIED.);
#1213=B_SPLINE_CURVE_WITH_KNOTS('',3,(#14192,#14193,#14194,#14195,#14196,
#14197,#14198,#14199,#14200,#14201,#14202,#14203,#14204,#14205,#14206,#14207,
#14208,#14209,#14210,#14211,#14212,#14213,#14214,#14215,#14216,#14217,#14218,
#14219,#14220,#14221,#14222,#14223,#14224,#14225,#14226,#14227,#14228,#14229,
#14230,#14231,#14232,#14233,#14234,#14235,#14236,#14237,#14238,#14239,#14240,
#14241,#14242,#14243,#14244,#14245,#14246,#14247,#14248,#14249,#14250,#14251,
#14252,#14253,#14254,#14255,#14256,#14257,#14258,#14259,#14260,#14261,#14262,
#14263,#14264,#14265,#14266,#14267,#14268,#14269,#14270,#14271,#14272,#14273,
#14274,#14275,#14276,#14277,#14278,#14279,#14280,#14281,#14282),
 .UNSPECIFIED.,.F.,.F.,(4,3,3,3,3,3,3,3,3,3,3,3,3,3,3,3,3,3,3,3,3,3,3,3,
3,3,3,3,3,3,4),(97.3893722612835,97.555763333119,97.6636833055627,97.7749676470458,
97.8825903472849,97.9901474011131,98.0976777951607,98.2052204718533,98.3128843396892,
98.4206214009902,98.5285425318896,98.5539580374275,98.6621940121476,98.7734388533462,
98.881375737639,98.9892454584003,99.0970865171573,99.2049373691907,99.3129038037117,
99.4209404931574,99.5291543370944,99.552152741736,99.6591027660594,99.7658697883256,
99.8725354114468,99.9791400170328,100.08572389744,100.192397532104,100.299117505247,
100.406021276585,100.477768433197),.UNSPECIFIED.);
#1214=B_SPLINE_CURVE_WITH_KNOTS('',3,(#14286,#14287,#14288,#14289,#14290,
#14291,#14292,#14293,#14294,#14295,#14296,#14297,#14298,#14299,#14300,#14301,
#14302,#14303,#14304,#14305,#14306,#14307,#14308,#14309,#14310,#14311,#14312,
#14313,#14314,#14315,#14316,#14317,#14318,#14319,#14320,#14321,#14322,#14323,
#14324,#14325,#14326,#14327,#14328,#14329,#14330,#14331,#14332,#14333,#14334,
#14335,#14336,#14337),.UNSPECIFIED.,.F.,.F.,(4,3,3,3,3,3,3,3,3,3,3,3,3,
3,3,3,3,4),(97.38937254813,97.4958016639887,97.6009101902419,97.7059494886238,
97.810961292752,97.9184223383138,98.0235759129497,98.1321906939746,98.2408054749994,
98.3517561547439,98.4626616578144,98.5732387102861,98.6837093999491,98.7941056372081,
98.9053292727331,99.0157026983767,99.1273514388423,99.2390001793079),
 .UNSPECIFIED.);
#1215=B_SPLINE_CURVE_WITH_KNOTS('',3,(#14338,#14339,#14340,#14341,#14342,
#14343),.UNSPECIFIED.,.F.,.F.,(4,1,1,4),(95.7916382276144,96.2444160663824,
97.2426107706909,97.3893722612835),.UNSPECIFIED.);
#1216=B_SPLINE_CURVE_WITH_KNOTS('',3,(#14720,#14721,#14722,#14723,#14724,
#14725,#14726,#14727,#14728,#14729,#14730,#14731,#14732,#14733,#14734,#14735,
#14736,#14737,#14738,#14739,#14740,#14741,#14742,#14743,#14744,#14745,#14746,
#14747,#14748,#14749,#14750,#14751,#14752,#14753,#14754,#14755,#14756,#14757,
#14758,#14759,#14760,#14761,#14762,#14763,#14764,#14765,#14766,#14767,#14768,
#14769,#14770,#14771,#14772,#14773,#14774,#14775,#14776,#14777,#14778,#14779,
#14780,#14781,#14782,#14783,#14784,#14785,#14786,#14787,#14788,#14789,#14790,
#14791,#14792,#14793,#14794,#14795,#14796,#14797,#14798,#14799,#14800,#14801,
#14802,#14803,#14804),.UNSPECIFIED.,.F.,.F.,(4,3,3,3,3,3,3,3,3,3,3,3,3,
3,3,3,3,3,3,3,3,3,3,3,3,3,3,3,4),(0.,0.0160334974104419,0.0395642075604872,
0.0633644118114054,0.0837263817738086,0.0874470583914756,0.1106044065324,
0.133695295128406,0.156786183724411,0.165329376229777,0.169027049684205,
0.191207839298198,0.212732869185845,0.226227078758941,0.238087469390583,
0.24288151240858,0.246186438911864,0.267772589720587,0.289583909367139,
0.305496742371809,0.315196008042082,0.319047580844878,0.340135104067482,
0.359186757307379,0.366235629765007,0.370741076209788,0.390853652067263,
0.410818111358785,0.415993328865216),.UNSPECIFIED.);
#1217=B_SPLINE_CURVE_WITH_KNOTS('',3,(#14805,#14806,#14807,#14808,#14809,
#14810,#14811,#14812,#14813,#14814,#14815,#14816,#14817,#14818,#14819,#14820,
#14821,#14822,#14823,#14824,#14825,#14826,#14827,#14828,#14829,#14830,#14831,
#14832,#14833,#14834,#14835,#14836,#14837,#14838,#14839,#14840,#14841,#14842,
#14843,#14844,#14845,#14846,#14847,#14848,#14849,#14850,#14851,#14852,#14853,
#14854,#14855,#14856,#14857,#14858,#14859,#14860,#14861,#14862,#14863,#14864,
#14865,#14866,#14867,#14868,#14869,#14870,#14871,#14872,#14873,#14874,#14875,
#14876,#14877,#14878,#14879,#14880,#14881,#14882,#14883,#14884,#14885,#14886),
 .UNSPECIFIED.,.F.,.F.,(4,3,3,3,3,3,3,3,3,3,3,3,3,3,3,3,3,3,3,3,3,3,3,3,
3,3,3,4),(-0.415993328865187,-0.402901270545643,-0.382908564830427,-0.371774763313882,
-0.367435224694355,-0.346965909888549,-0.32591580828458,-0.321433315753078,
-0.315781547589586,-0.294320173377462,-0.272479432300184,-0.257298137875953,
-0.244873415404794,-0.24111480505867,-0.218638203108128,-0.211619958938312,
-0.189699687125207,-0.167779415312101,-0.162843814523672,-0.140373337321852,
-0.117486011710451,-0.0943539309779002,-0.0856507589901794,-0.0817563326016671,
-0.0580189261100361,-0.034237541284798,-0.0109647718819074,0.),
 .UNSPECIFIED.);
#1218=B_SPLINE_CURVE_WITH_KNOTS('',3,(#14888,#14889,#14890,#14891,#14892,
#14893,#14894,#14895,#14896,#14897,#14898,#14899,#14900,#14901,#14902,#14903,
#14904,#14905,#14906,#14907,#14908,#14909,#14910,#14911,#14912,#14913,#14914,
#14915,#14916,#14917,#14918,#14919,#14920,#14921,#14922,#14923,#14924,#14925,
#14926,#14927,#14928,#14929,#14930,#14931,#14932,#14933,#14934,#14935,#14936,
#14937,#14938,#14939,#14940,#14941,#14942,#14943,#14944,#14945,#14946,#14947,
#14948,#14949,#14950,#14951,#14952,#14953,#14954,#14955,#14956,#14957,#14958,
#14959,#14960,#14961,#14962,#14963,#14964,#14965,#14966,#14967,#14968,#14969,
#14970,#14971,#14972,#14973,#14974,#14975),.UNSPECIFIED.,.F.,.F.,(4,3,3,
3,3,3,3,3,3,3,3,3,3,3,3,3,3,3,3,3,3,3,3,3,3,3,3,3,3,4),(-0.410048543780163,
-0.398139186466655,-0.374410169281135,-0.362901775202635,-0.357252904496043,
-0.353226071091677,-0.329831664544852,-0.312242260164576,-0.303769719034645,
-0.299630020912383,-0.276842045830078,-0.2545146021889,-0.232670178061085,
-0.225307920334055,-0.221146019951397,-0.21755552666877,-0.195982423137004,
-0.189116736674495,-0.166997686103039,-0.146198385794381,-0.141443407849317,
-0.120014324717733,-0.0987103641924262,-0.0775869942730841,-0.0725417907976872,
-0.0680291545044378,-0.0474611904118694,-0.02724361982139,-0.00767557047989959,
0.),.UNSPECIFIED.);
#1219=B_SPLINE_CURVE_WITH_KNOTS('',3,(#15332,#15333,#15334,#15335,#15336,
#15337,#15338,#15339,#15340,#15341,#15342,#15343,#15344,#15345,#15346,#15347,
#15348,#15349,#15350,#15351,#15352,#15353,#15354,#15355,#15356,#15357,#15358,
#15359,#15360,#15361,#15362,#15363,#15364,#15365,#15366,#15367,#15368,#15369,
#15370,#15371,#15372,#15373,#15374,#15375,#15376,#15377,#15378,#15379,#15380,
#15381,#15382,#15383,#15384,#15385,#15386,#15387,#15388,#15389,#15390,#15391,
#15392,#15393,#15394,#15395,#15396,#15397,#15398,#15399,#15400,#15401,#15402,
#15403,#15404,#15405,#15406,#15407,#15408,#15409,#15410,#15411,#15412,#15413,
#15414,#15415,#15416,#15417,#15418,#15419),.UNSPECIFIED.,.F.,.F.,(4,3,3,
3,3,3,3,3,3,3,3,3,3,3,3,3,3,3,3,3,3,3,3,3,3,3,3,3,3,4),(0.,0.0130464519754968,
0.0327301024266493,0.0529569041528836,0.0626751748968586,0.0683819350422815,
0.0728898740513483,0.0937859875900613,0.115528408032434,0.137270828474807,
0.143309507195499,0.146634619759991,0.168716970862334,0.190720450818485,
0.203657142534596,0.22030049657604,0.223957438687906,0.245775764328327,
0.268053423336898,0.290759291313493,0.295289317391233,0.299519479633725,
0.303835795791196,0.327020679917298,0.350378655359791,0.356293009821619,
0.360744190415631,0.384491412449796,0.408026460803736,0.414097116159588),
 .UNSPECIFIED.);
#1422=VERTEX_POINT('',#5072);
#1423=VERTEX_POINT('',#5073);
#1424=VERTEX_POINT('',#5075);
#1425=VERTEX_POINT('',#5224);
#1426=VERTEX_POINT('',#5232);
#1427=VERTEX_POINT('',#5344);
#1428=VERTEX_POINT('',#5345);
#1429=VERTEX_POINT('',#5541);
#1430=VERTEX_POINT('',#5734);
#1431=VERTEX_POINT('',#5735);
#1432=VERTEX_POINT('',#5737);
#1433=VERTEX_POINT('',#5797);
#1434=VERTEX_POINT('',#5860);
#1435=VERTEX_POINT('',#5861);
#1436=VERTEX_POINT('',#5863);
#1437=VERTEX_POINT('',#6012);
#1438=VERTEX_POINT('',#6171);
#1439=VERTEX_POINT('',#6172);
#1440=VERTEX_POINT('',#6174);
#1441=VERTEX_POINT('',#6559);
#1442=VERTEX_POINT('',#6560);
#1443=VERTEX_POINT('',#6752);
#1444=VERTEX_POINT('',#6958);
#1445=VERTEX_POINT('',#6959);
#1446=VERTEX_POINT('',#6961);
#1447=VERTEX_POINT('',#7345);
#1448=VERTEX_POINT('',#7346);
#1449=VERTEX_POINT('',#7548);
#1450=VERTEX_POINT('',#7746);
#1451=VERTEX_POINT('',#7747);
#1452=VERTEX_POINT('',#7749);
#1453=VERTEX_POINT('',#8141);
#1454=VERTEX_POINT('',#8142);
#1455=VERTEX_POINT('',#8342);
#1456=VERTEX_POINT('',#8550);
#1457=VERTEX_POINT('',#8551);
#1458=VERTEX_POINT('',#8553);
#1459=VERTEX_POINT('',#8953);
#1460=VERTEX_POINT('',#8954);
#1461=VERTEX_POINT('',#9144);
#1462=VERTEX_POINT('',#9335);
#1463=VERTEX_POINT('',#9336);
#1464=VERTEX_POINT('',#9338);
#1465=VERTEX_POINT('',#9394);
#1466=VERTEX_POINT('',#9454);
#1467=VERTEX_POINT('',#9456);
#1468=VERTEX_POINT('',#9457);
#1469=VERTEX_POINT('',#9459);
#1470=VERTEX_POINT('',#9466);
#1471=VERTEX_POINT('',#9657);
#1472=VERTEX_POINT('',#9848);
#1473=VERTEX_POINT('',#10039);
#1474=VERTEX_POINT('',#10230);
#1475=VERTEX_POINT('',#10421);
#1476=VERTEX_POINT('',#10612);
#1477=VERTEX_POINT('',#10803);
#1478=VERTEX_POINT('',#10994);
#1479=VERTEX_POINT('',#11185);
#1480=VERTEX_POINT('',#11376);
#1481=VERTEX_POINT('',#11570);
#1482=VERTEX_POINT('',#11761);
#1483=VERTEX_POINT('',#11772);
#1484=VERTEX_POINT('',#11774);
#1485=VERTEX_POINT('',#11784);
#1486=VERTEX_POINT('',#11978);
#1487=VERTEX_POINT('',#12169);
#1488=VERTEX_POINT('',#12360);
#1489=VERTEX_POINT('',#12551);
#1490=VERTEX_POINT('',#12745);
#1491=VERTEX_POINT('',#12936);
#1492=VERTEX_POINT('',#13127);
#1493=VERTEX_POINT('',#13318);
#1494=VERTEX_POINT('',#13509);
#1495=VERTEX_POINT('',#13700);
#1496=VERTEX_POINT('',#13891);
#1497=VERTEX_POINT('',#14082);
#1498=VERTEX_POINT('',#14185);
#1499=VERTEX_POINT('',#14191);
#1500=VERTEX_POINT('',#14283);
#1501=VERTEX_POINT('',#14285);
#1502=VERTEX_POINT('',#14345);
#1503=VERTEX_POINT('',#14347);
#1504=VERTEX_POINT('',#14350);
#1505=VERTEX_POINT('',#14352);
#1506=VERTEX_POINT('',#14356);
#1507=VERTEX_POINT('',#14362);
#1508=VERTEX_POINT('',#15422);
#1509=VERTEX_POINT('',#15424);
#1510=VERTEX_POINT('',#15428);
#1511=VERTEX_POINT('',#15433);
#1512=VERTEX_POINT('',#15435);
#1513=VERTEX_POINT('',#15439);
#1514=VERTEX_POINT('',#15444);
#1515=VERTEX_POINT('',#15448);
#1516=VERTEX_POINT('',#15451);
#1517=VERTEX_POINT('',#15453);
#1518=VERTEX_POINT('',#15457);
#1519=VERTEX_POINT('',#15461);
#1520=VERTEX_POINT('',#15466);
#1521=VERTEX_POINT('',#15470);
#1522=VERTEX_POINT('',#15474);
#1523=VERTEX_POINT('',#15478);
#1524=VERTEX_POINT('',#15481);
#1525=VERTEX_POINT('',#15483);
#1526=VERTEX_POINT('',#15487);
#1527=VERTEX_POINT('',#15491);
#1528=VERTEX_POINT('',#15494);
#1529=VERTEX_POINT('',#15498);
#1530=VERTEX_POINT('',#15501);
#1531=VERTEX_POINT('',#15503);
#1815=EDGE_CURVE('',#1422,#1423,#840,.T.);
#1816=EDGE_CURVE('',#1424,#1422,#1141,.F.);
#1817=EDGE_CURVE('',#1425,#1424,#1142,.T.);
#1818=EDGE_CURVE('',#1426,#1425,#280,.T.);
#1819=EDGE_CURVE('',#1426,#1423,#1143,.T.);
#1820=EDGE_CURVE('',#1427,#1428,#841,.T.);
#1821=EDGE_CURVE('',#1422,#1427,#1144,.F.);
#1822=EDGE_CURVE('',#1423,#1429,#1145,.T.);
#1823=EDGE_CURVE('',#1429,#1428,#1146,.T.);
#1824=EDGE_CURVE('',#1430,#1431,#842,.T.);
#1825=EDGE_CURVE('',#1432,#1430,#1147,.T.);
#1826=EDGE_CURVE('',#1427,#1432,#1148,.F.);
#1827=EDGE_CURVE('',#1428,#1433,#1149,.T.);
#1828=EDGE_CURVE('',#1433,#1431,#1150,.T.);
#1829=EDGE_CURVE('',#1434,#1435,#843,.T.);
#1830=EDGE_CURVE('',#1436,#1434,#1151,.T.);
#1831=EDGE_CURVE('',#1430,#1436,#1152,.T.);
#1832=EDGE_CURVE('',#1431,#1437,#1153,.T.);
#1833=EDGE_CURVE('',#1437,#1435,#1154,.T.);
#1834=EDGE_CURVE('',#1438,#1439,#844,.T.);
#1835=EDGE_CURVE('',#1440,#1438,#1155,.F.);
#1836=EDGE_CURVE('',#1434,#1440,#1156,.T.);
#1837=EDGE_CURVE('',#1435,#1439,#1157,.T.);
#1838=EDGE_CURVE('',#1441,#1442,#845,.T.);
#1839=EDGE_CURVE('',#1438,#1441,#1158,.F.);
#1840=EDGE_CURVE('',#1439,#1443,#1159,.T.);
#1841=EDGE_CURVE('',#1443,#1442,#1160,.T.);
#1842=EDGE_CURVE('',#1444,#1445,#846,.T.);
#1843=EDGE_CURVE('',#1446,#1444,#1161,.F.);
#1844=EDGE_CURVE('',#1441,#1446,#1162,.F.);
#1845=EDGE_CURVE('',#1442,#1445,#1163,.T.);
#1846=EDGE_CURVE('',#1447,#1448,#847,.T.);
#1847=EDGE_CURVE('',#1444,#1447,#1164,.F.);
#1848=EDGE_CURVE('',#1445,#1449,#1165,.T.);
#1849=EDGE_CURVE('',#1449,#1448,#1166,.T.);
#1850=EDGE_CURVE('',#1450,#1451,#848,.T.);
#1851=EDGE_CURVE('',#1452,#1450,#1167,.F.);
#1852=EDGE_CURVE('',#1447,#1452,#1168,.F.);
#1853=EDGE_CURVE('',#1448,#1451,#1169,.T.);
#1854=EDGE_CURVE('',#1453,#1454,#849,.T.);
#1855=EDGE_CURVE('',#1450,#1453,#1170,.F.);
#1856=EDGE_CURVE('',#1451,#1455,#1171,.T.);
#1857=EDGE_CURVE('',#1455,#1454,#1172,.T.);
#1858=EDGE_CURVE('',#1456,#1457,#850,.T.);
#1859=EDGE_CURVE('',#1458,#1456,#1173,.F.);
#1860=EDGE_CURVE('',#1453,#1458,#1174,.F.);
#1861=EDGE_CURVE('',#1454,#1457,#1175,.T.);
#1862=EDGE_CURVE('',#1459,#1460,#851,.T.);
#1863=EDGE_CURVE('',#1456,#1459,#1176,.F.);
#1864=EDGE_CURVE('',#1457,#1461,#1177,.T.);
#1865=EDGE_CURVE('',#1461,#1460,#1178,.T.);
#1866=EDGE_CURVE('',#1462,#1463,#852,.T.);
#1867=EDGE_CURVE('',#1464,#1462,#1179,.T.);
#1868=EDGE_CURVE('',#1459,#1464,#1180,.F.);
#1869=EDGE_CURVE('',#1460,#1465,#1181,.T.);
#1870=EDGE_CURVE('',#1465,#1463,#1182,.T.);
#1871=EDGE_CURVE('',#1466,#1466,#281,.F.);
#1872=EDGE_CURVE('',#1467,#1468,#282,.T.);
#1873=EDGE_CURVE('',#1468,#1469,#1183,.T.);
#1874=EDGE_CURVE('',#1469,#1470,#1184,.T.);
#1875=EDGE_CURVE('',#1470,#1471,#1185,.T.);
#1876=EDGE_CURVE('',#1471,#1472,#1186,.T.);
#1877=EDGE_CURVE('',#1472,#1473,#1187,.T.);
#1878=EDGE_CURVE('',#1473,#1474,#1188,.T.);
#1879=EDGE_CURVE('',#1474,#1475,#1189,.T.);
#1880=EDGE_CURVE('',#1475,#1476,#1190,.T.);
#1881=EDGE_CURVE('',#1476,#1477,#1191,.T.);
#1882=EDGE_CURVE('',#1477,#1478,#1192,.T.);
#1883=EDGE_CURVE('',#1478,#1479,#1193,.T.);
#1884=EDGE_CURVE('',#1479,#1480,#1194,.T.);
#1885=EDGE_CURVE('',#1480,#1481,#1195,.T.);
#1886=EDGE_CURVE('',#1481,#1482,#1196,.T.);
#1887=EDGE_CURVE('',#1483,#1482,#283,.F.);
#1888=EDGE_CURVE('',#1483,#1484,#1197,.T.);
#1889=EDGE_CURVE('',#1484,#1485,#1198,.T.);
#1890=EDGE_CURVE('',#1485,#1486,#1199,.T.);
#1891=EDGE_CURVE('',#1486,#1487,#1200,.T.);
#1892=EDGE_CURVE('',#1487,#1488,#1201,.T.);
#1893=EDGE_CURVE('',#1488,#1489,#1202,.T.);
#1894=EDGE_CURVE('',#1489,#1490,#1203,.T.);
#1895=EDGE_CURVE('',#1490,#1491,#1204,.T.);
#1896=EDGE_CURVE('',#1491,#1492,#1205,.T.);
#1897=EDGE_CURVE('',#1492,#1493,#1206,.T.);
#1898=EDGE_CURVE('',#1493,#1494,#1207,.T.);
#1899=EDGE_CURVE('',#1494,#1495,#1208,.T.);
#1900=EDGE_CURVE('',#1495,#1496,#1209,.T.);
#1901=EDGE_CURVE('',#1496,#1497,#1210,.T.);
#1902=EDGE_CURVE('',#1497,#1467,#1211,.T.);
#1903=EDGE_CURVE('',#1463,#1498,#1212,.T.);
#1904=EDGE_CURVE('',#1498,#1499,#1213,.T.);
#1905=EDGE_CURVE('',#1500,#1499,#284,.T.);
#1906=EDGE_CURVE('',#1501,#1500,#1214,.T.);
#1907=EDGE_CURVE('',#1462,#1501,#1215,.T.);
#1908=EDGE_CURVE('',#1502,#1502,#285,.T.);
#1909=EDGE_CURVE('',#1503,#1503,#286,.T.);
#1910=EDGE_CURVE('',#1504,#1504,#287,.T.);
#1911=EDGE_CURVE('',#1504,#1505,#288,.T.);
#1912=EDGE_CURVE('',#1505,#1505,#289,.T.);
#1913=EDGE_CURVE('',#1505,#1506,#853,.T.);
#1914=EDGE_CURVE('',#1506,#1506,#290,.T.);
#1915=EDGE_CURVE('',#1506,#1502,#291,.T.);
#1916=EDGE_CURVE('',#1507,#1507,#292,.T.);
#1917=EDGE_CURVE('',#1482,#1500,#1216,.T.);
#1918=EDGE_CURVE('',#1425,#1468,#1217,.T.);
#1919=EDGE_CURVE('',#1467,#1426,#1218,.T.);
#1920=EDGE_CURVE('',#1499,#1483,#1219,.T.);
#1921=EDGE_CURVE('',#1508,#1508,#293,.T.);
#1922=EDGE_CURVE('',#1508,#1509,#294,.T.);
#1923=EDGE_CURVE('',#1509,#1509,#295,.T.);
#1924=EDGE_CURVE('',#1509,#1510,#854,.T.);
#1925=EDGE_CURVE('',#1510,#1510,#296,.T.);
#1926=EDGE_CURVE('',#1511,#1511,#297,.T.);
#1927=EDGE_CURVE('',#1511,#1512,#298,.T.);
#1928=EDGE_CURVE('',#1512,#1512,#299,.T.);
#1929=EDGE_CURVE('',#1512,#1513,#855,.T.);
#1930=EDGE_CURVE('',#1513,#1513,#300,.T.);
#1931=EDGE_CURVE('',#1513,#1514,#301,.T.);
#1932=EDGE_CURVE('',#1514,#1514,#302,.T.);
#1933=EDGE_CURVE('',#1515,#1515,#303,.T.);
#1934=EDGE_CURVE('',#1516,#1516,#304,.T.);
#1935=EDGE_CURVE('',#1516,#1517,#305,.T.);
#1936=EDGE_CURVE('',#1517,#1517,#306,.T.);
#1937=EDGE_CURVE('',#1517,#1518,#856,.T.);
#1938=EDGE_CURVE('',#1518,#1518,#307,.T.);
#1939=EDGE_CURVE('',#1519,#1519,#308,.T.);
#1940=EDGE_CURVE('',#1518,#1507,#309,.T.);
#1941=EDGE_CURVE('',#1503,#1520,#310,.T.);
#1942=EDGE_CURVE('',#1520,#1520,#311,.T.);
#1943=EDGE_CURVE('',#1520,#1521,#857,.T.);
#1944=EDGE_CURVE('',#1521,#1521,#312,.T.);
#1945=EDGE_CURVE('',#1521,#1522,#313,.T.);
#1946=EDGE_CURVE('',#1522,#1522,#314,.T.);
#1947=EDGE_CURVE('',#1523,#1523,#315,.T.);
#1948=EDGE_CURVE('',#1524,#1524,#316,.T.);
#1949=EDGE_CURVE('',#1524,#1525,#317,.T.);
#1950=EDGE_CURVE('',#1525,#1525,#318,.T.);
#1951=EDGE_CURVE('',#1525,#1526,#858,.T.);
#1952=EDGE_CURVE('',#1526,#1526,#319,.T.);
#1953=EDGE_CURVE('',#1527,#1527,#320,.T.);
#1954=EDGE_CURVE('',#1526,#1528,#321,.T.);
#1955=EDGE_CURVE('',#1528,#1528,#322,.T.);
#1956=EDGE_CURVE('',#1529,#1529,#323,.T.);
#1957=EDGE_CURVE('',#1530,#1530,#324,.T.);
#1958=EDGE_CURVE('',#1530,#1531,#325,.T.);
#1959=EDGE_CURVE('',#1531,#1531,#326,.T.);
#1960=EDGE_CURVE('',#1529,#1530,#859,.T.);
#1961=EDGE_CURVE('',#1523,#1527,#860,.T.);
#1962=EDGE_CURVE('',#1515,#1519,#861,.T.);
#2404=ORIENTED_EDGE('',*,*,#1815,.F.);
#2405=ORIENTED_EDGE('',*,*,#1816,.F.);
#2406=ORIENTED_EDGE('',*,*,#1817,.F.);
#2407=ORIENTED_EDGE('',*,*,#1818,.F.);
#2408=ORIENTED_EDGE('',*,*,#1819,.T.);
#2409=ORIENTED_EDGE('',*,*,#1820,.F.);
#2410=ORIENTED_EDGE('',*,*,#1821,.F.);
#2411=ORIENTED_EDGE('',*,*,#1815,.T.);
#2412=ORIENTED_EDGE('',*,*,#1822,.T.);
#2413=ORIENTED_EDGE('',*,*,#1823,.T.);
#2414=ORIENTED_EDGE('',*,*,#1824,.F.);
#2415=ORIENTED_EDGE('',*,*,#1825,.F.);
#2416=ORIENTED_EDGE('',*,*,#1826,.F.);
#2417=ORIENTED_EDGE('',*,*,#1820,.T.);
#2418=ORIENTED_EDGE('',*,*,#1827,.T.);
#2419=ORIENTED_EDGE('',*,*,#1828,.T.);
#2420=ORIENTED_EDGE('',*,*,#1829,.F.);
#2421=ORIENTED_EDGE('',*,*,#1830,.F.);
#2422=ORIENTED_EDGE('',*,*,#1831,.F.);
#2423=ORIENTED_EDGE('',*,*,#1824,.T.);
#2424=ORIENTED_EDGE('',*,*,#1832,.T.);
#2425=ORIENTED_EDGE('',*,*,#1833,.T.);
#2426=ORIENTED_EDGE('',*,*,#1834,.F.);
#2427=ORIENTED_EDGE('',*,*,#1835,.F.);
#2428=ORIENTED_EDGE('',*,*,#1836,.F.);
#2429=ORIENTED_EDGE('',*,*,#1829,.T.);
#2430=ORIENTED_EDGE('',*,*,#1837,.T.);
#2431=ORIENTED_EDGE('',*,*,#1838,.F.);
#2432=ORIENTED_EDGE('',*,*,#1839,.F.);
#2433=ORIENTED_EDGE('',*,*,#1834,.T.);
#2434=ORIENTED_EDGE('',*,*,#1840,.T.);
#2435=ORIENTED_EDGE('',*,*,#1841,.T.);
#2436=ORIENTED_EDGE('',*,*,#1842,.F.);
#2437=ORIENTED_EDGE('',*,*,#1843,.F.);
#2438=ORIENTED_EDGE('',*,*,#1844,.F.);
#2439=ORIENTED_EDGE('',*,*,#1838,.T.);
#2440=ORIENTED_EDGE('',*,*,#1845,.T.);
#2441=ORIENTED_EDGE('',*,*,#1846,.F.);
#2442=ORIENTED_EDGE('',*,*,#1847,.F.);
#2443=ORIENTED_EDGE('',*,*,#1842,.T.);
#2444=ORIENTED_EDGE('',*,*,#1848,.T.);
#2445=ORIENTED_EDGE('',*,*,#1849,.T.);
#2446=ORIENTED_EDGE('',*,*,#1850,.F.);
#2447=ORIENTED_EDGE('',*,*,#1851,.F.);
#2448=ORIENTED_EDGE('',*,*,#1852,.F.);
#2449=ORIENTED_EDGE('',*,*,#1846,.T.);
#2450=ORIENTED_EDGE('',*,*,#1853,.T.);
#2451=ORIENTED_EDGE('',*,*,#1854,.F.);
#2452=ORIENTED_EDGE('',*,*,#1855,.F.);
#2453=ORIENTED_EDGE('',*,*,#1850,.T.);
#2454=ORIENTED_EDGE('',*,*,#1856,.T.);
#2455=ORIENTED_EDGE('',*,*,#1857,.T.);
#2456=ORIENTED_EDGE('',*,*,#1858,.F.);
#2457=ORIENTED_EDGE('',*,*,#1859,.F.);
#2458=ORIENTED_EDGE('',*,*,#1860,.F.);
#2459=ORIENTED_EDGE('',*,*,#1854,.T.);
#2460=ORIENTED_EDGE('',*,*,#1861,.T.);
#2461=ORIENTED_EDGE('',*,*,#1862,.F.);
#2462=ORIENTED_EDGE('',*,*,#1863,.F.);
#2463=ORIENTED_EDGE('',*,*,#1858,.T.);
#2464=ORIENTED_EDGE('',*,*,#1864,.T.);
#2465=ORIENTED_EDGE('',*,*,#1865,.T.);
#2466=ORIENTED_EDGE('',*,*,#1866,.F.);
#2467=ORIENTED_EDGE('',*,*,#1867,.F.);
#2468=ORIENTED_EDGE('',*,*,#1868,.F.);
#2469=ORIENTED_EDGE('',*,*,#1862,.T.);
#2470=ORIENTED_EDGE('',*,*,#1869,.T.);
#2471=ORIENTED_EDGE('',*,*,#1870,.T.);
#2472=ORIENTED_EDGE('',*,*,#1871,.T.);
#2473=ORIENTED_EDGE('',*,*,#1872,.T.);
#2474=ORIENTED_EDGE('',*,*,#1873,.T.);
#2475=ORIENTED_EDGE('',*,*,#1874,.T.);
#2476=ORIENTED_EDGE('',*,*,#1875,.T.);
#2477=ORIENTED_EDGE('',*,*,#1876,.T.);
#2478=ORIENTED_EDGE('',*,*,#1877,.T.);
#2479=ORIENTED_EDGE('',*,*,#1878,.T.);
#2480=ORIENTED_EDGE('',*,*,#1879,.T.);
#2481=ORIENTED_EDGE('',*,*,#1880,.T.);
#2482=ORIENTED_EDGE('',*,*,#1881,.T.);
#2483=ORIENTED_EDGE('',*,*,#1882,.T.);
#2484=ORIENTED_EDGE('',*,*,#1883,.T.);
#2485=ORIENTED_EDGE('',*,*,#1884,.T.);
#2486=ORIENTED_EDGE('',*,*,#1885,.T.);
#2487=ORIENTED_EDGE('',*,*,#1886,.T.);
#2488=ORIENTED_EDGE('',*,*,#1887,.F.);
#2489=ORIENTED_EDGE('',*,*,#1888,.T.);
#2490=ORIENTED_EDGE('',*,*,#1889,.T.);
#2491=ORIENTED_EDGE('',*,*,#1890,.T.);
#2492=ORIENTED_EDGE('',*,*,#1891,.T.);
#2493=ORIENTED_EDGE('',*,*,#1892,.T.);
#2494=ORIENTED_EDGE('',*,*,#1893,.T.);
#2495=ORIENTED_EDGE('',*,*,#1894,.T.);
#2496=ORIENTED_EDGE('',*,*,#1895,.T.);
#2497=ORIENTED_EDGE('',*,*,#1896,.T.);
#2498=ORIENTED_EDGE('',*,*,#1897,.T.);
#2499=ORIENTED_EDGE('',*,*,#1898,.T.);
#2500=ORIENTED_EDGE('',*,*,#1899,.T.);
#2501=ORIENTED_EDGE('',*,*,#1900,.T.);
#2502=ORIENTED_EDGE('',*,*,#1901,.T.);
#2503=ORIENTED_EDGE('',*,*,#1902,.T.);
#2504=ORIENTED_EDGE('',*,*,#1866,.T.);
#2505=ORIENTED_EDGE('',*,*,#1903,.T.);
#2506=ORIENTED_EDGE('',*,*,#1904,.T.);
#2507=ORIENTED_EDGE('',*,*,#1905,.F.);
#2508=ORIENTED_EDGE('',*,*,#1906,.F.);
#2509=ORIENTED_EDGE('',*,*,#1907,.F.);
#2510=ORIENTED_EDGE('',*,*,#1908,.F.);
#2511=ORIENTED_EDGE('',*,*,#1909,.F.);
#2512=ORIENTED_EDGE('',*,*,#1910,.T.);
#2513=ORIENTED_EDGE('',*,*,#1911,.T.);
#2514=ORIENTED_EDGE('',*,*,#1912,.T.);
#2515=ORIENTED_EDGE('',*,*,#1911,.F.);
#2516=ORIENTED_EDGE('',*,*,#1912,.F.);
#2517=ORIENTED_EDGE('',*,*,#1913,.T.);
#2518=ORIENTED_EDGE('',*,*,#1914,.F.);
#2519=ORIENTED_EDGE('',*,*,#1913,.F.);
#2520=ORIENTED_EDGE('',*,*,#1914,.T.);
#2521=ORIENTED_EDGE('',*,*,#1915,.T.);
#2522=ORIENTED_EDGE('',*,*,#1908,.T.);
#2523=ORIENTED_EDGE('',*,*,#1915,.F.);
#2524=ORIENTED_EDGE('',*,*,#1916,.F.);
#2525=ORIENTED_EDGE('',*,*,#1910,.F.);
#2526=ORIENTED_EDGE('',*,*,#1917,.F.);
#2527=ORIENTED_EDGE('',*,*,#1886,.F.);
#2528=ORIENTED_EDGE('',*,*,#1885,.F.);
#2529=ORIENTED_EDGE('',*,*,#1884,.F.);
#2530=ORIENTED_EDGE('',*,*,#1883,.F.);
#2531=ORIENTED_EDGE('',*,*,#1882,.F.);
#2532=ORIENTED_EDGE('',*,*,#1881,.F.);
#2533=ORIENTED_EDGE('',*,*,#1880,.F.);
#2534=ORIENTED_EDGE('',*,*,#1879,.F.);
#2535=ORIENTED_EDGE('',*,*,#1878,.F.);
#2536=ORIENTED_EDGE('',*,*,#1877,.F.);
#2537=ORIENTED_EDGE('',*,*,#1876,.F.);
#2538=ORIENTED_EDGE('',*,*,#1875,.F.);
#2539=ORIENTED_EDGE('',*,*,#1874,.F.);
#2540=ORIENTED_EDGE('',*,*,#1873,.F.);
#2541=ORIENTED_EDGE('',*,*,#1918,.F.);
#2542=ORIENTED_EDGE('',*,*,#1817,.T.);
#2543=ORIENTED_EDGE('',*,*,#1816,.T.);
#2544=ORIENTED_EDGE('',*,*,#1821,.T.);
#2545=ORIENTED_EDGE('',*,*,#1826,.T.);
#2546=ORIENTED_EDGE('',*,*,#1825,.T.);
#2547=ORIENTED_EDGE('',*,*,#1831,.T.);
#2548=ORIENTED_EDGE('',*,*,#1830,.T.);
#2549=ORIENTED_EDGE('',*,*,#1836,.T.);
#2550=ORIENTED_EDGE('',*,*,#1835,.T.);
#2551=ORIENTED_EDGE('',*,*,#1839,.T.);
#2552=ORIENTED_EDGE('',*,*,#1844,.T.);
#2553=ORIENTED_EDGE('',*,*,#1843,.T.);
#2554=ORIENTED_EDGE('',*,*,#1847,.T.);
#2555=ORIENTED_EDGE('',*,*,#1852,.T.);
#2556=ORIENTED_EDGE('',*,*,#1851,.T.);
#2557=ORIENTED_EDGE('',*,*,#1855,.T.);
#2558=ORIENTED_EDGE('',*,*,#1860,.T.);
#2559=ORIENTED_EDGE('',*,*,#1859,.T.);
#2560=ORIENTED_EDGE('',*,*,#1863,.T.);
#2561=ORIENTED_EDGE('',*,*,#1868,.T.);
#2562=ORIENTED_EDGE('',*,*,#1867,.T.);
#2563=ORIENTED_EDGE('',*,*,#1907,.T.);
#2564=ORIENTED_EDGE('',*,*,#1906,.T.);
#2565=ORIENTED_EDGE('',*,*,#1872,.F.);
#2566=ORIENTED_EDGE('',*,*,#1919,.T.);
#2567=ORIENTED_EDGE('',*,*,#1818,.T.);
#2568=ORIENTED_EDGE('',*,*,#1918,.T.);
#2569=ORIENTED_EDGE('',*,*,#1920,.F.);
#2570=ORIENTED_EDGE('',*,*,#1904,.F.);
#2571=ORIENTED_EDGE('',*,*,#1903,.F.);
#2572=ORIENTED_EDGE('',*,*,#1870,.F.);
#2573=ORIENTED_EDGE('',*,*,#1869,.F.);
#2574=ORIENTED_EDGE('',*,*,#1865,.F.);
#2575=ORIENTED_EDGE('',*,*,#1864,.F.);
#2576=ORIENTED_EDGE('',*,*,#1861,.F.);
#2577=ORIENTED_EDGE('',*,*,#1857,.F.);
#2578=ORIENTED_EDGE('',*,*,#1856,.F.);
#2579=ORIENTED_EDGE('',*,*,#1853,.F.);
#2580=ORIENTED_EDGE('',*,*,#1849,.F.);
#2581=ORIENTED_EDGE('',*,*,#1848,.F.);
#2582=ORIENTED_EDGE('',*,*,#1845,.F.);
#2583=ORIENTED_EDGE('',*,*,#1841,.F.);
#2584=ORIENTED_EDGE('',*,*,#1840,.F.);
#2585=ORIENTED_EDGE('',*,*,#1837,.F.);
#2586=ORIENTED_EDGE('',*,*,#1833,.F.);
#2587=ORIENTED_EDGE('',*,*,#1832,.F.);
#2588=ORIENTED_EDGE('',*,*,#1828,.F.);
#2589=ORIENTED_EDGE('',*,*,#1827,.F.);
#2590=ORIENTED_EDGE('',*,*,#1823,.F.);
#2591=ORIENTED_EDGE('',*,*,#1822,.F.);
#2592=ORIENTED_EDGE('',*,*,#1819,.F.);
#2593=ORIENTED_EDGE('',*,*,#1919,.F.);
#2594=ORIENTED_EDGE('',*,*,#1902,.F.);
#2595=ORIENTED_EDGE('',*,*,#1901,.F.);
#2596=ORIENTED_EDGE('',*,*,#1900,.F.);
#2597=ORIENTED_EDGE('',*,*,#1899,.F.);
#2598=ORIENTED_EDGE('',*,*,#1898,.F.);
#2599=ORIENTED_EDGE('',*,*,#1897,.F.);
#2600=ORIENTED_EDGE('',*,*,#1896,.F.);
#2601=ORIENTED_EDGE('',*,*,#1895,.F.);
#2602=ORIENTED_EDGE('',*,*,#1894,.F.);
#2603=ORIENTED_EDGE('',*,*,#1893,.F.);
#2604=ORIENTED_EDGE('',*,*,#1892,.F.);
#2605=ORIENTED_EDGE('',*,*,#1891,.F.);
#2606=ORIENTED_EDGE('',*,*,#1890,.F.);
#2607=ORIENTED_EDGE('',*,*,#1889,.F.);
#2608=ORIENTED_EDGE('',*,*,#1888,.F.);
#2609=ORIENTED_EDGE('',*,*,#1917,.T.);
#2610=ORIENTED_EDGE('',*,*,#1905,.T.);
#2611=ORIENTED_EDGE('',*,*,#1920,.T.);
#2612=ORIENTED_EDGE('',*,*,#1887,.T.);
#2613=ORIENTED_EDGE('',*,*,#1921,.T.);
#2614=ORIENTED_EDGE('',*,*,#1922,.T.);
#2615=ORIENTED_EDGE('',*,*,#1923,.T.);
#2616=ORIENTED_EDGE('',*,*,#1922,.F.);
#2617=ORIENTED_EDGE('',*,*,#1923,.F.);
#2618=ORIENTED_EDGE('',*,*,#1924,.T.);
#2619=ORIENTED_EDGE('',*,*,#1925,.T.);
#2620=ORIENTED_EDGE('',*,*,#1924,.F.);
#2621=ORIENTED_EDGE('',*,*,#1921,.F.);
#2622=ORIENTED_EDGE('',*,*,#1871,.F.);
#2623=ORIENTED_EDGE('',*,*,#1926,.T.);
#2624=ORIENTED_EDGE('',*,*,#1927,.T.);
#2625=ORIENTED_EDGE('',*,*,#1928,.T.);
#2626=ORIENTED_EDGE('',*,*,#1927,.F.);
#2627=ORIENTED_EDGE('',*,*,#1928,.F.);
#2628=ORIENTED_EDGE('',*,*,#1929,.T.);
#2629=ORIENTED_EDGE('',*,*,#1930,.F.);
#2630=ORIENTED_EDGE('',*,*,#1929,.F.);
#2631=ORIENTED_EDGE('',*,*,#1926,.F.);
#2632=ORIENTED_EDGE('',*,*,#1925,.F.);
#2633=ORIENTED_EDGE('',*,*,#1930,.T.);
#2634=ORIENTED_EDGE('',*,*,#1931,.T.);
#2635=ORIENTED_EDGE('',*,*,#1932,.T.);
#2636=ORIENTED_EDGE('',*,*,#1931,.F.);
#2637=ORIENTED_EDGE('',*,*,#1932,.F.);
#2638=ORIENTED_EDGE('',*,*,#1933,.T.);
#2639=ORIENTED_EDGE('',*,*,#1934,.T.);
#2640=ORIENTED_EDGE('',*,*,#1935,.T.);
#2641=ORIENTED_EDGE('',*,*,#1936,.T.);
#2642=ORIENTED_EDGE('',*,*,#1935,.F.);
#2643=ORIENTED_EDGE('',*,*,#1936,.F.);
#2644=ORIENTED_EDGE('',*,*,#1937,.T.);
#2645=ORIENTED_EDGE('',*,*,#1938,.F.);
#2646=ORIENTED_EDGE('',*,*,#1937,.F.);
#2647=ORIENTED_EDGE('',*,*,#1934,.F.);
#2648=ORIENTED_EDGE('',*,*,#1939,.F.);
#2649=ORIENTED_EDGE('',*,*,#1938,.T.);
#2650=ORIENTED_EDGE('',*,*,#1940,.T.);
#2651=ORIENTED_EDGE('',*,*,#1916,.T.);
#2652=ORIENTED_EDGE('',*,*,#1940,.F.);
#2653=ORIENTED_EDGE('',*,*,#1909,.T.);
#2654=ORIENTED_EDGE('',*,*,#1941,.T.);
#2655=ORIENTED_EDGE('',*,*,#1942,.T.);
#2656=ORIENTED_EDGE('',*,*,#1941,.F.);
#2657=ORIENTED_EDGE('',*,*,#1942,.F.);
#2658=ORIENTED_EDGE('',*,*,#1943,.T.);
#2659=ORIENTED_EDGE('',*,*,#1944,.F.);
#2660=ORIENTED_EDGE('',*,*,#1943,.F.);
#2661=ORIENTED_EDGE('',*,*,#1944,.T.);
#2662=ORIENTED_EDGE('',*,*,#1945,.T.);
#2663=ORIENTED_EDGE('',*,*,#1946,.T.);
#2664=ORIENTED_EDGE('',*,*,#1945,.F.);
#2665=ORIENTED_EDGE('',*,*,#1946,.F.);
#2666=ORIENTED_EDGE('',*,*,#1947,.T.);
#2667=ORIENTED_EDGE('',*,*,#1948,.T.);
#2668=ORIENTED_EDGE('',*,*,#1949,.T.);
#2669=ORIENTED_EDGE('',*,*,#1950,.T.);
#2670=ORIENTED_EDGE('',*,*,#1949,.F.);
#2671=ORIENTED_EDGE('',*,*,#1950,.F.);
#2672=ORIENTED_EDGE('',*,*,#1951,.T.);
#2673=ORIENTED_EDGE('',*,*,#1952,.F.);
#2674=ORIENTED_EDGE('',*,*,#1951,.F.);
#2675=ORIENTED_EDGE('',*,*,#1948,.F.);
#2676=ORIENTED_EDGE('',*,*,#1953,.F.);
#2677=ORIENTED_EDGE('',*,*,#1952,.T.);
#2678=ORIENTED_EDGE('',*,*,#1954,.T.);
#2679=ORIENTED_EDGE('',*,*,#1955,.T.);
#2680=ORIENTED_EDGE('',*,*,#1954,.F.);
#2681=ORIENTED_EDGE('',*,*,#1955,.F.);
#2682=ORIENTED_EDGE('',*,*,#1956,.T.);
#2683=ORIENTED_EDGE('',*,*,#1957,.T.);
#2684=ORIENTED_EDGE('',*,*,#1958,.T.);
#2685=ORIENTED_EDGE('',*,*,#1959,.T.);
#2686=ORIENTED_EDGE('',*,*,#1958,.F.);
#2687=ORIENTED_EDGE('',*,*,#1959,.F.);
#2688=ORIENTED_EDGE('',*,*,#1956,.F.);
#2689=ORIENTED_EDGE('',*,*,#1960,.T.);
#2690=ORIENTED_EDGE('',*,*,#1957,.F.);
#2691=ORIENTED_EDGE('',*,*,#1960,.F.);
#2692=ORIENTED_EDGE('',*,*,#1947,.F.);
#2693=ORIENTED_EDGE('',*,*,#1961,.T.);
#2694=ORIENTED_EDGE('',*,*,#1953,.T.);
#2695=ORIENTED_EDGE('',*,*,#1961,.F.);
#2696=ORIENTED_EDGE('',*,*,#1933,.F.);
#2697=ORIENTED_EDGE('',*,*,#1962,.T.);
#2698=ORIENTED_EDGE('',*,*,#1939,.T.);
#2699=ORIENTED_EDGE('',*,*,#1962,.F.);
#3404=CYLINDRICAL_SURFACE('',#3852,1.77625);
#3405=CYLINDRICAL_SURFACE('',#3854,1.77625);
#3406=CYLINDRICAL_SURFACE('',#3855,1.77625);
#3407=CYLINDRICAL_SURFACE('',#3856,1.77625);
#3408=CYLINDRICAL_SURFACE('',#3857,1.77625);
#3409=CYLINDRICAL_SURFACE('',#3858,1.77625);
#3410=CYLINDRICAL_SURFACE('',#3859,1.77625);
#3411=CYLINDRICAL_SURFACE('',#3860,1.77625);
#3412=CYLINDRICAL_SURFACE('',#3861,1.77625);
#3413=CYLINDRICAL_SURFACE('',#3862,1.77625);
#3414=CYLINDRICAL_SURFACE('',#3863,1.77625);
#3415=CYLINDRICAL_SURFACE('',#3864,1.77625);
#3416=CYLINDRICAL_SURFACE('',#3865,1.77625);
#3417=CYLINDRICAL_SURFACE('',#3866,2.204);
#3418=CYLINDRICAL_SURFACE('',#3870,1.77625);
#3419=CYLINDRICAL_SURFACE('',#3891,4.48902817623056);
#3420=CYLINDRICAL_SURFACE('',#3944,4.42329516333974);
#3421=CYLINDRICAL_SURFACE('',#3945,2.21164758166987);
#3422=CYLINDRICAL_SURFACE('',#3946,2.21164758166987);
#3496=ADVANCED_FACE('',(#404),#3404,.T.);
#3497=ADVANCED_FACE('',(#405),#3405,.T.);
#3498=ADVANCED_FACE('',(#406),#3406,.T.);
#3499=ADVANCED_FACE('',(#407),#3407,.T.);
#3500=ADVANCED_FACE('',(#408),#3408,.T.);
#3501=ADVANCED_FACE('',(#409),#3409,.T.);
#3502=ADVANCED_FACE('',(#410),#3410,.T.);
#3503=ADVANCED_FACE('',(#411),#3411,.T.);
#3504=ADVANCED_FACE('',(#412),#3412,.T.);
#3505=ADVANCED_FACE('',(#413),#3413,.T.);
#3506=ADVANCED_FACE('',(#414),#3414,.T.);
#3507=ADVANCED_FACE('',(#415),#3415,.T.);
#3508=ADVANCED_FACE('',(#416),#3416,.T.);
#3509=ADVANCED_FACE('',(#417,#181),#3417,.T.);
#3510=ADVANCED_FACE('',(#418),#3418,.T.);
#3511=ADVANCED_FACE('',(#419,#182),#209,.T.);
#3512=ADVANCED_FACE('',(#420),#98,.T.);
#3513=ADVANCED_FACE('',(#421),#164,.T.);
#3514=ADVANCED_FACE('',(#422),#99,.T.);
#3515=ADVANCED_FACE('',(#423,#183),#210,.T.);
#3516=ADVANCED_FACE('',(#424),#58,.F.);
#3517=ADVANCED_FACE('',(#425),#211,.T.);
#3518=ADVANCED_FACE('',(#426),#59,.F.);
#3519=ADVANCED_FACE('',(#427),#212,.T.);
#3520=ADVANCED_FACE('',(#428),#100,.T.);
#3521=ADVANCED_FACE('',(#429),#3419,.T.);
#3522=ADVANCED_FACE('',(#430,#184),#213,.T.);
#3523=ADVANCED_FACE('',(#431),#101,.T.);
#3524=ADVANCED_FACE('',(#432),#165,.T.);
#3525=ADVANCED_FACE('',(#433,#185),#214,.T.);
#3526=ADVANCED_FACE('',(#434),#102,.T.);
#3527=ADVANCED_FACE('',(#435,#186),#215,.T.);
#3528=ADVANCED_FACE('',(#436),#103,.T.);
#3529=ADVANCED_FACE('',(#437),#166,.T.);
#3530=ADVANCED_FACE('',(#438,#187),#216,.T.);
#3531=ADVANCED_FACE('',(#439),#104,.T.);
#3532=ADVANCED_FACE('',(#440),#105,.T.);
#3533=ADVANCED_FACE('',(#441),#167,.T.);
#3534=ADVANCED_FACE('',(#442),#106,.T.);
#3535=ADVANCED_FACE('',(#443,#188),#217,.T.);
#3536=ADVANCED_FACE('',(#444),#107,.T.);
#3537=ADVANCED_FACE('',(#445),#168,.T.);
#3538=ADVANCED_FACE('',(#446,#189),#218,.T.);
#3539=ADVANCED_FACE('',(#447),#108,.T.);
#3540=ADVANCED_FACE('',(#448,#190),#219,.T.);
#3541=ADVANCED_FACE('',(#449),#109,.T.);
#3542=ADVANCED_FACE('',(#450),#220,.T.);
#3543=ADVANCED_FACE('',(#451),#3420,.T.);
#3544=ADVANCED_FACE('',(#452),#3421,.T.);
#3545=ADVANCED_FACE('',(#453),#3422,.T.);
#3678=CLOSED_SHELL('',(#3496,#3497,#3498,#3499,#3500,#3501,#3502,#3503,
#3504,#3505,#3506,#3507,#3508,#3509,#3510,#3511,#3512,#3513,#3514,#3515,
#3516,#3517,#3518,#3519,#3520,#3521,#3522,#3523,#3524,#3525,#3526,#3527,
#3528,#3529,#3530,#3531,#3532,#3533,#3534,#3535,#3536,#3537,#3538,#3539,
#3540,#3541,#3542,#3543,#3544,#3545));
#3851=AXIS2_PLACEMENT_3D('',#5070,#4235,#4236);
#3852=AXIS2_PLACEMENT_3D('',#5071,#4237,#4238);
#3853=AXIS2_PLACEMENT_3D('',#5233,#4240,#4241);
#3854=AXIS2_PLACEMENT_3D('',#5343,#4242,#4243);
#3855=AXIS2_PLACEMENT_3D('',#5733,#4245,#4246);
#3856=AXIS2_PLACEMENT_3D('',#5859,#4248,#4249);
#3857=AXIS2_PLACEMENT_3D('',#6170,#4251,#4252);
#3858=AXIS2_PLACEMENT_3D('',#6558,#4254,#4255);
#3859=AXIS2_PLACEMENT_3D('',#6957,#4257,#4258);
#3860=AXIS2_PLACEMENT_3D('',#7344,#4260,#4261);
#3861=AXIS2_PLACEMENT_3D('',#7745,#4263,#4264);
#3862=AXIS2_PLACEMENT_3D('',#8140,#4266,#4267);
#3863=AXIS2_PLACEMENT_3D('',#8549,#4269,#4270);
#3864=AXIS2_PLACEMENT_3D('',#8952,#4272,#4273);
#3865=AXIS2_PLACEMENT_3D('',#9334,#4275,#4276);
#3866=AXIS2_PLACEMENT_3D('',#9453,#4278,#4279);
#3867=AXIS2_PLACEMENT_3D('',#9455,#4280,#4281);
#3868=AXIS2_PLACEMENT_3D('',#9458,#4282,#4283);
#3869=AXIS2_PLACEMENT_3D('',#11773,#4284,#4285);
#3870=AXIS2_PLACEMENT_3D('',#14184,#4286,#4287);
#3871=AXIS2_PLACEMENT_3D('',#14284,#4288,#4289);
#3872=AXIS2_PLACEMENT_3D('',#14344,#4290,#4291);
#3873=AXIS2_PLACEMENT_3D('',#14346,#4292,#4293);
#3874=AXIS2_PLACEMENT_3D('',#14348,#4294,#4295);
#3875=AXIS2_PLACEMENT_3D('',#14349,#4296,#4297);
#3876=AXIS2_PLACEMENT_3D('',#14351,#4298,#4299);
#3877=AXIS2_PLACEMENT_3D('',#14353,#4300,#4301);
#3878=AXIS2_PLACEMENT_3D('',#14354,#4302,#4303);
#3879=AXIS2_PLACEMENT_3D('',#14355,#4304,#4305);
#3880=AXIS2_PLACEMENT_3D('',#14358,#4307,#4308);
#3881=AXIS2_PLACEMENT_3D('',#14359,#4309,#4310);
#3882=AXIS2_PLACEMENT_3D('',#14360,#4311,#4312);
#3883=AXIS2_PLACEMENT_3D('',#14361,#4313,#4314);
#3884=AXIS2_PLACEMENT_3D('',#14363,#4315,#4316);
#3885=AXIS2_PLACEMENT_3D('',#14887,#4317,#4318);
#3886=AXIS2_PLACEMENT_3D('',#15420,#4319,#4320);
#3887=AXIS2_PLACEMENT_3D('',#15421,#4321,#4322);
#3888=AXIS2_PLACEMENT_3D('',#15423,#4323,#4324);
#3889=AXIS2_PLACEMENT_3D('',#15425,#4325,#4326);
#3890=AXIS2_PLACEMENT_3D('',#15426,#4327,#4328);
#3891=AXIS2_PLACEMENT_3D('',#15427,#4329,#4330);
#3892=AXIS2_PLACEMENT_3D('',#15430,#4332,#4333);
#3893=AXIS2_PLACEMENT_3D('',#15431,#4334,#4335);
#3894=AXIS2_PLACEMENT_3D('',#15432,#4336,#4337);
#3895=AXIS2_PLACEMENT_3D('',#15434,#4338,#4339);
#3896=AXIS2_PLACEMENT_3D('',#15436,#4340,#4341);
#3897=AXIS2_PLACEMENT_3D('',#15437,#4342,#4343);
#3898=AXIS2_PLACEMENT_3D('',#15438,#4344,#4345);
#3899=AXIS2_PLACEMENT_3D('',#15441,#4347,#4348);
#3900=AXIS2_PLACEMENT_3D('',#15442,#4349,#4350);
#3901=AXIS2_PLACEMENT_3D('',#15443,#4351,#4352);
#3902=AXIS2_PLACEMENT_3D('',#15445,#4353,#4354);
#3903=AXIS2_PLACEMENT_3D('',#15446,#4355,#4356);
#3904=AXIS2_PLACEMENT_3D('',#15447,#4357,#4358);
#3905=AXIS2_PLACEMENT_3D('',#15449,#4359,#4360);
#3906=AXIS2_PLACEMENT_3D('',#15450,#4361,#4362);
#3907=AXIS2_PLACEMENT_3D('',#15452,#4363,#4364);
#3908=AXIS2_PLACEMENT_3D('',#15454,#4365,#4366);
#3909=AXIS2_PLACEMENT_3D('',#15455,#4367,#4368);
#3910=AXIS2_PLACEMENT_3D('',#15456,#4369,#4370);
#3911=AXIS2_PLACEMENT_3D('',#15459,#4372,#4373);
#3912=AXIS2_PLACEMENT_3D('',#15460,#4374,#4375);
#3913=AXIS2_PLACEMENT_3D('',#15462,#4376,#4377);
#3914=AXIS2_PLACEMENT_3D('',#15463,#4378,#4379);
#3915=AXIS2_PLACEMENT_3D('',#15464,#4380,#4381);
#3916=AXIS2_PLACEMENT_3D('',#15465,#4382,#4383);
#3917=AXIS2_PLACEMENT_3D('',#15467,#4384,#4385);
#3918=AXIS2_PLACEMENT_3D('',#15468,#4386,#4387);
#3919=AXIS2_PLACEMENT_3D('',#15469,#4388,#4389);
#3920=AXIS2_PLACEMENT_3D('',#15472,#4391,#4392);
#3921=AXIS2_PLACEMENT_3D('',#15473,#4393,#4394);
#3922=AXIS2_PLACEMENT_3D('',#15475,#4395,#4396);
#3923=AXIS2_PLACEMENT_3D('',#15476,#4397,#4398);
#3924=AXIS2_PLACEMENT_3D('',#15477,#4399,#4400);
#3925=AXIS2_PLACEMENT_3D('',#15479,#4401,#4402);
#3926=AXIS2_PLACEMENT_3D('',#15480,#4403,#4404);
#3927=AXIS2_PLACEMENT_3D('',#15482,#4405,#4406);
#3928=AXIS2_PLACEMENT_3D('',#15484,#4407,#4408);
#3929=AXIS2_PLACEMENT_3D('',#15485,#4409,#4410);
#3930=AXIS2_PLACEMENT_3D('',#15486,#4411,#4412);
#3931=AXIS2_PLACEMENT_3D('',#15489,#4414,#4415);
#3932=AXIS2_PLACEMENT_3D('',#15490,#4416,#4417);
#3933=AXIS2_PLACEMENT_3D('',#15492,#4418,#4419);
#3934=AXIS2_PLACEMENT_3D('',#15493,#4420,#4421);
#3935=AXIS2_PLACEMENT_3D('',#15495,#4422,#4423);
#3936=AXIS2_PLACEMENT_3D('',#15496,#4424,#4425);
#3937=AXIS2_PLACEMENT_3D('',#15497,#4426,#4427);
#3938=AXIS2_PLACEMENT_3D('',#15499,#4428,#4429);
#3939=AXIS2_PLACEMENT_3D('',#15500,#4430,#4431);
#3940=AXIS2_PLACEMENT_3D('',#15502,#4432,#4433);
#3941=AXIS2_PLACEMENT_3D('',#15504,#4434,#4435);
#3942=AXIS2_PLACEMENT_3D('',#15505,#4436,#4437);
#3943=AXIS2_PLACEMENT_3D('',#15506,#4438,#4439);
#3944=AXIS2_PLACEMENT_3D('',#15507,#4440,#4441);
#3945=AXIS2_PLACEMENT_3D('',#15509,#4443,#4444);
#3946=AXIS2_PLACEMENT_3D('',#15511,#4446,#4447);
#4235=DIRECTION('axis',(0.,0.,1.));
#4236=DIRECTION('refdir',(1.,0.,0.));
#4237=DIRECTION('center_axis',(1.,0.,0.));
#4238=DIRECTION('ref_axis',(0.,-0.999641738703431,0.0267655420640338));
#4239=DIRECTION('',(-1.,0.,0.));
#4240=DIRECTION('center_axis',(-1.,0.,0.));
#4241=DIRECTION('ref_axis',(0.,9.28774802075533E-14,-1.));
#4242=DIRECTION('center_axis',(1.,0.,0.));
#4243=DIRECTION('ref_axis',(0.,-0.999641738703431,0.0267655420640338));
#4244=DIRECTION('',(-1.,0.,0.));
#4245=DIRECTION('center_axis',(1.,0.,0.));
#4246=DIRECTION('ref_axis',(0.,-0.999641738703431,0.0267655420640338));
#4247=DIRECTION('',(-1.,0.,0.));
#4248=DIRECTION('center_axis',(1.,0.,0.));
#4249=DIRECTION('ref_axis',(0.,-0.999641738703431,0.0267655420640338));
#4250=DIRECTION('',(-1.,0.,0.));
#4251=DIRECTION('center_axis',(1.,0.,0.));
#4252=DIRECTION('ref_axis',(0.,-0.999641738703431,0.0267655420640338));
#4253=DIRECTION('',(-1.,0.,0.));
#4254=DIRECTION('center_axis',(1.,0.,0.));
#4255=DIRECTION('ref_axis',(0.,-0.999641738703431,0.0267655420640338));
#4256=DIRECTION('',(-1.,0.,0.));
#4257=DIRECTION('center_axis',(1.,0.,0.));
#4258=DIRECTION('ref_axis',(0.,-0.999641738703431,0.0267655420640338));
#4259=DIRECTION('',(-1.,0.,0.));
#4260=DIRECTION('center_axis',(1.,0.,0.));
#4261=DIRECTION('ref_axis',(0.,-0.999641738703431,0.0267655420640338));
#4262=DIRECTION('',(-1.,0.,0.));
#4263=DIRECTION('center_axis',(1.,0.,0.));
#4264=DIRECTION('ref_axis',(0.,-0.999641738703431,0.0267655420640338));
#4265=DIRECTION('',(-1.,0.,0.));
#4266=DIRECTION('center_axis',(1.,0.,0.));
#4267=DIRECTION('ref_axis',(0.,-0.999641738703431,0.0267655420640338));
#4268=DIRECTION('',(-1.,0.,0.));
#4269=DIRECTION('center_axis',(1.,0.,0.));
#4270=DIRECTION('ref_axis',(0.,-0.999641738703431,0.0267655420640338));
#4271=DIRECTION('',(-1.,0.,0.));
#4272=DIRECTION('center_axis',(1.,0.,0.));
#4273=DIRECTION('ref_axis',(0.,-0.999641738703431,0.0267655420640338));
#4274=DIRECTION('',(-1.,0.,0.));
#4275=DIRECTION('center_axis',(1.,0.,0.));
#4276=DIRECTION('ref_axis',(0.,-0.999641738703431,0.0267655420640338));
#4277=DIRECTION('',(-1.,0.,0.));
#4278=DIRECTION('center_axis',(1.,0.,0.));
#4279=DIRECTION('ref_axis',(0.,0.,-1.));
#4280=DIRECTION('center_axis',(-1.,0.,0.));
#4281=DIRECTION('ref_axis',(0.,0.,-1.));
#4282=DIRECTION('center_axis',(-1.,0.,0.));
#4283=DIRECTION('ref_axis',(0.,0.,-1.));
#4284=DIRECTION('center_axis',(-1.,0.,0.));
#4285=DIRECTION('ref_axis',(0.,0.,-1.));
#4286=DIRECTION('center_axis',(1.,0.,0.));
#4287=DIRECTION('ref_axis',(0.,-0.999641738703431,0.0267655420640338));
#4288=DIRECTION('center_axis',(1.,0.,0.));
#4289=DIRECTION('ref_axis',(0.,9.28774802075533E-14,-1.));
#4290=DIRECTION('center_axis',(-1.,0.,0.));
#4291=DIRECTION('ref_axis',(0.,0.,1.));
#4292=DIRECTION('center_axis',(1.,0.,0.));
#4293=DIRECTION('ref_axis',(0.,1.22464679914735E-16,1.));
#4294=DIRECTION('center_axis',(-1.,0.,0.));
#4295=DIRECTION('ref_axis',(0.,1.22464679914735E-16,1.));
#4296=DIRECTION('center_axis',(1.,0.,0.));
#4297=DIRECTION('ref_axis',(0.,0.,-1.));
#4298=DIRECTION('center_axis',(-1.,0.,0.));
#4299=DIRECTION('ref_axis',(0.,0.,-1.));
#4300=DIRECTION('center_axis',(0.,-1.,-1.22464679914735E-16));
#4301=DIRECTION('ref_axis',(0.,-1.22464679914735E-16,1.));
#4302=DIRECTION('center_axis',(1.,0.,0.));
#4303=DIRECTION('ref_axis',(0.,0.,1.));
#4304=DIRECTION('center_axis',(1.,0.,0.));
#4305=DIRECTION('ref_axis',(0.,0.,-1.));
#4306=DIRECTION('',(-0.999999956307574,3.62016965809699E-20,-0.000295609285927787));
#4307=DIRECTION('center_axis',(-1.,0.,0.));
#4308=DIRECTION('ref_axis',(0.,0.,1.));
#4309=DIRECTION('center_axis',(1.,0.,0.));
#4310=DIRECTION('ref_axis',(0.,0.,-1.));
#4311=DIRECTION('center_axis',(0.,-1.,-1.22464679914735E-16));
#4312=DIRECTION('ref_axis',(0.,-1.22464679914735E-16,1.));
#4313=DIRECTION('center_axis',(-1.,0.,0.));
#4314=DIRECTION('ref_axis',(0.,0.,1.));
#4315=DIRECTION('center_axis',(1.,0.,0.));
#4316=DIRECTION('ref_axis',(0.,1.22464679914735E-16,1.));
#4317=DIRECTION('center_axis',(1.,0.,0.));
#4318=DIRECTION('ref_axis',(0.,0.,-1.));
#4319=DIRECTION('center_axis',(1.,0.,0.));
#4320=DIRECTION('ref_axis',(0.,0.,-1.));
#4321=DIRECTION('center_axis',(1.,0.,0.));
#4322=DIRECTION('ref_axis',(0.,0.,-1.));
#4323=DIRECTION('center_axis',(-1.,0.,0.));
#4324=DIRECTION('ref_axis',(0.,1.22464679914735E-16,1.));
#4325=DIRECTION('center_axis',(0.,-1.,-1.22464679914735E-16));
#4326=DIRECTION('ref_axis',(0.,-1.22464679914735E-16,1.));
#4327=DIRECTION('center_axis',(1.,0.,0.));
#4328=DIRECTION('ref_axis',(0.,1.22464679914735E-16,1.));
#4329=DIRECTION('center_axis',(1.,0.,0.));
#4330=DIRECTION('ref_axis',(0.,0.,-1.));
#4331=DIRECTION('',(-1.,0.,0.));
#4332=DIRECTION('center_axis',(1.,0.,0.));
#4333=DIRECTION('ref_axis',(0.,0.,-1.));
#4334=DIRECTION('center_axis',(1.,0.,0.));
#4335=DIRECTION('ref_axis',(0.,0.,-1.));
#4336=DIRECTION('center_axis',(1.,0.,0.));
#4337=DIRECTION('ref_axis',(0.,0.,-1.));
#4338=DIRECTION('center_axis',(-1.,0.,0.));
#4339=DIRECTION('ref_axis',(0.,1.22464679914735E-16,1.));
#4340=DIRECTION('center_axis',(0.,-1.,-1.22464679914735E-16));
#4341=DIRECTION('ref_axis',(0.,-1.22464679914735E-16,1.));
#4342=DIRECTION('center_axis',(1.,0.,0.));
#4343=DIRECTION('ref_axis',(0.,0.,1.));
#4344=DIRECTION('center_axis',(1.,0.,0.));
#4345=DIRECTION('ref_axis',(0.,0.,-1.));
#4346=DIRECTION('',(-0.999999956307574,3.62016965808668E-20,-0.000295609285926945));
#4347=DIRECTION('center_axis',(-1.,0.,0.));
#4348=DIRECTION('ref_axis',(0.,0.,1.));
#4349=DIRECTION('center_axis',(1.,0.,0.));
#4350=DIRECTION('ref_axis',(0.,0.,-1.));
#4351=DIRECTION('center_axis',(1.,0.,0.));
#4352=DIRECTION('ref_axis',(0.,0.,-1.));
#4353=DIRECTION('center_axis',(0.,-1.,-1.22464679914735E-16));
#4354=DIRECTION('ref_axis',(0.,-1.22464679914735E-16,1.));
#4355=DIRECTION('center_axis',(1.,0.,0.));
#4356=DIRECTION('ref_axis',(0.,1.22464679914735E-16,1.));
#4357=DIRECTION('center_axis',(-1.,0.,0.));
#4358=DIRECTION('ref_axis',(0.,0.,1.));
#4359=DIRECTION('center_axis',(1.,0.,0.));
#4360=DIRECTION('ref_axis',(0.,0.,-1.));
#4361=DIRECTION('center_axis',(1.,0.,0.));
#4362=DIRECTION('ref_axis',(0.,0.,-1.));
#4363=DIRECTION('center_axis',(-1.,0.,0.));
#4364=DIRECTION('ref_axis',(0.,1.22464679914735E-16,1.));
#4365=DIRECTION('center_axis',(0.,-1.,-1.22464679914735E-16));
#4366=DIRECTION('ref_axis',(0.,-1.22464679914735E-16,1.));
#4367=DIRECTION('center_axis',(1.,0.,0.));
#4368=DIRECTION('ref_axis',(0.,0.,1.));
#4369=DIRECTION('center_axis',(1.,0.,0.));
#4370=DIRECTION('ref_axis',(0.,0.,-1.));
#4371=DIRECTION('',(-0.999999956307574,3.62016965808707E-20,-0.000295609285926977));
#4372=DIRECTION('center_axis',(-1.,0.,0.));
#4373=DIRECTION('ref_axis',(0.,0.,1.));
#4374=DIRECTION('center_axis',(1.,0.,0.));
#4375=DIRECTION('ref_axis',(0.,0.,-1.));
#4376=DIRECTION('center_axis',(1.,0.,0.));
#4377=DIRECTION('ref_axis',(0.,0.,-1.));
#4378=DIRECTION('center_axis',(1.,0.,0.));
#4379=DIRECTION('ref_axis',(0.,0.,-1.));
#4380=DIRECTION('center_axis',(0.,-1.,-1.22464679914735E-16));
#4381=DIRECTION('ref_axis',(0.,-1.22464679914735E-16,1.));
#4382=DIRECTION('center_axis',(1.,0.,0.));
#4383=DIRECTION('ref_axis',(0.,0.,-1.));
#4384=DIRECTION('center_axis',(0.,-1.,-1.22464679914735E-16));
#4385=DIRECTION('ref_axis',(0.,-1.22464679914735E-16,1.));
#4386=DIRECTION('center_axis',(1.,0.,0.));
#4387=DIRECTION('ref_axis',(0.,0.,1.));
#4388=DIRECTION('center_axis',(1.,0.,0.));
#4389=DIRECTION('ref_axis',(0.,0.,-1.));
#4390=DIRECTION('',(-0.999999956307574,3.62016965808673E-20,-0.000295609285926949));
#4391=DIRECTION('center_axis',(-1.,0.,0.));
#4392=DIRECTION('ref_axis',(0.,0.,1.));
#4393=DIRECTION('center_axis',(1.,0.,0.));
#4394=DIRECTION('ref_axis',(0.,0.,-1.));
#4395=DIRECTION('center_axis',(0.,-1.,-1.22464679914735E-16));
#4396=DIRECTION('ref_axis',(0.,-1.22464679914735E-16,1.));
#4397=DIRECTION('center_axis',(1.,0.,0.));
#4398=DIRECTION('ref_axis',(0.,1.22464679914735E-16,1.));
#4399=DIRECTION('center_axis',(-1.,0.,0.));
#4400=DIRECTION('ref_axis',(0.,0.,1.));
#4401=DIRECTION('center_axis',(1.,0.,0.));
#4402=DIRECTION('ref_axis',(0.,0.,-1.));
#4403=DIRECTION('center_axis',(1.,0.,0.));
#4404=DIRECTION('ref_axis',(0.,0.,-1.));
#4405=DIRECTION('center_axis',(-1.,0.,0.));
#4406=DIRECTION('ref_axis',(0.,1.22464679914735E-16,1.));
#4407=DIRECTION('center_axis',(0.,-1.,-1.22464679914735E-16));
#4408=DIRECTION('ref_axis',(0.,-1.22464679914735E-16,1.));
#4409=DIRECTION('center_axis',(1.,0.,0.));
#4410=DIRECTION('ref_axis',(0.,0.,1.));
#4411=DIRECTION('center_axis',(1.,0.,0.));
#4412=DIRECTION('ref_axis',(0.,0.,-1.));
#4413=DIRECTION('',(-0.999999956307574,3.62016965810123E-20,-0.000295609285928133));
#4414=DIRECTION('center_axis',(-1.,0.,0.));
#4415=DIRECTION('ref_axis',(0.,0.,1.));
#4416=DIRECTION('center_axis',(1.,0.,0.));
#4417=DIRECTION('ref_axis',(0.,0.,-1.));
#4418=DIRECTION('center_axis',(1.,0.,0.));
#4419=DIRECTION('ref_axis',(0.,0.,-1.));
#4420=DIRECTION('center_axis',(1.,0.,0.));
#4421=DIRECTION('ref_axis',(0.,0.,-1.));
#4422=DIRECTION('center_axis',(0.,-1.,-1.22464679914735E-16));
#4423=DIRECTION('ref_axis',(0.,-1.22464679914735E-16,1.));
#4424=DIRECTION('center_axis',(1.,0.,0.));
#4425=DIRECTION('ref_axis',(0.,1.22464679914735E-16,1.));
#4426=DIRECTION('center_axis',(-1.,0.,0.));
#4427=DIRECTION('ref_axis',(0.,0.,1.));
#4428=DIRECTION('center_axis',(1.,0.,0.));
#4429=DIRECTION('ref_axis',(0.,0.,-1.));
#4430=DIRECTION('center_axis',(1.,0.,0.));
#4431=DIRECTION('ref_axis',(0.,0.,-1.));
#4432=DIRECTION('center_axis',(-1.,0.,0.));
#4433=DIRECTION('ref_axis',(0.,1.22464679914735E-16,1.));
#4434=DIRECTION('center_axis',(0.,-1.,-1.22464679914735E-16));
#4435=DIRECTION('ref_axis',(0.,-1.22464679914735E-16,1.));
#4436=DIRECTION('center_axis',(1.,0.,0.));
#4437=DIRECTION('ref_axis',(0.,1.22464679914735E-16,1.));
#4438=DIRECTION('center_axis',(-1.,0.,0.));
#4439=DIRECTION('ref_axis',(0.,0.,1.));
#4440=DIRECTION('center_axis',(1.,0.,0.));
#4441=DIRECTION('ref_axis',(0.,0.,-1.));
#4442=DIRECTION('',(-1.,0.,0.));
#4443=DIRECTION('center_axis',(1.,0.,0.));
#4444=DIRECTION('ref_axis',(0.,0.,-1.));
#4445=DIRECTION('',(-1.,0.,0.));
#4446=DIRECTION('center_axis',(1.,0.,0.));
#4447=DIRECTION('ref_axis',(0.,0.,-1.));
#4448=DIRECTION('',(-1.,0.,0.));
#5070=CARTESIAN_POINT('',(0.,0.,0.));
#5071=CARTESIAN_POINT('Origin',(88.3562164250559,0.,0.));
#5072=CARTESIAN_POINT('',(90.9367078804579,1.77561363837187,-0.0475422940951198));
#5073=CARTESIAN_POINT('',(90.790457845232,1.77561363837197,-0.0475422940912425));
#5074=CARTESIAN_POINT('',(88.3562164250559,1.77561363837197,-0.0475422940912398));
#5075=CARTESIAN_POINT('',(90.3790868290973,0.00149166109910448,1.77624937366552));
#5076=CARTESIAN_POINT('Ctrl Pts',(90.9367078804579,1.77561363837187,-0.0475422940950947));
#5077=CARTESIAN_POINT('Ctrl Pts',(90.9364406478333,1.7755088947135,-0.05145426914555));
#5078=CARTESIAN_POINT('Ctrl Pts',(90.9361741013816,1.77539122163591,-0.0553659470277124));
#5079=CARTESIAN_POINT('Ctrl Pts',(90.9354289302851,1.77502512697568,-0.0663299051595725));
#5080=CARTESIAN_POINT('Ctrl Pts',(90.9349519773079,1.77474761564714,-0.0733809392859071));
#5081=CARTESIAN_POINT('Ctrl Pts',(90.9338700479988,1.77401920580607,-0.0894508407210216));
#5082=CARTESIAN_POINT('Ctrl Pts',(90.9332665466041,1.7735415502998,-0.0984681352261746));
#5083=CARTESIAN_POINT('Ctrl Pts',(90.9313857021166,1.77182868231983,-0.126723255478906));
#5084=CARTESIAN_POINT('Ctrl Pts',(90.9301209560697,1.77034901257526,-0.145945574748464));
#5085=CARTESIAN_POINT('Ctrl Pts',(90.9271215763623,1.7660535158258,-0.191947670512226));
#5086=CARTESIAN_POINT('Ctrl Pts',(90.9253998762074,1.7629411144518,-0.218695472152004));
#5087=CARTESIAN_POINT('Ctrl Pts',(90.9185480272457,1.74797956202784,-0.325967674584511));
#5088=CARTESIAN_POINT('Ctrl Pts',(90.9135720397987,1.73121033391175,-0.405709252183148));
#5089=CARTESIAN_POINT('Ctrl Pts',(90.9019699944758,1.67970739744729,-0.587559898655641));
#5090=CARTESIAN_POINT('Ctrl Pts',(90.8953431282698,1.64104035264349,-0.688205369161317));
#5091=CARTESIAN_POINT('Ctrl Pts',(90.8868307636316,1.58265962080283,-0.806756158773526));
#5092=CARTESIAN_POINT('Ctrl Pts',(90.8852351222549,1.57135666021832,-0.828556049690737));
#5093=CARTESIAN_POINT('Ctrl Pts',(90.8826014014651,1.55214864891183,-0.863794774706981));
#5094=CARTESIAN_POINT('Ctrl Pts',(90.8815727556905,1.5445119213898,-0.877376623809287));
#5095=CARTESIAN_POINT('Ctrl Pts',(90.8797055013338,1.53041499760629,-0.901693362873107));
#5096=CARTESIAN_POINT('Ctrl Pts',(90.8788692159976,1.52401796437476,-0.912463816263084));
#5097=CARTESIAN_POINT('Ctrl Pts',(90.8770608598892,1.51001030365971,-0.935489734553268));
#5098=CARTESIAN_POINT('Ctrl Pts',(90.8760874939559,1.50236326652315,-0.947721876188245));
#5099=CARTESIAN_POINT('Ctrl Pts',(90.8733649913025,1.48068380974828,-0.981478314697449));
#5100=CARTESIAN_POINT('Ctrl Pts',(90.8716041266841,1.46633256015355,-1.0027925654589));
#5101=CARTESIAN_POINT('Ctrl Pts',(90.8640001035302,1.40299491096074,-1.09259264298843));
#5102=CARTESIAN_POINT('Ctrl Pts',(90.8579947681781,1.34964111770653,-1.15785089795823));
#5103=CARTESIAN_POINT('Ctrl Pts',(90.8426298158545,1.20429945138372,-1.31187150595062));
#5104=CARTESIAN_POINT('Ctrl Pts',(90.8331636770439,1.10698655422456,-1.39496453935183));
#5105=CARTESIAN_POINT('Ctrl Pts',(90.8225011795454,0.982406882686855,-1.48002751671084));
#5106=CARTESIAN_POINT('Ctrl Pts',(90.8208744920965,0.962947193885271,-1.49276172278426));
#5107=CARTESIAN_POINT('Ctrl Pts',(90.8186447573278,0.935566062419342,-1.50992127779915));
#5108=CARTESIAN_POINT('Ctrl Pts',(90.8180230580811,0.927853263265728,-1.51467305149509));
#5109=CARTESIAN_POINT('Ctrl Pts',(90.8169117880306,0.913919415775024,-1.52311117268993));
#5110=CARTESIAN_POINT('Ctrl Pts',(90.8164208879198,0.907711579817898,-1.52681892776984));
#5111=CARTESIAN_POINT('Ctrl Pts',(90.8154093083889,0.894806694745356,-1.53442009999958));
#5112=CARTESIAN_POINT('Ctrl Pts',(90.8148889836212,0.888106555159891,-1.53830777696759));
#5113=CARTESIAN_POINT('Ctrl Pts',(90.8135111430629,0.870205266059774,-1.54853884429454));
#5114=CARTESIAN_POINT('Ctrl Pts',(90.8126583732215,0.858959991189343,-1.5548046548435));
#5115=CARTESIAN_POINT('Ctrl Pts',(90.8082958618394,0.800639346221723,-1.58647472625119));
#5116=CARTESIAN_POINT('Ctrl Pts',(90.8048946921989,0.752497407587655,-1.60986777132373));
#5117=CARTESIAN_POINT('Ctrl Pts',(90.7907852954617,0.545390013993606,-1.69917981864387));
#5118=CARTESIAN_POINT('Ctrl Pts',(90.7805650191555,0.378360401570082,-1.74399212453831));
#5119=CARTESIAN_POINT('Ctrl Pts',(90.7678905896674,0.18291815532491,-1.76697964699746));
#5120=CARTESIAN_POINT('Ctrl Pts',(90.766283107693,0.158290967091757,-1.7693558145486));
#5121=CARTESIAN_POINT('Ctrl Pts',(90.7636332423648,0.118022107291155,-1.77239375459435));
#5122=CARTESIAN_POINT('Ctrl Pts',(90.7626004549225,0.102406663617898,-1.77336451084305));
#5123=CARTESIAN_POINT('Ctrl Pts',(90.7607277113767,0.0742484381325717,-1.77474185976951));
#5124=CARTESIAN_POINT('Ctrl Pts',(90.7598901137838,0.0617101773089686,-1.77522205358507));
#5125=CARTESIAN_POINT('Ctrl Pts',(90.7580811230724,0.0347573469733052,-1.77596841747888));
#5126=CARTESIAN_POINT('Ctrl Pts',(90.7571084574451,0.0203426008238719,-1.77619200828667));
#5127=CARTESIAN_POINT('Ctrl Pts',(90.7543939580964,-0.0196611554975341,
-1.77632549583768));
#5128=CARTESIAN_POINT('Ctrl Pts',(90.7526405406671,-0.0452470277500012,
-1.77585793796779));
#5129=CARTESIAN_POINT('Ctrl Pts',(90.7451082126153,-0.154032241144647,-1.77151760885236));
#5130=CARTESIAN_POINT('Ctrl Pts',(90.739170874313,-0.236903575661729,-1.76234894663126));
#5131=CARTESIAN_POINT('Ctrl Pts',(90.7242598777567,-0.439148955545672,-1.72544899074502));
#5132=CARTESIAN_POINT('Ctrl Pts',(90.7151928678592,-0.556890668247468,-1.69112371261827));
#5133=CARTESIAN_POINT('Ctrl Pts',(90.7044862299971,-0.696376849201785,-1.63429618824903));
#5134=CARTESIAN_POINT('Ctrl Pts',(90.7024975405662,-0.722324877688078,-1.62299468088015));
#5135=CARTESIAN_POINT('Ctrl Pts',(90.6997969830317,-0.757751871638434,-1.60654658113198));
#5136=CARTESIAN_POINT('Ctrl Pts',(90.6990577921756,-0.767469246832142,-1.6019272099874));
#5137=CARTESIAN_POINT('Ctrl Pts',(90.6978320942622,-0.783626006802249,-1.59406596531438));
#5138=CARTESIAN_POINT('Ctrl Pts',(90.6973427239503,-0.790088596149161,-1.5908727280353));
#5139=CARTESIAN_POINT('Ctrl Pts',(90.6963377104244,-0.803388887721289,-1.5841998652902));
#5140=CARTESIAN_POINT('Ctrl Pts',(90.6958223965398,-0.810223814011509,-1.58071512137936));
#5141=CARTESIAN_POINT('Ctrl Pts',(90.6944569908053,-0.828367329306277,-1.57131616269045));
#5142=CARTESIAN_POINT('Ctrl Pts',(90.6936116210907,-0.839635369012165,-1.56532405143173));
#5143=CARTESIAN_POINT('Ctrl Pts',(90.6892939826121,-0.897297787560878,-1.53385852329897));
#5144=CARTESIAN_POINT('Ctrl Pts',(90.6859293689884,-0.942605925081128,-1.50643968126981));
#5145=CARTESIAN_POINT('Ctrl Pts',(90.6723962832535,-1.12259627611808,-1.38621022416122));
#5146=CARTESIAN_POINT('Ctrl Pts',(90.6626870602337,-1.24537114954097,-1.27704934107327));
#5147=CARTESIAN_POINT('Ctrl Pts',(90.6500456738212,-1.37380638022623,-1.12645613364311));
#5148=CARTESIAN_POINT('Ctrl Pts',(90.6478226219318,-1.39536232499479,-1.09964136062491));
#5149=CARTESIAN_POINT('Ctrl Pts',(90.6445181375125,-1.42580205583846,-1.05943831812827));
#5150=CARTESIAN_POINT('Ctrl Pts',(90.6434611041254,-1.43530524041664,-1.04652753952237));
#5151=CARTESIAN_POINT('Ctrl Pts',(90.6415680174533,-1.45190194345323,-1.02332835565672));
#5152=CARTESIAN_POINT('Ctrl Pts',(90.6407347009393,-1.45906417564596,-1.01309026964812));
#5153=CARTESIAN_POINT('Ctrl Pts',(90.6389606136308,-1.47400566378672,-0.991244969840101));
#5154=CARTESIAN_POINT('Ctrl Pts',(90.6380188571002,-1.48175712458954,-0.979619870800271));
#5155=CARTESIAN_POINT('Ctrl Pts',(90.6354594795324,-1.50233343771649,-0.947957922257173));
#5156=CARTESIAN_POINT('Ctrl Pts',(90.6338321691614,-1.51489382192812,-0.927753519175028));
#5157=CARTESIAN_POINT('Ctrl Pts',(90.6301785787599,-1.54192939241401,-0.882251108812333));
#5158=CARTESIAN_POINT('Ctrl Pts',(90.6281454644399,-1.55619506279705,-0.856837223838339));
#5159=CARTESIAN_POINT('Ctrl Pts',(90.6214982588089,-1.60033899086924,-0.773454197305031));
#5160=CARTESIAN_POINT('Ctrl Pts',(90.6168074786084,-1.62764994047824,-0.714192200532683));
#5161=CARTESIAN_POINT('Ctrl Pts',(90.6050019226972,-1.68736670940282,-0.563281292074101));
#5162=CARTESIAN_POINT('Ctrl Pts',(90.5978372502738,-1.715630527162,-0.470217389575858));
#5163=CARTESIAN_POINT('Ctrl Pts',(90.5878271468518,-1.74502631577079,-0.334235186265452));
#5164=CARTESIAN_POINT('Ctrl Pts',(90.5848416840981,-1.7524458926945,-0.292854939791319));
#5165=CARTESIAN_POINT('Ctrl Pts',(90.5810695502963,-1.76013237667591,-0.239059905010199));
#5166=CARTESIAN_POINT('Ctrl Pts',(90.5802209201071,-1.76174704817757,-0.22685453779923));
#5167=CARTESIAN_POINT('Ctrl Pts',(90.578860302099,-1.76415135535286,-0.207102873126839));
#5168=CARTESIAN_POINT('Ctrl Pts',(90.5783441518275,-1.76501974263209,-0.199566826560699));
#5169=CARTESIAN_POINT('Ctrl Pts',(90.5773306912117,-1.76663865644254,-0.184679502025739));
#5170=CARTESIAN_POINT('Ctrl Pts',(90.5768332525516,-1.76739164093947,-0.177328658917269));
#5171=CARTESIAN_POINT('Ctrl Pts',(90.5755863520991,-1.769172932245,-0.158799270129472));
#5172=CARTESIAN_POINT('Ctrl Pts',(90.5748401425478,-1.77014120249121,-0.147615079978273));
#5173=CARTESIAN_POINT('Ctrl Pts',(90.5718371743613,-1.77363506255843,-0.102258514779939));
#5174=CARTESIAN_POINT('Ctrl Pts',(90.5696238404745,-1.77527781888608,-0.068023265765211));
#5175=CARTESIAN_POINT('Ctrl Pts',(90.5634622930758,-1.77711798315338,0.0287794297197061));
#5176=CARTESIAN_POINT('Ctrl Pts',(90.559593290057,-1.77500262495174,0.0913418981976327));
#5177=CARTESIAN_POINT('Ctrl Pts',(90.5473512532474,-1.75778691318612,0.289594850817781));
#5178=CARTESIAN_POINT('Ctrl Pts',(90.5390599267307,-1.73036340619092,0.42369608380026));
#5179=CARTESIAN_POINT('Ctrl Pts',(90.5286058814987,-1.67991461230748,0.577583099874535));
#5180=CARTESIAN_POINT('Ctrl Pts',(90.5269432945398,-1.67144328199262,0.601658200806042));
#5181=CARTESIAN_POINT('Ctrl Pts',(90.5243040799533,-1.65732118387112,0.639189483336105));
#5182=CARTESIAN_POINT('Ctrl Pts',(90.5233389493616,-1.6520180482435,0.652773352068889));
#5183=CARTESIAN_POINT('Ctrl Pts',(90.5216142649825,-1.64230019469282,0.676788292740844));
#5184=CARTESIAN_POINT('Ctrl Pts',(90.5208569756628,-1.63795177301964,0.687245445055579));
#5185=CARTESIAN_POINT('Ctrl Pts',(90.5190901271027,-1.62762026003468,0.711435684910198));
#5186=CARTESIAN_POINT('Ctrl Pts',(90.518078093155,-1.62156292498031,0.725135919063111));
#5187=CARTESIAN_POINT('Ctrl Pts',(90.5151428916477,-1.60359987427085,0.764413097628829));
#5188=CARTESIAN_POINT('Ctrl Pts',(90.5132050052202,-1.59125762523076,0.789784117986039));
#5189=CARTESIAN_POINT('Ctrl Pts',(90.5087230536394,-1.56163446014763,0.847162516906397));
#5190=CARTESIAN_POINT('Ctrl Pts',(90.5061666998465,-1.54396452489455,0.878953783391171));
#5191=CARTESIAN_POINT('Ctrl Pts',(90.4967276419374,-1.47591040084928,0.993003005017456));
#5192=CARTESIAN_POINT('Ctrl Pts',(90.4896806575694,-1.41982860034292,1.0716575807583));
#5193=CARTESIAN_POINT('Ctrl Pts',(90.4766256718245,-1.30459225405994,1.20825197639796));
#5194=CARTESIAN_POINT('Ctrl Pts',(90.4706357231352,-1.24722682831556,1.26738373712288));
#5195=CARTESIAN_POINT('Ctrl Pts',(90.4635911250846,-1.17242148549561,1.33447473370843));
#5196=CARTESIAN_POINT('Ctrl Pts',(90.4623272400515,-1.15869317950186,1.34641194810373));
#5197=CARTESIAN_POINT('Ctrl Pts',(90.4604673720094,-1.13799693689821,1.36385696084663));
#5198=CARTESIAN_POINT('Ctrl Pts',(90.4598608449729,-1.13116764329429,1.36952641786419));
#5199=CARTESIAN_POINT('Ctrl Pts',(90.4587698246762,-1.11873261545039,1.37969309531884));
#5200=CARTESIAN_POINT('Ctrl Pts',(90.4582841636812,-1.11314188310701,1.38420766252412));
#5201=CARTESIAN_POINT('Ctrl Pts',(90.4571831855773,-1.10034333783009,1.39441491318847));
#5202=CARTESIAN_POINT('Ctrl Pts',(90.456569361653,-1.09311858222134,1.4000857779059));
#5203=CARTESIAN_POINT('Ctrl Pts',(90.4546657645702,-1.0704465932619,1.41759902385506));
#5204=CARTESIAN_POINT('Ctrl Pts',(90.4533884615712,-1.05484792220282,1.42924414872662));
#5205=CARTESIAN_POINT('Ctrl Pts',(90.4465481035699,-0.969429811660141,1.49085226171763));
#5206=CARTESIAN_POINT('Ctrl Pts',(90.4412311971354,-0.896241933193827,1.53596492986674));
#5207=CARTESIAN_POINT('Ctrl Pts',(90.4291874646331,-0.723032100909454,1.62611686355231));
#5208=CARTESIAN_POINT('Ctrl Pts',(90.4224892885638,-0.62154285176125,1.66754722517513));
#5209=CARTESIAN_POINT('Ctrl Pts',(90.4131880519771,-0.482157299403821,1.70994340869914));
#5210=CARTESIAN_POINT('Ctrl Pts',(90.4108429667422,-0.447109704668306,1.71944024357985));
#5211=CARTESIAN_POINT('Ctrl Pts',(90.4073928178437,-0.395889829676749,1.73164740463657));
#5212=CARTESIAN_POINT('Ctrl Pts',(90.4063146914316,-0.379930978291518,1.7352186933647));
#5213=CARTESIAN_POINT('Ctrl Pts',(90.404382367012,-0.351427985210454,1.74118507508166));
#5214=CARTESIAN_POINT('Ctrl Pts',(90.4035309399273,-0.338902893809712,1.74366622627442));
#5215=CARTESIAN_POINT('Ctrl Pts',(90.401879394256,-0.314680080017998,1.74819378586932));
#5216=CARTESIAN_POINT('Ctrl Pts',(90.4010798972719,-0.302986414349454,1.75025834854431));
#5217=CARTESIAN_POINT('Ctrl Pts',(90.3993386860087,-0.277594124432116,1.75447936762318));
#5218=CARTESIAN_POINT('Ctrl Pts',(90.3983956820409,-0.263889269859646,1.7565929476446));
#5219=CARTESIAN_POINT('Ctrl Pts',(90.3953272929415,-0.219456873991419,1.76291366473226));
#5220=CARTESIAN_POINT('Ctrl Pts',(90.3931822805761,-0.188644984952052,1.76647637174408));
#5221=CARTESIAN_POINT('Ctrl Pts',(90.3872951384509,-0.10478676224065,1.77395376904623));
#5222=CARTESIAN_POINT('Ctrl Pts',(90.3835097511813,-0.0516363347368595,
1.77629526122296));
#5223=CARTESIAN_POINT('Ctrl Pts',(90.3796762924913,0.00153415989328701,
1.77624933746741));
#5224=CARTESIAN_POINT('',(90.3499141080351,0.430772083774147,1.72400118248596));
#5225=CARTESIAN_POINT('Ctrl Pts',(90.3499212718705,0.430397524873051,1.72331715974836));
#5226=CARTESIAN_POINT('Ctrl Pts',(90.354782198075,0.360606047738533,1.74074754326541));
#5227=CARTESIAN_POINT('Ctrl Pts',(90.3596431242794,0.289637073919477,1.75396322484711));
#5228=CARTESIAN_POINT('Ctrl Pts',(90.3645040504839,0.217984708007283,1.76282351061443));
#5229=CARTESIAN_POINT('Ctrl Pts',(90.3693649766884,0.146332342095089,1.77168379638175));
#5230=CARTESIAN_POINT('Ctrl Pts',(90.3742259028928,0.0739968663745415,1.77618848514627));
#5231=CARTESIAN_POINT('Ctrl Pts',(90.3790868290973,0.00149166109910448,
1.77624937366552));
#5232=CARTESIAN_POINT('',(90.3498698986825,-1.48890580190326,0.968619417293912));
#5233=CARTESIAN_POINT('Origin',(90.3498698986825,0.,0.));
#5234=CARTESIAN_POINT('Ctrl Pts',(90.3498698986825,-1.48890580190326,0.968619417293917));
#5235=CARTESIAN_POINT('Ctrl Pts',(90.3542650496983,-1.52457107695468,0.913796817207203));
#5236=CARTESIAN_POINT('Ctrl Pts',(90.3586602007142,-1.55723341380908,0.856958034254269));
#5237=CARTESIAN_POINT('Ctrl Pts',(90.36305535173,-1.58667231885172,0.798457898132208));
#5238=CARTESIAN_POINT('Ctrl Pts',(90.3674705710205,-1.61624564203603,0.739690650187431));
#5239=CARTESIAN_POINT('Ctrl Pts',(90.371885790311,-1.64256575033591,0.679247235760215));
#5240=CARTESIAN_POINT('Ctrl Pts',(90.3763010096014,-1.66545525170715,0.617513454963586));
#5241=CARTESIAN_POINT('Ctrl Pts',(90.3806927242746,-1.68822289979423,0.556108316709745));
#5242=CARTESIAN_POINT('Ctrl Pts',(90.3850844389477,-1.70759623302425,0.493426970910843));
#5243=CARTESIAN_POINT('Ctrl Pts',(90.3894761536209,-1.72344922018923,0.429868407689064));
#5244=CARTESIAN_POINT('Ctrl Pts',(90.3938679372515,-1.73930245627353,0.366308846487906));
#5245=CARTESIAN_POINT('Ctrl Pts',(90.3982597208822,-1.75163512245982,0.301872497983461));
#5246=CARTESIAN_POINT('Ctrl Pts',(90.4026515045129,-1.76037179242643,0.236970915787881));
#5247=CARTESIAN_POINT('Ctrl Pts',(90.4070446198946,-1.76911111167417,0.172049653034722));
#5248=CARTESIAN_POINT('Ctrl Pts',(90.4114377352763,-1.77425220553906,0.106663343536512));
#5249=CARTESIAN_POINT('Ctrl Pts',(90.415830850658,-1.77577143528477,0.0412295055351104));
#5250=CARTESIAN_POINT('Ctrl Pts',(90.420263330995,-1.77730427824246,-0.0247906589979149));
#5251=CARTESIAN_POINT('Ctrl Pts',(90.4246958113319,-1.7751500030428,-0.0908587202707488));
#5252=CARTESIAN_POINT('Ctrl Pts',(90.4291282916689,-1.76933800722062,-0.156547368884247));
#5253=CARTESIAN_POINT('Ctrl Pts',(90.4335309847615,-1.7635650692908,-0.221794575307162));
#5254=CARTESIAN_POINT('Ctrl Pts',(90.4379336778541,-1.754183558958,-0.286666991404655));
#5255=CARTESIAN_POINT('Ctrl Pts',(90.4423363709467,-1.74127406352506,-0.350754469957176));
#5256=CARTESIAN_POINT('Ctrl Pts',(90.4467837449058,-1.72823355567973,-0.415492342261526));
#5257=CARTESIAN_POINT('Ctrl Pts',(90.451231118865,-1.71159317016332,-0.479428777441116));
#5258=CARTESIAN_POINT('Ctrl Pts',(90.4556784928241,-1.69148746417727,-0.542157007730383));
#5259=CARTESIAN_POINT('Ctrl Pts',(90.4601258667833,-1.67138175819121,-0.604885238019651));
#5260=CARTESIAN_POINT('Ctrl Pts',(90.4645732407425,-1.64781096407574,-0.666404828878841));
#5261=CARTESIAN_POINT('Ctrl Pts',(90.4690206147016,-1.62095839669095,-0.726331837865526));
#5262=CARTESIAN_POINT('Ctrl Pts',(90.4732817188201,-1.59523049826715,-0.783748917504813));
#5263=CARTESIAN_POINT('Ctrl Pts',(90.4775428229385,-1.56638569702523,-0.839936213934016));
#5264=CARTESIAN_POINT('Ctrl Pts',(90.4818039270569,-1.53456308597654,-0.894527918881331));
#5265=CARTESIAN_POINT('Ctrl Pts',(90.4862359022096,-1.50146438255593,-0.951308760921983));
#5266=CARTESIAN_POINT('Ctrl Pts',(90.4906678773623,-1.46514408957627,-1.00636277571506));
#5267=CARTESIAN_POINT('Ctrl Pts',(90.4950998525149,-1.42581458344523,-1.05930016337906));
#5268=CARTESIAN_POINT('Ctrl Pts',(90.4993477343201,-1.38811872826863,-1.11003866215809));
#5269=CARTESIAN_POINT('Ctrl Pts',(90.5035956161253,-1.34765904649706,-1.15883242890056));
#5270=CARTESIAN_POINT('Ctrl Pts',(90.5078434979305,-1.3046685113476,-1.20536473235201));
#5271=CARTESIAN_POINT('Ctrl Pts',(90.5120883386773,-1.26170875312058,-1.25186372332924));
#5272=CARTESIAN_POINT('Ctrl Pts',(90.516333179424,-1.21622207966895,-1.29610408253071));
#5273=CARTESIAN_POINT('Ctrl Pts',(90.5205780201708,-1.16848166994252,-1.33780217129004));
#5274=CARTESIAN_POINT('Ctrl Pts',(90.5248214199474,-1.12075746636133,-1.37948610505391));
#5275=CARTESIAN_POINT('Ctrl Pts',(90.529064819724,-1.07078143086178,-1.4186291419559));
#5276=CARTESIAN_POINT('Ctrl Pts',(90.5333082195006,-1.01886197753949,-1.45498602509588));
#5277=CARTESIAN_POINT('Ctrl Pts',(90.5375517761135,-0.966940605271517,-1.49134425198815));
#5278=CARTESIAN_POINT('Ctrl Pts',(90.5417953327264,-0.913076095775772,-1.52491582865905));
#5279=CARTESIAN_POINT('Ctrl Pts',(90.5460388893393,-0.857606422015877,-1.55549840482629));
#5280=CARTESIAN_POINT('Ctrl Pts',(90.5502869934474,-0.802077305646338,-1.58611375400288));
#5281=CARTESIAN_POINT('Ctrl Pts',(90.5545350975556,-0.744940045311707,-1.61373346556902));
#5282=CARTESIAN_POINT('Ctrl Pts',(90.5587832016638,-0.686556629401138,-1.63820147024881));
#5283=CARTESIAN_POINT('Ctrl Pts',(90.5630340088166,-0.628136064453105,-1.66268504378164));
#5284=CARTESIAN_POINT('Ctrl Pts',(90.5672848159693,-0.56846825163121,-1.68401275130926));
#5285=CARTESIAN_POINT('Ctrl Pts',(90.5715356231221,-0.50793161955539,-1.70207800419248));
#5286=CARTESIAN_POINT('Ctrl Pts',(90.5757937716034,-0.44729043808791,-1.72017445655169));
#5287=CARTESIAN_POINT('Ctrl Pts',(90.5800519200847,-0.385777944191992,-1.73499710021916));
#5288=CARTESIAN_POINT('Ctrl Pts',(90.584310068566,-0.32378277377414,-1.74649041735336));
#5289=CARTESIAN_POINT('Ctrl Pts',(90.5855971559509,-0.305043830751616,-1.74996443982102));
#5290=CARTESIAN_POINT('Ctrl Pts',(90.5868842433359,-0.286260816369676,-1.75313464227076));
#5291=CARTESIAN_POINT('Ctrl Pts',(90.5881713307208,-0.267444501795399,-1.75600042738019));
#5292=CARTESIAN_POINT('Ctrl Pts',(90.5924735824778,-0.204548599478252,-1.76557967519693));
#5293=CARTESIAN_POINT('Ctrl Pts',(90.5967758342347,-0.141009940094459,-1.77179489134502));
#5294=CARTESIAN_POINT('Ctrl Pts',(90.6010780859917,-0.0772198733713044,
-1.77457069559275));
#5295=CARTESIAN_POINT('Ctrl Pts',(90.6055049176896,-0.0115826430720942,
-1.7774268785697));
#5296=CARTESIAN_POINT('Ctrl Pts',(90.6099317493874,0.0543202676253199,-1.77664118668768));
#5297=CARTESIAN_POINT('Ctrl Pts',(90.6143585810852,0.12005235508134,-1.77218833495185));
#5298=CARTESIAN_POINT('Ctrl Pts',(90.6186489176737,0.183757686365544,-1.76787278061653));
#5299=CARTESIAN_POINT('Ctrl Pts',(90.6229392542622,0.247302032647212,-1.76011297008372));
#5300=CARTESIAN_POINT('Ctrl Pts',(90.6272295908507,0.310286434006175,-1.7489386471148));
#5301=CARTESIAN_POINT('Ctrl Pts',(90.6315172607396,0.37323168681021,-1.73777126965281));
#5302=CARTESIAN_POINT('Ctrl Pts',(90.6358049306285,0.435617190748632,-1.72319367647727));
#5303=CARTESIAN_POINT('Ctrl Pts',(90.6400926005174,0.497050741105725,-1.70528725535209));
#5304=CARTESIAN_POINT('Ctrl Pts',(90.644379141861,0.558468121714196,-1.68738554732465));
#5305=CARTESIAN_POINT('Ctrl Pts',(90.6486656832046,0.618933563499767,-1.66615689140698));
#5306=CARTESIAN_POINT('Ctrl Pts',(90.6529522245482,0.678068587108382,-1.64173294225244));
#5307=CARTESIAN_POINT('Ctrl Pts',(90.6572391736718,0.737209236249965,-1.6173066696401));
#5308=CARTESIAN_POINT('Ctrl Pts',(90.6615261227954,0.795018752432631,-1.58968469543067));
#5309=CARTESIAN_POINT('Ctrl Pts',(90.665813071919,0.851139090974467,-1.55904660299657));
#5310=CARTESIAN_POINT('Ctrl Pts',(90.6701046721401,0.907320316911708,-1.52837526996384));
#5311=CARTESIAN_POINT('Ctrl Pts',(90.6743962723612,0.961808267680585,-1.49468153315526));
#5312=CARTESIAN_POINT('Ctrl Pts',(90.6786878725823,1.01427103013557,-1.45819009046411));
#5313=CARTESIAN_POINT('Ctrl Pts',(90.6829822939531,1.06676827979854,-1.42167465955894));
#5314=CARTESIAN_POINT('Ctrl Pts',(90.687276715324,1.11723729617056,-1.38235817295531));
#5315=CARTESIAN_POINT('Ctrl Pts',(90.6915711366948,1.16537893228083,-1.34050587715832));
#5316=CARTESIAN_POINT('Ctrl Pts',(90.6958726801322,1.21360040870171,-1.29858417158289));
#5317=CARTESIAN_POINT('Ctrl Pts',(90.7001742235696,1.25948644666761,-1.25411861877814));
#5318=CARTESIAN_POINT('Ctrl Pts',(90.704475767007,1.3027753085361,-1.20741068322616));
#5319=CARTESIAN_POINT('Ctrl Pts',(90.705424526918,1.31232321554433,-1.19710865619317));
#5320=CARTESIAN_POINT('Ctrl Pts',(90.7063732868289,1.32174493585239,-1.18669766337584));
#5321=CARTESIAN_POINT('Ctrl Pts',(90.7073220467399,1.33103793858093,-1.1761811376477));
#5322=CARTESIAN_POINT('Ctrl Pts',(90.7116269592798,1.37320410044859,-1.12846335050273));
#5323=CARTESIAN_POINT('Ctrl Pts',(90.7159318718197,1.41288366859533,-1.0783816722617));
#5324=CARTESIAN_POINT('Ctrl Pts',(90.7202367843596,1.44980187306361,-1.02622540962561));
#5325=CARTESIAN_POINT('Ctrl Pts',(90.7245356918203,1.48666857898457,-0.974141901658876));
#5326=CARTESIAN_POINT('Ctrl Pts',(90.7288345992809,1.52078127230915,-0.919989954391084));
#5327=CARTESIAN_POINT('Ctrl Pts',(90.7331335067416,1.55190447100271,-0.8640929205715));
#5328=CARTESIAN_POINT('Ctrl Pts',(90.7374279508293,1.58299535580106,-0.808253922267861));
#5329=CARTESIAN_POINT('Ctrl Pts',(90.7417223949169,1.61110266111203,-0.750673868712587));
#5330=CARTESIAN_POINT('Ctrl Pts',(90.7460168390046,1.63603450473893,-0.691704533600605));
#5331=CARTESIAN_POINT('Ctrl Pts',(90.7503089529768,1.66095282063736,-0.63276719456425));
#5332=CARTESIAN_POINT('Ctrl Pts',(90.7546010669491,1.68269889395222,-0.57244252918758));
#5333=CARTESIAN_POINT('Ctrl Pts',(90.7588931809213,1.70112787033456,-0.511104716541551));
#5334=CARTESIAN_POINT('Ctrl Pts',(90.7631839204141,1.71955094513826,-0.44978654632802));
#5335=CARTESIAN_POINT('Ctrl Pts',(90.767474659907,1.73465889208006,-0.387456354892826));
#5336=CARTESIAN_POINT('Ctrl Pts',(90.7717653993998,1.74635655767869,-0.32450398449422));
#5337=CARTESIAN_POINT('Ctrl Pts',(90.776057765654,1.75805865824954,-0.261527746768321));
#5338=CARTESIAN_POINT('Ctrl Pts',(90.7803501319082,1.766347806312,-0.197929353333886));
#5339=CARTESIAN_POINT('Ctrl Pts',(90.7846424981625,1.77118015857365,-0.134107823690546));
#5340=CARTESIAN_POINT('Ctrl Pts',(90.7865809471856,1.7733624673438,-0.105285776719741));
#5341=CARTESIAN_POINT('Ctrl Pts',(90.7885193962088,1.77484047957058,-0.0764182946841652));
#5342=CARTESIAN_POINT('Ctrl Pts',(90.790457845232,1.77561363837197,-0.0475422940912425));
#5343=CARTESIAN_POINT('Origin',(88.3562164250559,0.,0.));
#5344=CARTESIAN_POINT('',(91.6892085678292,1.77561362793331,-0.0475426839535425));
#5345=CARTESIAN_POINT('',(91.5405159974736,1.77561363837197,-0.0475422940912406));
#5346=CARTESIAN_POINT('',(88.3562164250559,1.77561363837197,-0.0475422940912398));
#5347=CARTESIAN_POINT('Ctrl Pts',(91.6892085678292,1.77561362793331,-0.0475426839535299));
#5348=CARTESIAN_POINT('Ctrl Pts',(91.68325628541,1.77340527983042,-0.130019579674131));
#5349=CARTESIAN_POINT('Ctrl Pts',(91.6771948219063,1.76545186668815,-0.212286424862139));
#5350=CARTESIAN_POINT('Ctrl Pts',(91.6656640609989,1.739318000267,-0.368140712732106));
#5351=CARTESIAN_POINT('Ctrl Pts',(91.6602047775528,1.72211467929499,-0.441676596123442));
#5352=CARTESIAN_POINT('Ctrl Pts',(91.6539885632293,1.69628166439824,-0.527147058730273));
#5353=CARTESIAN_POINT('Ctrl Pts',(91.6530325290953,1.69212377798698,-0.540344941896463));
#5354=CARTESIAN_POINT('Ctrl Pts',(91.6515411317898,1.68533810343189,-0.56103704525579));
#5355=CARTESIAN_POINT('Ctrl Pts',(91.6510001825116,1.68281366442813,-0.56856421453817));
#5356=CARTESIAN_POINT('Ctrl Pts',(91.6499745130515,1.67790451646542,-0.582882748657257));
#5357=CARTESIAN_POINT('Ctrl Pts',(91.6494893232398,1.67552889504532,-0.589676851045445));
#5358=CARTESIAN_POINT('Ctrl Pts',(91.6483177900537,1.66966431465331,-0.606127507070891));
#5359=CARTESIAN_POINT('Ctrl Pts',(91.6476339089797,1.66613273688137,-0.615768783062606));
#5360=CARTESIAN_POINT('Ctrl Pts',(91.64566887427,1.65567799621406,-0.643561826727751));
#5361=CARTESIAN_POINT('Ctrl Pts',(91.6443992182078,1.64854017658055,-0.661631930473293));
#5362=CARTESIAN_POINT('Ctrl Pts',(91.6347123104552,1.59124515305282,-0.799992338117911));
#5363=CARTESIAN_POINT('Ctrl Pts',(91.6268719473405,1.52827686563687,-0.914563967965044));
#5364=CARTESIAN_POINT('Ctrl Pts',(91.6136132141823,1.40461194741173,-1.09055469943526));
#5365=CARTESIAN_POINT('Ctrl Pts',(91.6083298694113,1.35100106874289,-1.15630360631929));
#5366=CARTESIAN_POINT('Ctrl Pts',(91.6011996568442,1.27524070565146,-1.23672511068899));
#5367=CARTESIAN_POINT('Ctrl Pts',(91.5995214372892,1.2571690836017,-1.2550910891414));
#5368=CARTESIAN_POINT('Ctrl Pts',(91.5968758150981,1.22835895390123,-1.2831238175237));
#5369=CARTESIAN_POINT('Ctrl Pts',(91.5959204085836,1.21789069629355,-1.29306406720859));
#5370=CARTESIAN_POINT('Ctrl Pts',(91.5941261064355,1.19812009984183,-1.31138438766517));
#5371=CARTESIAN_POINT('Ctrl Pts',(91.5932886316958,1.18884800960429,-1.31979588651493));
#5372=CARTESIAN_POINT('Ctrl Pts',(91.5914015343876,1.16786152965186,-1.33843389769051));
#5373=CARTESIAN_POINT('Ctrl Pts',(91.5903497251235,1.15610032891292,-1.3486058925982));
#5374=CARTESIAN_POINT('Ctrl Pts',(91.5876268503027,1.12549897368901,-1.37437781477037));
#5375=CARTESIAN_POINT('Ctrl Pts',(91.5859465971801,1.10646794060709,-1.38974490836504));
#5376=CARTESIAN_POINT('Ctrl Pts',(91.5764062045671,0.997632662000477,-1.47397397833268));
#5377=CARTESIAN_POINT('Ctrl Pts',(91.5682329767863,0.901739363217165,-1.53451244803781));
#5378=CARTESIAN_POINT('Ctrl Pts',(91.554322965559,0.731846480293256,-1.62031628804731));
#5379=CARTESIAN_POINT('Ctrl Pts',(91.5486579448799,0.660736790177042,-1.65059139542308));
#5380=CARTESIAN_POINT('Ctrl Pts',(91.5412435054073,0.563179575514897,-1.68480800715479));
#5381=CARTESIAN_POINT('Ctrl Pts',(91.5393821972104,0.538288791631596,-1.69292485842697));
#5382=CARTESIAN_POINT('Ctrl Pts',(91.5362184024868,0.495153533447352,-1.70594355812178));
#5383=CARTESIAN_POINT('Ctrl Pts',(91.5349050294414,0.476993896868415,-1.71110997272856));
#5384=CARTESIAN_POINT('Ctrl Pts',(91.5329908063195,0.45010301649039,-1.71829902345869));
#5385=CARTESIAN_POINT('Ctrl Pts',(91.5323783561629,0.441433967087397,-1.72054651808009));
#5386=CARTESIAN_POINT('Ctrl Pts',(91.5312899581227,0.425904048984359,-1.7244476216172));
#5387=CARTESIAN_POINT('Ctrl Pts',(91.5308126637137,0.419049919768289,-1.72612601749346));
#5388=CARTESIAN_POINT('Ctrl Pts',(91.5297477268693,0.403658645439486,-1.72979785149007));
#5389=CARTESIAN_POINT('Ctrl Pts',(91.5291613398985,0.395116552877595,-1.73176898771762));
#5390=CARTESIAN_POINT('Ctrl Pts',(91.5273891262743,0.369108930696934,-1.73756793820439));
#5391=CARTESIAN_POINT('Ctrl Pts',(91.5262139131143,0.351599288526059,-1.74119549246946));
#5392=CARTESIAN_POINT('Ctrl Pts',(91.5187779355657,0.239367849530657,-1.76268486340317));
#5393=CARTESIAN_POINT('Ctrl Pts',(91.5128506571035,0.143367824799995,-1.77307789274259));
#5394=CARTESIAN_POINT('Ctrl Pts',(91.5039892872169,-0.000898945261336359,
-1.77689562584708));
#5395=CARTESIAN_POINT('Ctrl Pts',(91.5010545382994,-0.0488175700636594,
-1.77622510462011));
#5396=CARTESIAN_POINT('Ctrl Pts',(91.4946268280648,-0.152664113404289,-1.77056619554675));
#5397=CARTESIAN_POINT('Ctrl Pts',(91.4911275415671,-0.208498793042176,-1.76486219064826));
#5398=CARTESIAN_POINT('Ctrl Pts',(91.4851029702985,-0.302123060112933,-1.75079252383094));
#5399=CARTESIAN_POINT('Ctrl Pts',(91.4826165786719,-0.340079450461037,-1.74381720044289));
#5400=CARTESIAN_POINT('Ctrl Pts',(91.4789925820975,-0.39418470360664,-1.73204054912488));
#5401=CARTESIAN_POINT('Ctrl Pts',(91.4778864894195,-0.410540879112052,-1.72823673114892));
#5402=CARTESIAN_POINT('Ctrl Pts',(91.4759336992656,-0.439124984767491,-1.72116050231054));
#5403=CARTESIAN_POINT('Ctrl Pts',(91.4750902738271,-0.451376621301081,-1.71798817181518));
#5404=CARTESIAN_POINT('Ctrl Pts',(91.4733227598521,-0.476849105852667,-1.7111012713601));
#5405=CARTESIAN_POINT('Ctrl Pts',(91.4723979754407,-0.490062823043254,-1.70736376956547));
#5406=CARTESIAN_POINT('Ctrl Pts',(91.4699522123687,-0.524702023403014,-1.69713083162884));
#5407=CARTESIAN_POINT('Ctrl Pts',(91.4684231114339,-0.546049749338592,-1.69038305253282));
#5408=CARTESIAN_POINT('Ctrl Pts',(91.4598472669505,-0.664021746462519,-1.65062553606843));
#5409=CARTESIAN_POINT('Ctrl Pts',(91.4525425847481,-0.757772088670623,-1.6097405652619));
#5410=CARTESIAN_POINT('Ctrl Pts',(91.4395751305044,-0.914278512007832,-1.52477414275634));
#5411=CARTESIAN_POINT('Ctrl Pts',(91.4339870529958,-0.978680957397881,-1.48425907131499));
#5412=CARTESIAN_POINT('Ctrl Pts',(91.4243598080906,-1.08629701772805,-1.40650081682382));
#5413=CARTESIAN_POINT('Ctrl Pts',(91.4202933304705,-1.13068906222673,-1.37106867932037));
#5414=CARTESIAN_POINT('Ctrl Pts',(91.41544047149,-1.18310655990328,-1.32495023662403));
#5415=CARTESIAN_POINT('Ctrl Pts',(91.4145402132914,-1.19280635572832,-1.31622463301532));
#5416=CARTESIAN_POINT('Ctrl Pts',(91.4131158605141,-1.20812727861732,-1.30213397460057));
#5417=CARTESIAN_POINT('Ctrl Pts',(91.4125869544873,-1.21381065304967,-1.29683773600981));
#5418=CARTESIAN_POINT('Ctrl Pts',(91.4115739097267,-1.22468864055343,-1.28656656402832));
#5419=CARTESIAN_POINT('Ctrl Pts',(91.4110894104585,-1.2298880377113,-1.28159713121034));
#5420=CARTESIAN_POINT('Ctrl Pts',(91.4100081510242,-1.24148061797128,-1.27038176044984));
#5421=CARTESIAN_POINT('Ctrl Pts',(91.409412680503,-1.24785722614641,-1.2641187814425));
#5422=CARTESIAN_POINT('Ctrl Pts',(91.4073273020998,-1.27014853022522,-1.24189165564753));
#5423=CARTESIAN_POINT('Ctrl Pts',(91.405855622513,-1.28580708547034,-1.2256722342066));
#5424=CARTESIAN_POINT('Ctrl Pts',(91.396110810024,-1.38860760748972,-1.11505043636696));
#5425=CARTESIAN_POINT('Ctrl Pts',(91.3883795158571,-1.46560417354145,-1.01172173940859));
#5426=CARTESIAN_POINT('Ctrl Pts',(91.3752548001773,-1.57359407653429,-0.828244374402557));
#5427=CARTESIAN_POINT('Ctrl Pts',(91.3699915110453,-1.61116098671449,-0.752558965538474));
#5428=CARTESIAN_POINT('Ctrl Pts',(91.3628857738388,-1.65296970274245,-0.65070469174771));
#5429=CARTESIAN_POINT('Ctrl Pts',(91.3612105498061,-1.6622170174491,-0.626705601985232));
#5430=CARTESIAN_POINT('Ctrl Pts',(91.3585686509802,-1.67583282533875,-0.588945235015135));
#5431=CARTESIAN_POINT('Ctrl Pts',(91.357613918196,-1.68056032492367,-0.575316540664702));
#5432=CARTESIAN_POINT('Ctrl Pts',(91.3558203040742,-1.6890794477124,-0.549755761445475));
#5433=CARTESIAN_POINT('Ctrl Pts',(91.3549828359578,-1.69291194881462,-0.537838170486027));
#5434=CARTESIAN_POINT('Ctrl Pts',(91.3530949901467,-1.70122495963668,-0.51101842276115));
#5435=CARTESIAN_POINT('Ctrl Pts',(91.3520424163737,-1.70563620612524,-0.496096056346474));
#5436=CARTESIAN_POINT('Ctrl Pts',(91.3493159769002,-1.71648671685574,-0.457534308563045));
#5437=CARTESIAN_POINT('Ctrl Pts',(91.3476328807635,-1.72263377343176,-0.433816863644595));
#5438=CARTESIAN_POINT('Ctrl Pts',(91.3382509220641,-1.75386926627506,-0.30214259620563));
#5439=CARTESIAN_POINT('Ctrl Pts',(91.3302531026308,-1.76929733532401,-0.192164098984426));
#5440=CARTESIAN_POINT('Ctrl Pts',(91.3163927829745,-1.77799963710245,-0.00266316402731915));
#5441=CARTESIAN_POINT('Ctrl Pts',(91.3105997154047,-1.77636341355964,0.0763133267285429));
#5442=CARTESIAN_POINT('Ctrl Pts',(91.3030385347111,-1.76717134824712,0.181303064497504));
#5443=CARTESIAN_POINT('Ctrl Pts',(91.3011548010791,-1.76427178061678,0.207630941515872));
#5444=CARTESIAN_POINT('Ctrl Pts',(91.297957258132,-1.75827715092089,0.252760941122569));
#5445=CARTESIAN_POINT('Ctrl Pts',(91.2966322705087,-1.75546643206794,0.271595860918295));
#5446=CARTESIAN_POINT('Ctrl Pts',(91.2947045605403,-1.75088434100287,0.299247087075983));
#5447=CARTESIAN_POINT('Ctrl Pts',(91.2940900109151,-1.74934816937235,0.308100285283694));
#5448=CARTESIAN_POINT('Ctrl Pts',(91.2929994972425,-1.74648570135877,0.32388509355939));
#5449=CARTESIAN_POINT('Ctrl Pts',(91.2925221614057,-1.74518520717268,0.330820882871658));
#5450=CARTESIAN_POINT('Ctrl Pts',(91.2914591104128,-1.7421820362496,0.346326650217968));
#5451=CARTESIAN_POINT('Ctrl Pts',(91.2908746267797,-1.74045742961265,0.35489201151041));
#5452=CARTESIAN_POINT('Ctrl Pts',(91.2891141085383,-1.73504183467548,0.380799488248176));
#5453=CARTESIAN_POINT('Ctrl Pts',(91.2879484855765,-1.73115420626327,0.398099976343473));
#5454=CARTESIAN_POINT('Ctrl Pts',(91.2781570305158,-1.69597973471441,0.544357433338902));
#5455=CARTESIAN_POINT('Ctrl Pts',(91.2701702780981,-1.65058753120124,0.669509519818571));
#5456=CARTESIAN_POINT('Ctrl Pts',(91.2566102990108,-1.55285658995098,0.866802171358049));
#5457=CARTESIAN_POINT('Ctrl Pts',(91.251167339358,-1.50831575611698,0.942173376839766));
#5458=CARTESIAN_POINT('Ctrl Pts',(91.2438426260323,-1.44349520068649,1.0354073445338));
#5459=CARTESIAN_POINT('Ctrl Pts',(91.2421412793614,-1.42810910883382,1.05652781427212));
#5460=CARTESIAN_POINT('Ctrl Pts',(91.2394673092088,-1.40346267234034,1.08883752137705));
#5461=CARTESIAN_POINT('Ctrl Pts',(91.2385071174246,-1.39452112575662,1.10026607210096));
#5462=CARTESIAN_POINT('Ctrl Pts',(91.2367084825461,-1.37760998147121,1.12134356083809));
#5463=CARTESIAN_POINT('Ctrl Pts',(91.2358715214746,-1.36967644338061,1.13102036635003));
#5464=CARTESIAN_POINT('Ctrl Pts',(91.2339917010964,-1.3517194055667,1.15245713955055));
#5465=CARTESIAN_POINT('Ctrl Pts',(91.2329467312469,-1.34164346415074,1.16417163624273));
#5466=CARTESIAN_POINT('Ctrl Pts',(91.2302541952085,-1.31545002736335,1.19383294355072));
#5467=CARTESIAN_POINT('Ctrl Pts',(91.2285977859649,-1.29911790318704,1.21158509640262));
#5468=CARTESIAN_POINT('Ctrl Pts',(91.2183200611899,-1.19649004726787,1.31867477192972));
#5469=CARTESIAN_POINT('Ctrl Pts',(91.2093131842151,-1.10139521766226,1.39907468922928));
#5470=CARTESIAN_POINT('Ctrl Pts',(91.1951495050721,-0.941240329206732,1.50796584707608));
#5471=CARTESIAN_POINT('Ctrl Pts',(91.1900634476284,-0.881519629631283,1.54363804668006));
#5472=CARTESIAN_POINT('Ctrl Pts',(91.1824798015324,-0.787545995094066,1.59253327175776));
#5473=CARTESIAN_POINT('Ctrl Pts',(91.179904593186,-0.754720059903905,1.60834976797192));
#5474=CARTESIAN_POINT('Ctrl Pts',(91.1765889126055,-0.710972525575328,1.6277939220882));
#5475=CARTESIAN_POINT('Ctrl Pts',(91.1758016599338,-0.700471632386018,1.63234018958223));
#5476=CARTESIAN_POINT('Ctrl Pts',(91.1745133950152,-0.683087585080062,1.63966780340691));
#5477=CARTESIAN_POINT('Ctrl Pts',(91.1740090067544,-0.676229775229471,1.64250797618951));
#5478=CARTESIAN_POINT('Ctrl Pts',(91.1729960307621,-0.662348589476972,1.6481552139936));
#5479=CARTESIAN_POINT('Ctrl Pts',(91.1724875448238,-0.655324717666835,1.65096056379733));
#5480=CARTESIAN_POINT('Ctrl Pts',(91.1711728210498,-0.63702540028215,1.65813416546171));
#5481=CARTESIAN_POINT('Ctrl Pts',(91.1703706161617,-0.625722668726462,1.6624323845356));
#5482=CARTESIAN_POINT('Ctrl Pts',(91.1669913450675,-0.57757432162533,1.68018166383017));
#5483=CARTESIAN_POINT('Ctrl Pts',(91.1644712002435,-0.540329687436431,1.69252676885963));
#5484=CARTESIAN_POINT('Ctrl Pts',(91.1549497168399,-0.395966428544315,1.73512521561807));
#5485=CARTESIAN_POINT('Ctrl Pts',(91.1482288337121,-0.286498786355872,1.75652235241753));
#5486=CARTESIAN_POINT('Ctrl Pts',(91.1377540351192,-0.117647347094808,1.773310901848));
#5487=CARTESIAN_POINT('Ctrl Pts',(91.1341183055209,-0.0593063493967736,
1.7762191493932));
#5488=CARTESIAN_POINT('Ctrl Pts',(91.1279426759111,0.0378385514972737,1.77627008327119));
#5489=CARTESIAN_POINT('Ctrl Pts',(91.1254469392346,0.0765962020687426,1.77502108118855));
#5490=CARTESIAN_POINT('Ctrl Pts',(91.1218934589584,0.130831531399746,1.77149373431687));
#5491=CARTESIAN_POINT('Ctrl Pts',(91.1208684531434,0.146368804344909,1.77027768668389));
#5492=CARTESIAN_POINT('Ctrl Pts',(91.1189885391545,0.174655352231179,1.76768887241048));
#5493=CARTESIAN_POINT('Ctrl Pts',(91.1181357491288,0.187409717095556,1.766382185413));
#5494=CARTESIAN_POINT('Ctrl Pts',(91.1163992235073,0.213217444564372,1.76345552157812));
#5495=CARTESIAN_POINT('Ctrl Pts',(91.1155153136268,0.226269170032844,1.76182839736807));
#5496=CARTESIAN_POINT('Ctrl Pts',(91.1133044939307,0.258695953653458,1.75741957744828));
#5497=CARTESIAN_POINT('Ctrl Pts',(91.1119721298375,0.27804496306384,1.75446234288203));
#5498=CARTESIAN_POINT('Ctrl Pts',(91.1065089780794,0.35657188779343,1.74112895975894));
#5499=CARTESIAN_POINT('Ctrl Pts',(91.1022953651592,0.415248285640318,1.7280743590951));
#5500=CARTESIAN_POINT('Ctrl Pts',(91.0903970120789,0.5758756093973,1.68368372478917));
#5501=CARTESIAN_POINT('Ctrl Pts',(91.0825617078658,0.675835764470835,1.64610632770786));
#5502=CARTESIAN_POINT('Ctrl Pts',(91.0695174860263,0.836954003363458,1.56837586327051));
#5503=CARTESIAN_POINT('Ctrl Pts',(91.0642904728375,0.900120941813972,1.53299687225567));
#5504=CARTESIAN_POINT('Ctrl Pts',(91.0582809446137,0.972700704378237,1.48630827231153));
#5505=CARTESIAN_POINT('Ctrl Pts',(91.0573161886683,0.98435225478397,1.4786174656265));
#5506=CARTESIAN_POINT('Ctrl Pts',(91.0558143004754,1.00250830764549,1.46632350107263));
#5507=CARTESIAN_POINT('Ctrl Pts',(91.0552714575822,1.00907429237472,1.46181277714816));
#5508=CARTESIAN_POINT('Ctrl Pts',(91.0542448711953,1.02150251479465,1.45315114961383));
#5509=CARTESIAN_POINT('Ctrl Pts',(91.0537606301867,1.02737018147873,1.44900868295922));
#5510=CARTESIAN_POINT('Ctrl Pts',(91.0525947347182,1.04150636499295,1.4388997585303));
#5511=CARTESIAN_POINT('Ctrl Pts',(91.0519154884229,1.04974908386172,1.43289737830857));
#5512=CARTESIAN_POINT('Ctrl Pts',(91.049490915183,1.07917481155081,1.41107923696332));
#5513=CARTESIAN_POINT('Ctrl Pts',(91.0477708046864,1.10005695092557,1.39486120083402));
#5514=CARTESIAN_POINT('Ctrl Pts',(91.0433798112992,1.15310357586009,1.35173011637927));
#5515=CARTESIAN_POINT('Ctrl Pts',(91.0407437027549,1.18469194591766,1.32413277723071));
#5516=CARTESIAN_POINT('Ctrl Pts',(91.033182620921,1.27335849177491,1.2409531821744));
#5517=CARTESIAN_POINT('Ctrl Pts',(91.0283364725427,1.32771218119164,1.18261899326054));
#5518=CARTESIAN_POINT('Ctrl Pts',(91.0176851014514,1.43681503705992,1.04848629623619));
#5519=CARTESIAN_POINT('Ctrl Pts',(91.0118703603176,1.48986548204182,0.971626809387183));
#5520=CARTESIAN_POINT('Ctrl Pts',(91.0043853027762,1.54776151583363,0.871774298212982));
#5521=CARTESIAN_POINT('Ctrl Pts',(91.0029349227798,1.55852746200069,0.852377976876884));
#5522=CARTESIAN_POINT('Ctrl Pts',(91.0005690621447,1.57534170156359,0.820700787354758));
#5523=CARTESIAN_POINT('Ctrl Pts',(90.9996616588206,1.58161642527279,0.808542345587602));
#5524=CARTESIAN_POINT('Ctrl Pts',(90.9979051086482,1.59342496061709,0.784997579750812));
#5525=CARTESIAN_POINT('Ctrl Pts',(90.9970567294771,1.59897874729834,0.773622166591484));
#5526=CARTESIAN_POINT('Ctrl Pts',(90.9950677135531,1.61164926206272,0.746950677830628));
#5527=CARTESIAN_POINT('Ctrl Pts',(90.9939238577632,1.61867049308735,0.731610866155257));
#5528=CARTESIAN_POINT('Ctrl Pts',(90.99010256062,1.64124382480983,0.680377050511052));
#5529=CARTESIAN_POINT('Ctrl Pts',(90.9873929470631,1.65582772611047,0.644071695454346));
#5530=CARTESIAN_POINT('Ctrl Pts',(90.9806271430366,1.68877199748613,0.553524910304817));
#5531=CARTESIAN_POINT('Ctrl Pts',(90.9765320167168,1.70573012229351,0.498823001959849));
#5532=CARTESIAN_POINT('Ctrl Pts',(90.9696910017619,1.72931567533396,0.407331467129618));
#5533=CARTESIAN_POINT('Ctrl Pts',(90.9669753030179,1.73747712635044,0.370978061596516));
#5534=CARTESIAN_POINT('Ctrl Pts',(90.9565242822811,1.76439780659845,0.230537233790908));
#5535=CARTESIAN_POINT('Ctrl Pts',(90.9487490797319,1.77499312743169,0.125100087455849));
#5536=CARTESIAN_POINT('Ctrl Pts',(90.9401102254816,1.77633543066197,0.00182430299203653));
#5537=CARTESIAN_POINT('Ctrl Pts',(90.9388935730831,1.7762670550413,-0.015693861606117));
#5538=CARTESIAN_POINT('Ctrl Pts',(90.9373616027383,1.7758501855836,-0.0379870968353825));
#5539=CARTESIAN_POINT('Ctrl Pts',(90.9370342299329,1.77574155328481,-0.042764917060308));
#5540=CARTESIAN_POINT('Ctrl Pts',(90.9367078804579,1.77561363837187,-0.0475422940950947));
#5541=CARTESIAN_POINT('',(90.9812164249928,0.00152582238372352,1.77624934464901));
#5542=CARTESIAN_POINT('Ctrl Pts',(90.790457845232,1.77561363837197,-0.0475422940912425));
#5543=CARTESIAN_POINT('Ctrl Pts',(90.7947551663863,1.77732764355503,0.0164725170880728));
#5544=CARTESIAN_POINT('Ctrl Pts',(90.7990524875405,1.77557414327281,0.0805287757352375));
#5545=CARTESIAN_POINT('Ctrl Pts',(90.8033498086948,1.7703849040683,0.144226744909051));
#5546=CARTESIAN_POINT('Ctrl Pts',(90.807655136144,1.76518599684554,0.208043389114973));
#5547=CARTESIAN_POINT('Ctrl Pts',(90.8119604635933,1.75653863148026,0.271499911855457));
#5548=CARTESIAN_POINT('Ctrl Pts',(90.8162657910424,1.7445262204379,0.334204022574007));
#5549=CARTESIAN_POINT('Ctrl Pts',(90.819668114948,1.735033304107,0.383756512457684));
#5550=CARTESIAN_POINT('Ctrl Pts',(90.8230704388535,1.72343993306419,0.43283922549068));
#5551=CARTESIAN_POINT('Ctrl Pts',(90.826472762759,1.70980912878435,0.481265836753137));
#5552=CARTESIAN_POINT('Ctrl Pts',(90.830767001692,1.69260502592648,0.542387424600279));
#5553=CARTESIAN_POINT('Ctrl Pts',(90.835061240625,1.67208360227967,0.602712333521105));
#5554=CARTESIAN_POINT('Ctrl Pts',(90.839355479558,1.64833651614558,0.661854056451308));
#5555=CARTESIAN_POINT('Ctrl Pts',(90.8437833128588,1.62385065487345,0.722835686571596));
#5556=CARTESIAN_POINT('Ctrl Pts',(90.8482111461596,1.59593513686523,0.782558742003975));
#5557=CARTESIAN_POINT('Ctrl Pts',(90.8526389794605,1.56474685617675,0.840613667855199));
#5558=CARTESIAN_POINT('Ctrl Pts',(90.8569212506853,1.53458386948086,0.896760076615978));
#5559=CARTESIAN_POINT('Ctrl Pts',(90.8612035219102,1.50136022647957,0.951345849076749));
#5560=CARTESIAN_POINT('Ctrl Pts',(90.865485793135,1.46526665824609,1.00402075811825));
#5561=CARTESIAN_POINT('Ctrl Pts',(90.8697654007131,1.42919554083589,1.05666290245588));
#5562=CARTESIAN_POINT('Ctrl Pts',(90.8740450082913,1.39025832290734,1.1073961244502));
#5563=CARTESIAN_POINT('Ctrl Pts',(90.8783246158694,1.34869001932574,1.15589761409527));
#5564=CARTESIAN_POINT('Ctrl Pts',(90.8826031111121,1.30713251998172,1.20438649746172));
#5565=CARTESIAN_POINT('Ctrl Pts',(90.8868816063548,1.26294562097733,1.25064441647907));
#5566=CARTESIAN_POINT('Ctrl Pts',(90.8911601015975,1.21640447789817,1.29438178627841));
#5567=CARTESIAN_POINT('Ctrl Pts',(90.8954390339994,1.16985857943503,1.33812362498362));
#5568=CARTESIAN_POINT('Ctrl Pts',(90.8997179664013,1.12095832981624,1.37934405987335));
#5569=CARTESIAN_POINT('Ctrl Pts',(90.9039968988031,1.07001410762691,1.41779190009655));
#5570=CARTESIAN_POINT('Ctrl Pts',(90.9082805777271,1.01901337417435,1.45628238963161));
#5571=CARTESIAN_POINT('Ctrl Pts',(90.912564256651,0.965964549780858,1.4919938455216));
#5572=CARTESIAN_POINT('Ctrl Pts',(90.916847935575,0.911208309015228,1.52471750828854));
#5573=CARTESIAN_POINT('Ctrl Pts',(90.9211344824345,0.856415408785725,1.55746307964373));
#5574=CARTESIAN_POINT('Ctrl Pts',(90.9254210292941,0.799913265220529,1.58721664419762));
#5575=CARTESIAN_POINT('Ctrl Pts',(90.9297075761536,0.742065909822544,1.61381605146908));
#5576=CARTESIAN_POINT('Ctrl Pts',(90.9340013842004,0.684120564016517,1.64046051675147));
#5577=CARTESIAN_POINT('Ctrl Pts',(90.9382951922471,0.62482593063744,1.6639399843529));
#5578=CARTESIAN_POINT('Ctrl Pts',(90.9425890002939,0.564563525786503,1.68414135031817));
#5579=CARTESIAN_POINT('Ctrl Pts',(90.943600493122,0.550367504528681,1.68890018829335));
#5580=CARTESIAN_POINT('Ctrl Pts',(90.94461198595,0.536117828318496,1.69347733604087));
#5581=CARTESIAN_POINT('Ctrl Pts',(90.9456234787781,0.52181956461287,1.69787172792506));
#5582=CARTESIAN_POINT('Ctrl Pts',(90.9508792364086,0.447525208302705,1.72070516582578));
#5583=CARTESIAN_POINT('Ctrl Pts',(90.956134994039,0.371672095356916,1.73867619936979));
#5584=CARTESIAN_POINT('Ctrl Pts',(90.9613907516695,0.294836286418164,1.75160943897638));
#5585=CARTESIAN_POINT('Ctrl Pts',(90.9665711570939,0.219102078450892,1.76435725372037));
#5586=CARTESIAN_POINT('Ctrl Pts',(90.9717515625183,0.1424131311743,1.77221064472054));
#5587=CARTESIAN_POINT('Ctrl Pts',(90.9769319679427,0.0653420109390083,1.77504774135978));
#5588=CARTESIAN_POINT('Ctrl Pts',(90.9783601202927,0.0440947740017713,1.77582988211917));
#5589=CARTESIAN_POINT('Ctrl Pts',(90.9797882726427,0.0228186163093154,1.77623105384898));
#5590=CARTESIAN_POINT('Ctrl Pts',(90.9812164249928,0.00152582238372707,
1.77624934464901));
#5591=CARTESIAN_POINT('Ctrl Pts',(90.9812164250559,0.00152582144218705,
1.77624934464982));
#5592=CARTESIAN_POINT('Ctrl Pts',(90.9854749319705,-0.0619656612165415,
1.77630388466468));
#5593=CARTESIAN_POINT('Ctrl Pts',(90.9897334388851,-0.125518642809964,1.77294990638981));
#5594=CARTESIAN_POINT('Ctrl Pts',(90.9939919457997,-0.188737306903355,1.76619429607359));
#5595=CARTESIAN_POINT('Ctrl Pts',(90.9982487764536,-0.251931086463013,1.75944134494378));
#5596=CARTESIAN_POINT('Ctrl Pts',(91.0025056071076,-0.314790302202684,1.74928947146205));
#5597=CARTESIAN_POINT('Ctrl Pts',(91.0067624377615,-0.376923173624967,1.73579750653251));
#5598=CARTESIAN_POINT('Ctrl Pts',(91.0110191723997,-0.439054643597801,1.72230584592348));
#5599=CARTESIAN_POINT('Ctrl Pts',(91.0152759070379,-0.500459303301463,1.70547435420072));
#5600=CARTESIAN_POINT('Ctrl Pts',(91.0195326416762,-0.560756541552351,1.6854127576372));
#5601=CARTESIAN_POINT('Ctrl Pts',(91.023793808635,-0.621116564241113,1.66533027195671));
#5602=CARTESIAN_POINT('Ctrl Pts',(91.0280549755938,-0.680366378618047,1.64201113055681));
#5603=CARTESIAN_POINT('Ctrl Pts',(91.0323161425526,-0.738142707939781,1.61561425012759));
#5604=CARTESIAN_POINT('Ctrl Pts',(91.036579751792,-0.795952151666422,1.58920224037123));
#5605=CARTESIAN_POINT('Ctrl Pts',(91.0408433610314,-0.852285977784346,1.55970921940593));
#5606=CARTESIAN_POINT('Ctrl Pts',(91.0451069702709,-0.906805755943714,1.5273399698454));
#5607=CARTESIAN_POINT('Ctrl Pts',(91.0493782819981,-0.961424027633953,1.49491224312689));
#5608=CARTESIAN_POINT('Ctrl Pts',(91.0536495937254,-1.01422128714294,1.45959820236663));
#5609=CARTESIAN_POINT('Ctrl Pts',(91.0579209054526,-1.06488920516866,1.42164518893262));
#5610=CARTESIAN_POINT('Ctrl Pts',(91.0602053352342,-1.0919879767638,1.40134674205597));
#5611=CARTESIAN_POINT('Ctrl Pts',(91.0624897650158,-1.11847824373169,1.38029410984162));
#5612=CARTESIAN_POINT('Ctrl Pts',(91.0647741947973,-1.14431715305377,1.35852946811135));
#5613=CARTESIAN_POINT('Ctrl Pts',(91.0690737655509,-1.19294907850031,1.31756580277999));
#5614=CARTESIAN_POINT('Ctrl Pts',(91.0733733363045,-1.23947723262404,1.27390443676415));
#5615=CARTESIAN_POINT('Ctrl Pts',(91.0776729070581,-1.28358730356138,1.22778976076363));
#5616=CARTESIAN_POINT('Ctrl Pts',(91.0821000738813,-1.3290064055644,1.18030656410139));
#5617=CARTESIAN_POINT('Ctrl Pts',(91.0865272407046,-1.37186114746335,1.13022239935008));
#5618=CARTESIAN_POINT('Ctrl Pts',(91.0909544075278,-1.41184454676913,1.07784926509149));
#5619=CARTESIAN_POINT('Ctrl Pts',(91.0952422023726,-1.45056922561345,1.02712489349108));
#5620=CARTESIAN_POINT('Ctrl Pts',(91.0995299972175,-1.48660034009003,0.974253971554576));
#5621=CARTESIAN_POINT('Ctrl Pts',(91.1038177920623,-1.51969766000126,0.919555917107115));
#5622=CARTESIAN_POINT('Ctrl Pts',(91.1081029792507,-1.55277485151513,0.864891127714878));
#5623=CARTESIAN_POINT('Ctrl Pts',(91.112388166439,-1.58292152656567,0.808401839493629));
#5624=CARTESIAN_POINT('Ctrl Pts',(91.1166733536274,-1.60994076449013,0.750436404589313));
#5625=CARTESIAN_POINT('Ctrl Pts',(91.1209574757118,-1.63695328665184,0.692485377275248));
#5626=CARTESIAN_POINT('Ctrl Pts',(91.1252415977961,-1.66083970214394,0.633059387996253));
#5627=CARTESIAN_POINT('Ctrl Pts',(91.1295257198804,-1.68144995841518,0.572529562420654));
#5628=CARTESIAN_POINT('Ctrl Pts',(91.1338103176526,-1.70206250314828,0.511993015909827));
#5629=CARTESIAN_POINT('Ctrl Pts',(91.1380949154249,-1.71939800743963,0.450352867635421));
#5630=CARTESIAN_POINT('Ctrl Pts',(91.1423795131971,-1.73335594783436,0.387996418291795));
#5631=CARTESIAN_POINT('Ctrl Pts',(91.1466688784554,-1.74732941927524,0.325570584722028));
#5632=CARTESIAN_POINT('Ctrl Pts',(91.1509582437136,-1.75791772080779,0.262427352657418));
#5633=CARTESIAN_POINT('Ctrl Pts',(91.1552476089719,-1.76507149025372,0.198964059049623));
#5634=CARTESIAN_POINT('Ctrl Pts',(91.1595398611743,-1.77223007452218,0.135458051667291));
#5635=CARTESIAN_POINT('Ctrl Pts',(91.1638321133766,-1.77594949939217,0.0716320567027389));
#5636=CARTESIAN_POINT('Ctrl Pts',(91.168124365579,-1.77623249677777,0.00788542266422285));
#5637=CARTESIAN_POINT('Ctrl Pts',(91.1724238554985,-1.77651597136158,-0.0559687027535952));
#5638=CARTESIAN_POINT('Ctrl Pts',(91.1767233454181,-1.77335148746199,-0.119742698575047));
#5639=CARTESIAN_POINT('Ctrl Pts',(91.1810228353376,-1.76679366480799,-0.183041548546642));
#5640=CARTESIAN_POINT('Ctrl Pts',(91.1819901938306,-1.76531819549464,-0.197283396127977));
#5641=CARTESIAN_POINT('Ctrl Pts',(91.1829575523235,-1.7636711524572,-0.211501233370493));
#5642=CARTESIAN_POINT('Ctrl Pts',(91.1839249108164,-1.76185351127122,-0.225690645178881));
#5643=CARTESIAN_POINT('Ctrl Pts',(91.1882231241585,-1.75377728135864,-0.288737715729961));
#5644=CARTESIAN_POINT('Ctrl Pts',(91.1925213375006,-1.74229612461739,-0.351479443022377));
#5645=CARTESIAN_POINT('Ctrl Pts',(91.1968195508426,-1.72744485579698,-0.413519446556672));
#5646=CARTESIAN_POINT('Ctrl Pts',(91.2012468873423,-1.71214743817654,-0.477423201496006));
#5647=CARTESIAN_POINT('Ctrl Pts',(91.2056742238421,-1.69327413474614,-0.540581848403752));
#5648=CARTESIAN_POINT('Ctrl Pts',(91.2101015603418,-1.67092064643609,-0.60256805077403));
#5649=CARTESIAN_POINT('Ctrl Pts',(91.2143879366153,-1.64927886205207,-0.662580698816891));
#5650=CARTESIAN_POINT('Ctrl Pts',(91.2186743128888,-1.62437536707959,-0.72149392708246));
#5651=CARTESIAN_POINT('Ctrl Pts',(91.2229606891622,-1.59634820683966,-0.778932901487549));
#5652=CARTESIAN_POINT('Ctrl Pts',(91.2272444390262,-1.56833821980045,-0.836336681066321));
#5653=CARTESIAN_POINT('Ctrl Pts',(91.2315281888903,-1.53720858364255,-0.892267546083985));
#5654=CARTESIAN_POINT('Ctrl Pts',(91.2358119387542,-1.50314513970486,-0.946371360239546));
#5655=CARTESIAN_POINT('Ctrl Pts',(91.2400946070401,-1.46909029624063,-1.00046151404948));
#5656=CARTESIAN_POINT('Ctrl Pts',(91.2443772753259,-1.43210338390166,-1.05272510635283));
#5657=CARTESIAN_POINT('Ctrl Pts',(91.2486599436117,-1.3924147911509,-1.10283503384875));
#5658=CARTESIAN_POINT('Ctrl Pts',(91.2529430733713,-1.35272192180399,-1.15295036087911));
#5659=CARTESIAN_POINT('Ctrl Pts',(91.2572262031309,-1.31032710974795,-1.20091116947056));
#5660=CARTESIAN_POINT('Ctrl Pts',(91.2615093328904,-1.26550118595883,-1.24642320695532));
#5661=CARTESIAN_POINT('Ctrl Pts',(91.2657972184817,-1.22062548909183,-1.2919857793537));
#5662=CARTESIAN_POINT('Ctrl Pts',(91.270085104073,-1.1733136507143,-1.33509379785901));
#5663=CARTESIAN_POINT('Ctrl Pts',(91.2743729896643,-1.12387266717102,-1.37549056357574));
#5664=CARTESIAN_POINT('Ctrl Pts',(91.2786637536486,-1.07439849464054,-1.41591444703253));
#5665=CARTESIAN_POINT('Ctrl Pts',(91.2829545176329,-1.02279274071359,-1.4536231603876));
#5666=CARTESIAN_POINT('Ctrl Pts',(91.2872452816171,-0.969392325396927,-1.48840269482474));
#5667=CARTESIAN_POINT('Ctrl Pts',(91.29154328421,-0.915901822462332,-1.52324090306416));
#5668=CARTESIAN_POINT('Ctrl Pts',(91.2958412868029,-0.860611055822227,-1.55513982642731));
#5669=CARTESIAN_POINT('Ctrl Pts',(91.3001392893958,-0.803881423270245,-1.58393141259999));
#5670=CARTESIAN_POINT('Ctrl Pts',(91.3011180685424,-0.790962449831687,-1.59048808713297));
#5671=CARTESIAN_POINT('Ctrl Pts',(91.302096847689,-0.777968932998481,-1.59688381334398));
#5672=CARTESIAN_POINT('Ctrl Pts',(91.3030756268356,-0.764905266538352,-1.60311696258317));
#5673=CARTESIAN_POINT('Ctrl Pts',(91.3073745691009,-0.707527718110618,-1.63049387268879));
#5674=CARTESIAN_POINT('Ctrl Pts',(91.3116735113661,-0.648561767975585,-1.65484218375743));
#5675=CARTESIAN_POINT('Ctrl Pts',(91.3159724536313,-0.588359603674145,-1.67597644352909));
#5676=CARTESIAN_POINT('Ctrl Pts',(91.3203996990156,-0.526360689154039,-1.69774146111995));
#5677=CARTESIAN_POINT('Ctrl Pts',(91.3248269443999,-0.463051030788027,-1.71609718988282));
#5678=CARTESIAN_POINT('Ctrl Pts',(91.3292541897843,-0.398841581838443,-1.73089267578802));
#5679=CARTESIAN_POINT('Ctrl Pts',(91.3335413175578,-0.336664293701429,-1.74521990029008));
#5680=CARTESIAN_POINT('Ctrl Pts',(91.3378284453313,-0.273643854694677,-1.75620876014265));
#5681=CARTESIAN_POINT('Ctrl Pts',(91.3421155731048,-0.210170241194075,-1.76377224499549));
#5682=CARTESIAN_POINT('Ctrl Pts',(91.3464000807608,-0.146735420174489,-1.77133110735519));
#5683=CARTESIAN_POINT('Ctrl Pts',(91.3506845884169,-0.0828484731931914,
-1.77546868675301));
#5684=CARTESIAN_POINT('Ctrl Pts',(91.3549690960729,-0.0189078653409894,
-1.77614936171715));
#5685=CARTESIAN_POINT('Ctrl Pts',(91.3592525272335,0.0450166772412661,-1.77682986565966));
#5686=CARTESIAN_POINT('Ctrl Pts',(91.3635359583942,0.10899435030359,-1.77405518402828));
#5687=CARTESIAN_POINT('Ctrl Pts',(91.3678193895548,0.172625282557775,-1.76784178430137));
#5688=CARTESIAN_POINT('Ctrl Pts',(91.3721032860686,0.236263127695454,-1.76162770954886));
#5689=CARTESIAN_POINT('Ctrl Pts',(91.3763871825825,0.299553656171313,-1.75197422745588));
#5690=CARTESIAN_POINT('Ctrl Pts',(91.3806710790963,0.36210270141522,-1.73894959562599));
#5691=CARTESIAN_POINT('Ctrl Pts',(91.3849597322688,0.424721198489555,-1.72591050179244));
#5692=CARTESIAN_POINT('Ctrl Pts',(91.3892483854413,0.486596076204566,-1.70949289526432));
#5693=CARTESIAN_POINT('Ctrl Pts',(91.3935370386137,0.547345140759118,-1.68981577676011));
#5694=CARTESIAN_POINT('Ctrl Pts',(91.3978285715565,0.608134997456195,-1.67012544534755));
#5695=CARTESIAN_POINT('Ctrl Pts',(91.4021201044993,0.667797067397921,-1.64717142917015));
#5696=CARTESIAN_POINT('Ctrl Pts',(91.406411637442,0.72596882539495,-1.62112100938045));
#5697=CARTESIAN_POINT('Ctrl Pts',(91.4107104040958,0.784238636393311,-1.59502667959156));
#5698=CARTESIAN_POINT('Ctrl Pts',(91.4150091707495,0.841012678882903,-1.56582576762878));
#5699=CARTESIAN_POINT('Ctrl Pts',(91.4193079374033,0.895953791088256,-1.533731028158));
#5700=CARTESIAN_POINT('Ctrl Pts',(91.4202807392204,0.908386848775099,-1.52646805638209));
#5701=CARTESIAN_POINT('Ctrl Pts',(91.4212535410375,0.920726165329498,-1.51905706017416));
#5702=CARTESIAN_POINT('Ctrl Pts',(91.4222263428547,0.932968059999427,-1.5115007977242));
#5703=CARTESIAN_POINT('Ctrl Pts',(91.4265252513526,0.987066216582616,-1.47810891842586));
#5704=CARTESIAN_POINT('Ctrl Pts',(91.4308241598505,1.03947950536856,-1.44174107480054));
#5705=CARTESIAN_POINT('Ctrl Pts',(91.4351230683485,1.08986123451802,-1.40259279621523));
#5706=CARTESIAN_POINT('Ctrl Pts',(91.4395144403953,1.14132660466173,-1.36260249254969));
#5707=CARTESIAN_POINT('Ctrl Pts',(91.4439058124422,1.19067150034813,-1.31971094349971));
#5708=CARTESIAN_POINT('Ctrl Pts',(91.4482971844891,1.23755467153794,-1.27417522243003));
#5709=CARTESIAN_POINT('Ctrl Pts',(91.4525842797451,1.28332456273594,-1.22972078502554));
#5710=CARTESIAN_POINT('Ctrl Pts',(91.4568713750012,1.32674796788167,-1.18274673913133));
#5711=CARTESIAN_POINT('Ctrl Pts',(91.4611584702572,1.3675401660274,-1.13353339465662));
#5712=CARTESIAN_POINT('Ctrl Pts',(91.4654429248555,1.40830723801461,-1.08435036338763));
#5713=CARTESIAN_POINT('Ctrl Pts',(91.4697273794537,1.44644599623708,-1.03293115604103));
#5714=CARTESIAN_POINT('Ctrl Pts',(91.474011834052,1.4817102738338,-0.979591101896785));
#5715=CARTESIAN_POINT('Ctrl Pts',(91.4782951917256,1.5169655229177,-0.926264704103836));
#5716=CARTESIAN_POINT('Ctrl Pts',(91.4825785493993,1.54934747463787,-0.871018855963951));
#5717=CARTESIAN_POINT('Ctrl Pts',(91.486861907073,1.57865294795679,-0.814198337266384));
#5718=CARTESIAN_POINT('Ctrl Pts',(91.4913330812731,1.6092434067058,-0.754886354334056));
#5719=CARTESIAN_POINT('Ctrl Pts',(91.4958042554731,1.63648104049615,-0.693858919280336));
#5720=CARTESIAN_POINT('Ctrl Pts',(91.5002754296732,1.66018901052115,-0.631535044035412));
#5721=CARTESIAN_POINT('Ctrl Pts',(91.5045639800986,1.68292863559235,-0.571756768857921));
#5722=CARTESIAN_POINT('Ctrl Pts',(91.508852530524,1.70242124843261,-0.510786427960019));
#5723=CARTESIAN_POINT('Ctrl Pts',(91.5131410809495,1.71856159337882,-0.449010147171809));
#5724=CARTESIAN_POINT('Ctrl Pts',(91.5174325578708,1.73471295245526,-0.387191710407141));
#5725=CARTESIAN_POINT('Ctrl Pts',(91.5217240347921,1.74750739301217,-0.324566733028707));
#5726=CARTESIAN_POINT('Ctrl Pts',(91.5260155117134,1.75689093212616,-0.261530715429101));
#5727=CARTESIAN_POINT('Ctrl Pts',(91.5303139690037,1.76628973418252,-0.198392165608831));
#5728=CARTESIAN_POINT('Ctrl Pts',(91.5346124262939,1.7722665268007,-0.134841742660515));
#5729=CARTESIAN_POINT('Ctrl Pts',(91.5389108835842,1.7748192920435,-0.0712779284927003));
#5730=CARTESIAN_POINT('Ctrl Pts',(91.5394459215473,1.77513704006881,-0.0633660076883157));
#5731=CARTESIAN_POINT('Ctrl Pts',(91.5399809595105,1.77540180472763,-0.0554538750348641));
#5732=CARTESIAN_POINT('Ctrl Pts',(91.5405159974736,1.77561363837197,-0.0475422940912406));
#5733=CARTESIAN_POINT('Origin',(88.3562164250559,0.,0.));
#5734=CARTESIAN_POINT('',(92.4383302476831,1.77320199105526,-0.0474633882366059));
#5735=CARTESIAN_POINT('',(92.2906253551795,1.77468168403539,-0.0475286896032536));
#5736=CARTESIAN_POINT('',(88.3562164250559,1.77561363837197,-0.0475422940912398));
#5737=CARTESIAN_POINT('',(91.8790868291566,-0.000950402920720204,1.77856749323898));
#5738=CARTESIAN_POINT('Ctrl Pts',(91.8790868291566,-0.000950402920720204,
1.77856749323898));
#5739=CARTESIAN_POINT('Ctrl Pts',(91.8827809065456,-0.0557221683725779,
1.7789218457455));
#5740=CARTESIAN_POINT('Ctrl Pts',(91.9261918892744,-0.699017003225842,1.75176962424819));
#5741=CARTESIAN_POINT('Ctrl Pts',(92.0093197773428,-1.8628457362405,0.969248007846431));
#5742=CARTESIAN_POINT('Ctrl Pts',(92.1284704933619,-1.82397533873842,-1.04055267810004));
#5743=CARTESIAN_POINT('Ctrl Pts',(92.2476212093811,-0.113688812436545,-2.09683346434928));
#5744=CARTESIAN_POINT('Ctrl Pts',(92.3509077941549,1.45919325958565,-1.34685406637966));
#5745=CARTESIAN_POINT('Ctrl Pts',(92.4144774735888,1.76180986717413,-0.403366942278606));
#5746=CARTESIAN_POINT('Ctrl Pts',(92.4383302476831,1.77320199105525,-0.0474633882366439));
#5747=CARTESIAN_POINT('Ctrl Pts',(91.8777557556434,-0.00103318020657592,
1.77624969951825));
#5748=CARTESIAN_POINT('Ctrl Pts',(91.8707368718479,0.109507008580014,1.77631399674803));
#5749=CARTESIAN_POINT('Ctrl Pts',(91.8640538279637,0.219824095479598,1.76605951654221));
#5750=CARTESIAN_POINT('Ctrl Pts',(91.8519898096994,0.412189196020058,1.72986097897984));
#5751=CARTESIAN_POINT('Ctrl Pts',(91.846680475189,0.494645281326305,1.70811082915314));
#5752=CARTESIAN_POINT('Ctrl Pts',(91.83951860179,0.599650062392536,1.67216947119991));
#5753=CARTESIAN_POINT('Ctrl Pts',(91.8378365911201,0.623896042496529,1.66327524938476));
#5754=CARTESIAN_POINT('Ctrl Pts',(91.8351863225811,0.661390960938906,1.64858569769984));
#5755=CARTESIAN_POINT('Ctrl Pts',(91.8342301316928,0.674778216568841,1.64315158873551));
#5756=CARTESIAN_POINT('Ctrl Pts',(91.832435126572,0.699637814510184,1.63270563433127));
#5757=CARTESIAN_POINT('Ctrl Pts',(91.8315977433032,0.711126414284918,1.62773461255972));
#5758=CARTESIAN_POINT('Ctrl Pts',(91.8297118721351,0.736751081864573,1.61632397214454));
#5759=CARTESIAN_POINT('Ctrl Pts',(91.8286612102891,0.750856995888474,1.60981958135189));
#5760=CARTESIAN_POINT('Ctrl Pts',(91.8259434306869,0.786899469107592,1.59262323375946));
#5761=CARTESIAN_POINT('Ctrl Pts',(91.8242671835355,0.808703643108505,1.58166300264375));
#5762=CARTESIAN_POINT('Ctrl Pts',(91.8145418753254,0.93273275792427,1.51608256608761));
#5763=CARTESIAN_POINT('Ctrl Pts',(91.8061626329232,1.0296263861501,1.45201853769499));
#5764=CARTESIAN_POINT('Ctrl Pts',(91.7921925889266,1.17798832582408,1.331566174817));
#5765=CARTESIAN_POINT('Ctrl Pts',(91.7866751450469,1.23333018416285,1.28047747329819));
#5766=CARTESIAN_POINT('Ctrl Pts',(91.7794304657962,1.30308532221069,1.2073521040174));
#5767=CARTESIAN_POINT('Ctrl Pts',(91.7775956144617,1.32049517270121,1.18828578136537));
#5768=CARTESIAN_POINT('Ctrl Pts',(91.7744717417336,1.34977891659175,1.15477704813706));
#5769=CARTESIAN_POINT('Ctrl Pts',(91.7731721720948,1.36185163924426,1.1405145051594));
#5770=CARTESIAN_POINT('Ctrl Pts',(91.7712740418605,1.37935182975643,1.11916582287923));
#5771=CARTESIAN_POINT('Ctrl Pts',(91.7706641470608,1.38495414045629,1.11222553773524));
#5772=CARTESIAN_POINT('Ctrl Pts',(91.7695783802573,1.3948944191896,1.09971969407853));
#5773=CARTESIAN_POINT('Ctrl Pts',(91.7691011916088,1.39925175680091,1.0941701750966));
#5774=CARTESIAN_POINT('Ctrl Pts',(91.7680341564229,1.40896918169565,1.08164104164261));
#5775=CARTESIAN_POINT('Ctrl Pts',(91.7674455935812,1.41431059633009,1.07464740415189));
#5776=CARTESIAN_POINT('Ctrl Pts',(91.7656596544044,1.43045248538915,1.05318363424268));
#5777=CARTESIAN_POINT('Ctrl Pts',(91.764473134501,1.44108486569628,1.03858776808788));
#5778=CARTESIAN_POINT('Ctrl Pts',(91.7577880790405,1.50031744818914,0.954613317933439));
#5779=CARTESIAN_POINT('Ctrl Pts',(91.752543651256,1.54413376610337,0.881982610982947));
#5780=CARTESIAN_POINT('Ctrl Pts',(91.7426013691406,1.61753349565499,0.737948589834908));
#5781=CARTESIAN_POINT('Ctrl Pts',(91.7379076574362,1.64797336191563,0.667207743810491));
#5782=CARTESIAN_POINT('Ctrl Pts',(91.7288392094935,1.69675312593909,0.529925381656571));
#5783=CARTESIAN_POINT('Ctrl Pts',(91.7244918029674,1.71599135168586,0.463857919493194));
#5784=CARTESIAN_POINT('Ctrl Pts',(91.7186962456932,1.73590228256272,0.376991095390475));
#5785=CARTESIAN_POINT('Ctrl Pts',(91.7173613993357,1.74011136719097,0.357059370934363));
#5786=CARTESIAN_POINT('Ctrl Pts',(91.7151362191763,1.74650257608371,0.323990753469435));
#5787=CARTESIAN_POINT('Ctrl Pts',(91.7142522013224,1.74888148861618,0.310893517115));
#5788=CARTESIAN_POINT('Ctrl Pts',(91.7125152829974,1.75324258674415,0.285247052917134));
#5789=CARTESIAN_POINT('Ctrl Pts',(91.7116628538573,1.75523778736061,0.272700833232157));
#5790=CARTESIAN_POINT('Ctrl Pts',(91.7095997191405,1.75971793371518,0.242439353121466));
#5791=CARTESIAN_POINT('Ctrl Pts',(91.7083848997398,1.76207013059135,0.224706163995916));
#5792=CARTESIAN_POINT('Ctrl Pts',(91.7042214800063,1.76916288372251,0.164241067954009));
#5793=CARTESIAN_POINT('Ctrl Pts',(91.7012335637153,1.77261940804443,0.121376792252211));
#5794=CARTESIAN_POINT('Ctrl Pts',(91.6952385851482,1.77637357342182,0.0364394768755772));
#5795=CARTESIAN_POINT('Ctrl Pts',(91.6922370670237,1.77673722724866,-0.00557874564042932));
#5796=CARTESIAN_POINT('Ctrl Pts',(91.6892085678292,1.77561362793331,-0.0475426839535299));
#5797=CARTESIAN_POINT('',(91.7312164509562,-0.000866965636682646,1.77616513543833));
#5798=CARTESIAN_POINT('Ctrl Pts',(91.5405159974736,1.77561363837197,-0.0475422940912406));
#5799=CARTESIAN_POINT('Ctrl Pts',(91.5408030179403,1.77572727627368,-0.0432981360846548));
#5800=CARTESIAN_POINT('Ctrl Pts',(91.5410900384071,1.77582568204212,-0.0390541368196787));
#5801=CARTESIAN_POINT('Ctrl Pts',(91.5413770588738,1.77590886522354,-0.0348104139653638));
#5802=CARTESIAN_POINT('Ctrl Pts',(91.5456757924709,1.77715470786581,0.0287482382035046));
#5803=CARTESIAN_POINT('Ctrl Pts',(91.549974526068,1.77498669166783,0.0925033035107822));
#5804=CARTESIAN_POINT('Ctrl Pts',(91.5542732596652,1.76938128301735,0.156057482383559));
#5805=CARTESIAN_POINT('Ctrl Pts',(91.558700531133,1.76360826516845,0.221512016010193));
#5806=CARTESIAN_POINT('Ctrl Pts',(91.5631278026008,1.75418888579952,0.286752923207428));
#5807=CARTESIAN_POINT('Ctrl Pts',(91.5675550740686,1.74115529809571,0.351343550407898));
#5808=CARTESIAN_POINT('Ctrl Pts',(91.571841988888,1.72853491087002,0.413886477569995));
#5809=CARTESIAN_POINT('Ctrl Pts',(91.5761289037074,1.71252616655278,0.475819205086708));
#5810=CARTESIAN_POINT('Ctrl Pts',(91.5804158185268,1.69321079658883,0.536750650502649));
#5811=CARTESIAN_POINT('Ctrl Pts',(91.5847001122304,1.6739072364748,0.597644841067788));
#5812=CARTESIAN_POINT('Ctrl Pts',(91.588984405934,1.65130121199289,0.657538484231631));
#5813=CARTESIAN_POINT('Ctrl Pts',(91.5932686996377,1.62552476460653,0.716053979914141));
#5814=CARTESIAN_POINT('Ctrl Pts',(91.597551916192,1.59975479788712,0.774554763738437));
#5815=CARTESIAN_POINT('Ctrl Pts',(91.6018351327464,1.5708161936863,0.831677626948991));
#5816=CARTESIAN_POINT('Ctrl Pts',(91.6061183493008,1.53888901708276,0.887065192419401));
#5817=CARTESIAN_POINT('Ctrl Pts',(91.6104020308983,1.50695837403931,0.942458771502284));
#5818=CARTESIAN_POINT('Ctrl Pts',(91.6146857124958,1.47203876905022,0.996116244024471));
#5819=CARTESIAN_POINT('Ctrl Pts',(91.6189693940932,1.43435508267371,1.04770680980325));
#5820=CARTESIAN_POINT('Ctrl Pts',(91.6232578332735,1.39662954368612,1.09935467358263));
#5821=CARTESIAN_POINT('Ctrl Pts',(91.6275462724539,1.35613409809761,1.14893064454811));
#5822=CARTESIAN_POINT('Ctrl Pts',(91.6318347116342,1.31313490030285,1.19613577661845));
#5823=CARTESIAN_POINT('Ctrl Pts',(91.6361260308787,1.27010682476358,1.24337261108821));
#5824=CARTESIAN_POINT('Ctrl Pts',(91.6404173501233,1.22457201107376,1.28823508618731));
#5825=CARTESIAN_POINT('Ctrl Pts',(91.6447086693678,1.17683246650155,1.33046210328888));
#5826=CARTESIAN_POINT('Ctrl Pts',(91.6490072246725,1.12901242309016,1.37276032395742));
#5827=CARTESIAN_POINT('Ctrl Pts',(91.6533057799772,1.07898062884179,1.41241391212508));
#5828=CARTESIAN_POINT('Ctrl Pts',(91.657604335282,1.02707003592149,1.44920364470016));
#5829=CARTESIAN_POINT('Ctrl Pts',(91.6585788151523,1.01530193611311,1.45754385467487));
#5830=CARTESIAN_POINT('Ctrl Pts',(91.6595532950226,1.00343738422584,1.46573706813981));
#5831=CARTESIAN_POINT('Ctrl Pts',(91.660527774893,0.991480433293622,1.47378106002754));
#5832=CARTESIAN_POINT('Ctrl Pts',(91.6648979419894,0.937858111141657,1.50985526714243));
#5833=CARTESIAN_POINT('Ctrl Pts',(91.6692681090858,0.88216220231501,1.54306827283372));
#5834=CARTESIAN_POINT('Ctrl Pts',(91.6736382761822,0.824724424407,1.5731794831762));
#5835=CARTESIAN_POINT('Ctrl Pts',(91.6780010643716,0.767383628608955,1.60323985156729));
#5836=CARTESIAN_POINT('Ctrl Pts',(91.6823638525609,0.70830722561498,1.63020859975998));
#5837=CARTESIAN_POINT('Ctrl Pts',(91.6867266407503,0.647855562855665,1.65388851866653));
#5838=CARTESIAN_POINT('Ctrl Pts',(91.6910823738664,0.587501656597596,1.67753014473023));
#5839=CARTESIAN_POINT('Ctrl Pts',(91.6954381069825,0.525777357976388,1.69789333956063));
#5840=CARTESIAN_POINT('Ctrl Pts',(91.6997938400986,0.463065448793341,1.71482782011309));
#5841=CARTESIAN_POINT('Ctrl Pts',(91.704145446695,0.400412951406215,1.73174625733478));
#5842=CARTESIAN_POINT('Ctrl Pts',(91.7084970532914,0.336775164611691,1.74524230409755));
#5843=CARTESIAN_POINT('Ctrl Pts',(91.7128486598878,0.272551386052349,1.75521503083267));
#5844=CARTESIAN_POINT('Ctrl Pts',(91.7171974553322,0.208369096262898,1.76518131515388));
#5845=CARTESIAN_POINT('Ctrl Pts',(91.7215462507766,0.143602042190318,1.77162872716101));
#5846=CARTESIAN_POINT('Ctrl Pts',(91.725895046221,0.0786594231437778,1.77450746903209));
#5847=CARTESIAN_POINT('Ctrl Pts',(91.7276688391659,0.0521705342173203,1.77568165440975));
#5848=CARTESIAN_POINT('Ctrl Pts',(91.7294426321109,0.0256525205454586,1.77626272710031));
#5849=CARTESIAN_POINT('Ctrl Pts',(91.7312164250558,-0.000866620254329586,
1.77624978859093));
#5850=CARTESIAN_POINT('Ctrl Pts',(91.7312171833216,-0.000876731753600045,
1.77377146193875));
#5851=CARTESIAN_POINT('Ctrl Pts',(91.7473709525184,-0.242047698959972,1.77483106190353));
#5852=CARTESIAN_POINT('Ctrl Pts',(91.8032416270549,-1.07484492687079,1.61655950001718));
#5853=CARTESIAN_POINT('Ctrl Pts',(91.8988292069313,-2.07083606885155,0.348244089557057));
#5854=CARTESIAN_POINT('Ctrl Pts',(92.0179799229503,-1.41471804329461,-1.55184057332674));
#5855=CARTESIAN_POINT('Ctrl Pts',(92.1371306389695,0.537789440227507,-2.02988107712031));
#5856=CARTESIAN_POINT('Ctrl Pts',(92.2280124497125,1.65117025021109,-0.975720506046015));
#5857=CARTESIAN_POINT('Ctrl Pts',(92.2791773551159,1.77170285356651,-0.21804953119594));
#5858=CARTESIAN_POINT('Ctrl Pts',(92.2906253551795,1.77468168403539,-0.047528689603001));
#5859=CARTESIAN_POINT('Origin',(88.3562164250559,0.,0.));
#5860=CARTESIAN_POINT('',(93.1883366943682,1.77561363837197,-0.047542294091239));
#5861=CARTESIAN_POINT('',(93.0389806716277,1.77561363837854,-0.0475422938458683));
#5862=CARTESIAN_POINT('',(88.3562164250559,1.77561363837197,-0.0475422940912398));
#5863=CARTESIAN_POINT('',(92.6290868540185,0.00157867016090192,1.77624929846588));
#5864=CARTESIAN_POINT('Ctrl Pts',(92.6290868540186,0.00157867016090192,
1.77624929846588));
#5865=CARTESIAN_POINT('Ctrl Pts',(92.6333154763636,-0.0612556274311389,
1.77630514345947));
#5866=CARTESIAN_POINT('Ctrl Pts',(92.6375440987086,-0.124197499503331,1.7730226365899));
#5867=CARTESIAN_POINT('Ctrl Pts',(92.6417727210536,-0.186857609780307,1.76639415085286));
#5868=CARTESIAN_POINT('Ctrl Pts',(92.6459976525732,-0.249463029071135,1.75977145058954));
#5869=CARTESIAN_POINT('Ctrl Pts',(92.6502225840928,-0.311786659069597,1.74980860976227));
#5870=CARTESIAN_POINT('Ctrl Pts',(92.6544475156124,-0.373440848285772,1.73655002672874));
#5871=CARTESIAN_POINT('Ctrl Pts',(92.6586703829559,-0.435064915094421,1.72329792144549));
#5872=CARTESIAN_POINT('Ctrl Pts',(92.6628932502993,-0.496019681904808,1.70675337422147));
#5873=CARTESIAN_POINT('Ctrl Pts',(92.6671161176427,-0.555926481664665,1.68701209523938));
#5874=CARTESIAN_POINT('Ctrl Pts',(92.6713385441744,-0.615827027943092,1.66727287698698));
#5875=CARTESIAN_POINT('Ctrl Pts',(92.6755609707061,-0.674679331323129,1.64433775375019));
#5876=CARTESIAN_POINT('Ctrl Pts',(92.6797833972377,-0.732120831172046,1.61835198614639));
#5877=CARTESIAN_POINT('Ctrl Pts',(92.6840098160817,-0.78961664206863,1.59234164894975));
#5878=CARTESIAN_POINT('Ctrl Pts',(92.6882362349257,-0.84569851279654,1.5632751255513));
#5879=CARTESIAN_POINT('Ctrl Pts',(92.6924626537697,-0.900026111334196,1.53134485385123));
#5880=CARTESIAN_POINT('Ctrl Pts',(92.6966912893475,-0.954382204402451,1.49939783489694));
#5881=CARTESIAN_POINT('Ctrl Pts',(92.7009199249252,-1.00698176234783,1.46458436810422));
#5882=CARTESIAN_POINT('Ctrl Pts',(92.7051485605029,-1.05751387769493,1.42713995844228));
#5883=CARTESIAN_POINT('Ctrl Pts',(92.709384550352,-1.10813387644569,1.38963042698311));
#5884=CARTESIAN_POINT('Ctrl Pts',(92.7136205402011,-1.15667885988232,1.34948115599194));
#5885=CARTESIAN_POINT('Ctrl Pts',(92.7178565300502,-1.20287236373434,1.3069667704514));
#5886=CARTESIAN_POINT('Ctrl Pts',(92.7199790445193,-1.22601840133124,1.28566421740665));
#5887=CARTESIAN_POINT('Ctrl Pts',(92.7221015589885,-1.24857465810838,1.26376841918942));
#5888=CARTESIAN_POINT('Ctrl Pts',(92.7242240734576,-1.27051017199142,1.24131702854925));
#5889=CARTESIAN_POINT('Ctrl Pts',(92.7285228830294,-1.31493700554775,1.19584537010543));
#5890=CARTESIAN_POINT('Ctrl Pts',(92.7328216926012,-1.35701005379085,1.1478930620762));
#5891=CARTESIAN_POINT('Ctrl Pts',(92.737120502173,-1.39644013775725,1.0977335761288));
#5892=CARTESIAN_POINT('Ctrl Pts',(92.7415477641439,-1.43704842903952,1.04607527842757));
#5893=CARTESIAN_POINT('Ctrl Pts',(92.7459750261149,-1.47485283271129,0.992076099468365));
#5894=CARTESIAN_POINT('Ctrl Pts',(92.7504022880859,-1.50957782884443,0.936076300929225));
#5895=CARTESIAN_POINT('Ctrl Pts',(92.7546892817189,-1.54320263765496,0.881850736379493));
#5896=CARTESIAN_POINT('Ctrl Pts',(92.7589762753519,-1.5739399715431,0.82574989835249));
#5897=CARTESIAN_POINT('Ctrl Pts',(92.7632632689849,-1.60158163077267,0.76811479771682));
#5898=CARTESIAN_POINT('Ctrl Pts',(92.7675476423367,-1.62920639496417,0.710514924605348));
#5899=CARTESIAN_POINT('Ctrl Pts',(92.7718320156885,-1.65373901932468,0.651383101978016));
#5900=CARTESIAN_POINT('Ctrl Pts',(92.7761163890403,-1.67501720372595,0.591084959817191));
#5901=CARTESIAN_POINT('Ctrl Pts',(92.7803996859506,-1.69629004201977,0.53080196746149));
#5902=CARTESIAN_POINT('Ctrl Pts',(92.7846829828608,-1.71430989594296,0.469353712276196));
#5903=CARTESIAN_POINT('Ctrl Pts',(92.7889662797711,-1.72896331348721,0.407123965292314));
#5904=CARTESIAN_POINT('Ctrl Pts',(92.7932500423064,-1.74361832396242,0.344887453491231));
#5905=CARTESIAN_POINT('Ctrl Pts',(92.7975338048416,-1.75490605944284,0.28186977244651));
#5906=CARTESIAN_POINT('Ctrl Pts',(92.8018175673768,-1.76276392813596,0.21846600688138));
#5907=CARTESIAN_POINT('Ctrl Pts',(92.8061060878377,-1.7706305244734,0.154991819483508));
#5908=CARTESIAN_POINT('Ctrl Pts',(92.8103946082987,-1.77505959383456,0.0911311931016721));
#5909=CARTESIAN_POINT('Ctrl Pts',(92.8146831287597,-1.7760404364522,0.0272842552893976));
#5910=CARTESIAN_POINT('Ctrl Pts',(92.8189745295803,-1.77702193784703,-0.0366055649449436));
#5911=CARTESIAN_POINT('Ctrl Pts',(92.8232659304009,-1.77455062526379,-0.100481175186551));
#5912=CARTESIAN_POINT('Ctrl Pts',(92.8275573312215,-1.76866784348525,-0.163945484601535));
#5913=CARTESIAN_POINT('Ctrl Pts',(92.8318559678007,-1.76277514271052,-0.227516801596808));
#5914=CARTESIAN_POINT('Ctrl Pts',(92.8361546043798,-1.75345957497829,-0.290674937515888));
#5915=CARTESIAN_POINT('Ctrl Pts',(92.840453240959,-1.74081371049053,-0.353032134328007));
#5916=CARTESIAN_POINT('Ctrl Pts',(92.8414270904649,-1.73794880933956,-0.367159061363439));
#5917=CARTESIAN_POINT('Ctrl Pts',(92.8424009399708,-1.7349131854478,-0.381244943827301));
#5918=CARTESIAN_POINT('Ctrl Pts',(92.8433747894767,-1.73170826646264,-0.395285393563877));
#5919=CARTESIAN_POINT('Ctrl Pts',(92.8476735990735,-1.71756097121167,-0.45726336829579));
#5920=CARTESIAN_POINT('Ctrl Pts',(92.8519724086702,-1.70005337510742,-0.518607066947605));
#5921=CARTESIAN_POINT('Ctrl Pts',(92.8562712182669,-1.67925864640917,-0.578925263708581));
#5922=CARTESIAN_POINT('Ctrl Pts',(92.8606984802348,-1.6578425521565,-0.641045823477781));
#5923=CARTESIAN_POINT('Ctrl Pts',(92.8651257422027,-1.63293975690463,-0.702078069452736));
#5924=CARTESIAN_POINT('Ctrl Pts',(92.8695530041706,-1.60468696627331,-0.761606067972524));
#5925=CARTESIAN_POINT('Ctrl Pts',(92.8738399978295,-1.57732930477416,-0.819248049413498));
#5926=CARTESIAN_POINT('Ctrl Pts',(92.8781269914885,-1.54683099355722,-0.875479186541712));
#5927=CARTESIAN_POINT('Ctrl Pts',(92.8824139851475,-1.51336584339643,-0.929939721993324));
#5928=CARTESIAN_POINT('Ctrl Pts',(92.8866983585256,-1.47992114768489,-0.984366970271449));
#5929=CARTESIAN_POINT('Ctrl Pts',(92.8909827319036,-1.44351347241234,-1.0370253345937));
#5930=CARTESIAN_POINT('Ctrl Pts',(92.8952671052817,-1.40436218992483,-1.08758029681009));
#5931=CARTESIAN_POINT('Ctrl Pts',(92.8995504022186,-1.36522074412762,-1.13812255718188));
#5932=CARTESIAN_POINT('Ctrl Pts',(92.9038336991554,-1.3233373679364,-1.18656206631749));
#5933=CARTESIAN_POINT('Ctrl Pts',(92.9081169960923,-1.27897314805749,-1.23259553343663));
#5934=CARTESIAN_POINT('Ctrl Pts',(92.9124007586543,-1.23460410546924,-1.27863400472426));
#5935=CARTESIAN_POINT('Ctrl Pts',(92.9166845212163,-1.18775403591931,-1.32226555437649));
#5936=CARTESIAN_POINT('Ctrl Pts',(92.9209682837783,-1.1387210923156,-1.36322350933938));
#5937=CARTESIAN_POINT('Ctrl Pts',(92.9252568042662,-1.08963368838422,-1.40422695583273));
#5938=CARTESIAN_POINT('Ctrl Pts',(92.9295453247541,-1.03835896202669,-1.44255056134764));
#5939=CARTESIAN_POINT('Ctrl Pts',(92.933833845242,-0.985227420784922,-1.47796853546802));
#5940=CARTESIAN_POINT('Ctrl Pts',(92.9381252460897,-0.932060194053257,-1.51341029786423));
#5941=CARTESIAN_POINT('Ctrl Pts',(92.9424166469374,-0.877034105232559,-1.54594229080387));
#5942=CARTESIAN_POINT('Ctrl Pts',(92.9467080477851,-0.82050530832499,-1.57538411237086));
#5943=CARTESIAN_POINT('Ctrl Pts',(92.9510066843912,-0.763881197850672,-1.60487557598187));
#5944=CARTESIAN_POINT('Ctrl Pts',(92.9553053209974,-0.705749784086856,-1.6312662697093));
#5945=CARTESIAN_POINT('Ctrl Pts',(92.9596039576036,-0.646487131852348,-1.65442390300954));
#5946=CARTESIAN_POINT('Ctrl Pts',(92.960577806901,-0.63306127209009,-1.65967022806237));
#5947=CARTESIAN_POINT('Ctrl Pts',(92.9615516561985,-0.619577408992279,-1.66475082291976));
#5948=CARTESIAN_POINT('Ctrl Pts',(92.9625255054959,-0.60604000430414,-1.669664509919));
#5949=CARTESIAN_POINT('Ctrl Pts',(92.9668243150826,-0.546282580639698,-1.69135472916942));
#5950=CARTESIAN_POINT('Ctrl Pts',(92.9711231246693,-0.485237582363842,-1.70987697123046));
#5951=CARTESIAN_POINT('Ctrl Pts',(92.9754219342561,-0.423273476567525,-1.72508075942387));
#5952=CARTESIAN_POINT('Ctrl Pts',(92.9798491962252,-0.359457826325535,-1.74073885078556));
#5953=CARTESIAN_POINT('Ctrl Pts',(92.9842764581943,-0.294667731340171,-1.75287671939473));
#5954=CARTESIAN_POINT('Ctrl Pts',(92.9887037201634,-0.229326851357022,-1.76138390413523));
#5955=CARTESIAN_POINT('Ctrl Pts',(92.9929907138121,-0.166056157315864,-1.76962155693402));
#5956=CARTESIAN_POINT('Ctrl Pts',(92.9972777074609,-0.102269601256815,-1.77445508743876));
#5957=CARTESIAN_POINT('Ctrl Pts',(93.0015647011096,-0.0383637314043607,
-1.77583565867248));
#5958=CARTESIAN_POINT('Ctrl Pts',(93.0058490744773,0.0255030781299301,-1.77721538607837));
#5959=CARTESIAN_POINT('Ctrl Pts',(93.010133447845,0.0894885540990822,-1.77514632869863));
#5960=CARTESIAN_POINT('Ctrl Pts',(93.0144178212127,0.153192675496442,-1.76963161891797));
#5961=CARTESIAN_POINT('Ctrl Pts',(93.0187011181392,0.216880791345497,-1.76411829469843));
#5962=CARTESIAN_POINT('Ctrl Pts',(93.0229844150656,0.280287191138943,-1.75516108009091));
#5963=CARTESIAN_POINT('Ctrl Pts',(93.0272677119921,0.343015498596663,-1.74281508778828));
#5964=CARTESIAN_POINT('Ctrl Pts',(93.0315514745436,0.405750625071331,-1.73046775338774));
#5965=CARTESIAN_POINT('Ctrl Pts',(93.0358352370952,0.467807019197287,-1.71473101065585));
#5966=CARTESIAN_POINT('Ctrl Pts',(93.0401189996467,0.528798998452338,-1.69571096644912));
#5967=CARTESIAN_POINT('Ctrl Pts',(93.0444075201242,0.589858720799145,-1.67666979689746));
#5968=CARTESIAN_POINT('Ctrl Pts',(93.0486960406017,0.649851188524717,-1.65433820267206));
#5969=CARTESIAN_POINT('Ctrl Pts',(93.0529845610792,0.708407550322267,-1.62887163556445));
#5970=CARTESIAN_POINT('Ctrl Pts',(93.0572759619164,0.767003241158813,-1.60338796398552));
#5971=CARTESIAN_POINT('Ctrl Pts',(93.0615673627537,0.824160457267757,-1.57476535677365));
#5972=CARTESIAN_POINT('Ctrl Pts',(93.065858763591,0.879534600335056,-1.54320541384271));
#5973=CARTESIAN_POINT('Ctrl Pts',(93.0701574001868,0.935002110101268,-1.51159225748893));
#5974=CARTESIAN_POINT('Ctrl Pts',(93.0744560367826,0.988680128613843,-1.47703216068398));
#5975=CARTESIAN_POINT('Ctrl Pts',(93.0787546733784,1.04025370679951,-1.43976952599709));
#5976=CARTESIAN_POINT('Ctrl Pts',(93.0797285227573,1.05193762005059,-1.43132773455068));
#5977=CARTESIAN_POINT('Ctrl Pts',(93.0807023721362,1.06351366541221,-1.42274739559128));
#5978=CARTESIAN_POINT('Ctrl Pts',(93.0816762215151,1.07497843559964,-1.41403162110886));
#5979=CARTESIAN_POINT('Ctrl Pts',(93.086120407884,1.12729820546713,-1.37425696294458));
#5980=CARTESIAN_POINT('Ctrl Pts',(93.0905645942528,1.17751761796227,-1.33149086968185));
#5981=CARTESIAN_POINT('Ctrl Pts',(93.0950087806217,1.22527686049464,-1.2859862665038));
#5982=CARTESIAN_POINT('Ctrl Pts',(93.099299967917,1.27139190558409,-1.24204824077171));
#5983=CARTESIAN_POINT('Ctrl Pts',(93.1035911552123,1.31521299779926,-1.19555756077289));
#5984=CARTESIAN_POINT('Ctrl Pts',(93.1078823425076,1.35644716415272,-1.14678470227068));
#5985=CARTESIAN_POINT('Ctrl Pts',(93.112169235915,1.39764007039022,-1.09806064732084));
#5986=CARTESIAN_POINT('Ctrl Pts',(93.1164561293224,1.43625085980126,-1.04705932475888));
#5987=CARTESIAN_POINT('Ctrl Pts',(93.1207430227299,1.47202372930437,-0.994087623333509));
#5988=CARTESIAN_POINT('Ctrl Pts',(93.1250271698193,1.50777368158822,-0.941149857237133));
#5989=CARTESIAN_POINT('Ctrl Pts',(93.1293113169087,1.54068903955213,-0.886244633256476));
#5990=CARTESIAN_POINT('Ctrl Pts',(93.1335954639981,1.57055582273612,-0.82970987108125));
#5991=CARTESIAN_POINT('Ctrl Pts',(93.1378784086902,1.60041422344894,-0.773190976065579));
#5992=CARTESIAN_POINT('Ctrl Pts',(93.1421613533823,1.62722551427406,-0.715043896799184));
#5993=CARTESIAN_POINT('Ctrl Pts',(93.1464442980744,1.65082139094303,-0.655631602124937));
#5994=CARTESIAN_POINT('Ctrl Pts',(93.1507295910831,1.67443020511009,-0.596186731994426));
#5995=CARTESIAN_POINT('Ctrl Pts',(93.1550148840919,1.69481989690216,-0.535475729423321));
#5996=CARTESIAN_POINT('Ctrl Pts',(93.1593001771006,1.71187065899416,-0.473880691076261));
#5997=CARTESIAN_POINT('Ctrl Pts',(93.1635869163134,1.72892717539119,-0.412264865585633));
#5998=CARTESIAN_POINT('Ctrl Pts',(93.1678736555263,1.74264240457422,-0.349764901372216));
#5999=CARTESIAN_POINT('Ctrl Pts',(93.1721603947392,1.75294734932356,-0.286774568257931));
#6000=CARTESIAN_POINT('Ctrl Pts',(93.1764524215333,1.76326500495393,-0.223706538207797));
#6001=CARTESIAN_POINT('Ctrl Pts',(93.1807444483274,1.7701639253717,-0.160147432770856));
#6002=CARTESIAN_POINT('Ctrl Pts',(93.1850364751214,1.77362694173368,-0.0964962903765215));
#6003=CARTESIAN_POINT('Ctrl Pts',(93.1861365482037,1.77451453430148,-0.0801821078789996));
#6004=CARTESIAN_POINT('Ctrl Pts',(93.187236621286,1.77517667934864,-0.0638618768134948));
#6005=CARTESIAN_POINT('Ctrl Pts',(93.1883366943682,1.77561363837197,-0.0475422940912359));
#6006=CARTESIAN_POINT('Ctrl Pts',(92.4383302476831,1.77320199105525,-0.0474633882366439));
#6007=CARTESIAN_POINT('Ctrl Pts',(92.4541943789285,1.7807787260589,0.189242861096052));
#6008=CARTESIAN_POINT('Ctrl Pts',(92.5097754155136,1.6490061063227,1.02148169742008));
#6009=CARTESIAN_POINT('Ctrl Pts',(92.5733609426715,0.828714911293434,1.71278513326118));
#6010=CARTESIAN_POINT('Ctrl Pts',(92.621082338584,0.12056136551938,1.77794021860673));
#6011=CARTESIAN_POINT('Ctrl Pts',(92.6290868291567,0.00157956711881646,
1.77684271104738));
#6012=CARTESIAN_POINT('',(92.4812153597462,-0.0010931502662158,1.77831379137429));
#6013=CARTESIAN_POINT('Ctrl Pts',(92.2906253551795,1.77468168403539,-0.047528689603001));
#6014=CARTESIAN_POINT('Ctrl Pts',(92.3188942604556,1.7820374034528,0.373543767752086));
#6015=CARTESIAN_POINT('Ctrl Pts',(92.3824242619779,1.46982358280908,1.33346230864534));
#6016=CARTESIAN_POINT('Ctrl Pts',(92.4459542635001,0.521916176252472,1.77448723514747));
#6017=CARTESIAN_POINT('Ctrl Pts',(92.4812153597462,-0.0010931502662158,
1.77831379137429));
#6018=CARTESIAN_POINT('Ctrl Pts',(92.4824006868533,-0.00102231093804463,
1.77624970580725));
#6019=CARTESIAN_POINT('Ctrl Pts',(92.4845492905966,-0.0308338137244965,
1.77623254795761));
#6020=CARTESIAN_POINT('Ctrl Pts',(92.4866800846044,-0.0606420849328428,
1.77546488257387));
#6021=CARTESIAN_POINT('Ctrl Pts',(92.4900600408051,-0.108506512965212,1.77302521661446));
#6022=CARTESIAN_POINT('Ctrl Pts',(92.4913267374793,-0.126580022702816,1.77182663925871));
#6023=CARTESIAN_POINT('Ctrl Pts',(92.4931678342244,-0.153091812170338,1.76966069952318));
#6024=CARTESIAN_POINT('Ctrl Pts',(92.4937523798425,-0.161545936555108,1.76890898912668));
#6025=CARTESIAN_POINT('Ctrl Pts',(92.4947947242983,-0.176692663677203,1.7674526993751));
#6026=CARTESIAN_POINT('Ctrl Pts',(92.4952536823725,-0.183387201378406,1.76677063594963));
#6027=CARTESIAN_POINT('Ctrl Pts',(92.4961905783265,-0.197108315274421,1.76529384939534));
#6028=CARTESIAN_POINT('Ctrl Pts',(92.4966682223702,-0.204134026809555,1.76449521531135));
#6029=CARTESIAN_POINT('Ctrl Pts',(92.4977559852287,-0.220201914634042,1.76257147254318));
#6030=CARTESIAN_POINT('Ctrl Pts',(92.498364570249,-0.22924042489869,1.76141872240714));
#6031=CARTESIAN_POINT('Ctrl Pts',(92.5003155409023,-0.258356638486375,1.75747739097445));
#6032=CARTESIAN_POINT('Ctrl Pts',(92.501643747523,-0.278396401949765,1.75441456363633));
#6033=CARTESIAN_POINT('Ctrl Pts',(92.5074966346105,-0.367419455457645,1.73924460847041));
#6034=CARTESIAN_POINT('Ctrl Pts',(92.5118603367432,-0.43570968617708,1.7234059090987));
#6035=CARTESIAN_POINT('Ctrl Pts',(92.5199185636984,-0.561001786575576,1.68641988981419));
#6036=CARTESIAN_POINT('Ctrl Pts',(92.5236185218169,-0.618195851469421,1.66630400098528));
#6037=CARTESIAN_POINT('Ctrl Pts',(92.5326437004274,-0.753702442599686,1.61070544810568));
#6038=CARTESIAN_POINT('Ctrl Pts',(92.5379946540685,-0.830677246488275,1.57239063412253));
#6039=CARTESIAN_POINT('Ctrl Pts',(92.5452072081148,-0.926880391095909,1.51546315863747));
#6040=CARTESIAN_POINT('Ctrl Pts',(92.5468952372244,-0.948893826025128,1.50177769315874));
#6041=CARTESIAN_POINT('Ctrl Pts',(92.5495528525222,-0.982715258622012,1.47971080876184));
#6042=CARTESIAN_POINT('Ctrl Pts',(92.5505102582548,-0.994734096935685,1.47165804882015));
#6043=CARTESIAN_POINT('Ctrl Pts',(92.5523063093579,-1.016964628259,1.45636659146167));
#6044=CARTESIAN_POINT('Ctrl Pts',(92.5531435077076,-1.02720082871013,1.44916498284711));
#6045=CARTESIAN_POINT('Ctrl Pts',(92.5550273302939,-1.04994676311298,1.43280015880263));
#6046=CARTESIAN_POINT('Ctrl Pts',(92.5560761079423,-1.06241419502789,1.42358018811742));
#6047=CARTESIAN_POINT('Ctrl Pts',(92.5592547582628,-1.09960295474346,1.39531756746504));
#6048=CARTESIAN_POINT('Ctrl Pts',(92.561403622792,-1.12394361263514,1.37578643464634));
#6049=CARTESIAN_POINT('Ctrl Pts',(92.5731731089358,-1.2529044534201,1.26660024294768));
#6050=CARTESIAN_POINT('Ctrl Pts',(92.5832574740353,-1.34732281392176,1.16565625548978));
#6051=CARTESIAN_POINT('Ctrl Pts',(92.5987045445723,-1.47292661875574,0.995486829843145));
#6052=CARTESIAN_POINT('Ctrl Pts',(92.6040593281352,-1.51300256809924,0.933451742933734));
#6053=CARTESIAN_POINT('Ctrl Pts',(92.6104859292972,-1.55785274147325,0.853509464273474));
#6054=CARTESIAN_POINT('Ctrl Pts',(92.611727985458,-1.56636327041993,0.837788598602819));
#6055=CARTESIAN_POINT('Ctrl Pts',(92.6135588517891,-1.57869123875451,0.814171269895876));
#6056=CARTESIAN_POINT('Ctrl Pts',(92.614157916902,-1.58268959711021,0.80637121193379));
#6057=CARTESIAN_POINT('Ctrl Pts',(92.6151852269149,-1.58948753229712,0.792864328854585));
#6058=CARTESIAN_POINT('Ctrl Pts',(92.6156151172737,-1.59231439035989,0.78717173802353));
#6059=CARTESIAN_POINT('Ctrl Pts',(92.616621787836,-1.59889179991191,0.773746040087949));
#6060=CARTESIAN_POINT('Ctrl Pts',(92.6171970030907,-1.60261685703751,0.766000743864701));
#6061=CARTESIAN_POINT('Ctrl Pts',(92.6188658934207,-1.6133209839759,0.743324353929958));
#6062=CARTESIAN_POINT('Ctrl Pts',(92.61995088611,-1.62014885393761,0.728322340211201));
#6063=CARTESIAN_POINT('Ctrl Pts',(92.6285941527618,-1.67336603703679,0.606941641606831));
#6064=CARTESIAN_POINT('Ctrl Pts',(92.6356535983921,-1.70944311890215,0.496330273727835));
#6065=CARTESIAN_POINT('Ctrl Pts',(92.6487598942345,-1.75546517037981,0.287899998950804));
#6066=CARTESIAN_POINT('Ctrl Pts',(92.6547643035926,-1.76860351289484,0.191267654549485));
#6067=CARTESIAN_POINT('Ctrl Pts',(92.6630064392568,-1.77540991748136,0.0629020919228067));
#6068=CARTESIAN_POINT('Ctrl Pts',(92.6650282268388,-1.77624066832517,0.0317166686974413));
#6069=CARTESIAN_POINT('Ctrl Pts',(92.6680928712898,-1.77625452159584,-0.0149769166232618));
#6070=CARTESIAN_POINT('Ctrl Pts',(92.6691165253765,-1.77605613384216,-0.0304797886551062));
#6071=CARTESIAN_POINT('Ctrl Pts',(92.6709780469295,-1.77533088136162,-0.0584889915098783));
#6072=CARTESIAN_POINT('Ctrl Pts',(92.6718136462712,-1.7748747052451,-0.0709962487183724));
#6073=CARTESIAN_POINT('Ctrl Pts',(92.6736242825017,-1.77360626927814,-0.0979500158814898));
#6074=CARTESIAN_POINT('Ctrl Pts',(92.6746006555988,-1.77274958764284,-0.112393424764536));
#6075=CARTESIAN_POINT('Ctrl Pts',(92.6772946626731,-1.76991545896634,-0.151985751520627));
#6076=CARTESIAN_POINT('Ctrl Pts',(92.6790233757145,-1.76757863036,-0.177104692319194));
#6077=CARTESIAN_POINT('Ctrl Pts',(92.6902838227045,-1.74905353911342,-0.338811670470226));
#6078=CARTESIAN_POINT('Ctrl Pts',(92.700300299322,-1.71758321673294,-0.473155277589021));
#6079=CARTESIAN_POINT('Ctrl Pts',(92.7148508139103,-1.65008157532417,-0.660362602074984));
#6080=CARTESIAN_POINT('Ctrl Pts',(92.7193374353437,-1.62622339631619,-0.717109664540585));
#6081=CARTESIAN_POINT('Ctrl Pts',(92.7261522728757,-1.58473239674092,-0.80301633596489));
#6082=CARTESIAN_POINT('Ctrl Pts',(92.7285429440067,-1.56912602398888,-0.833100161945485));
#6083=CARTESIAN_POINT('Ctrl Pts',(92.7316607551414,-1.5472464559242,-0.872477528823854));
#6084=CARTESIAN_POINT('Ctrl Pts',(92.7324282416505,-1.54173349499317,-0.882182793020596));
#6085=CARTESIAN_POINT('Ctrl Pts',(92.7336927839779,-1.53243206937843,-0.89820389528087));
#6086=CARTESIAN_POINT('Ctrl Pts',(92.7341929820825,-1.52869522052787,-0.904549177455522));
#6087=CARTESIAN_POINT('Ctrl Pts',(92.7352062710777,-1.52100521738175,-0.917423259425176));
#6088=CARTESIAN_POINT('Ctrl Pts',(92.7357191748343,-1.51704926073363,-0.923950136253548));
#6089=CARTESIAN_POINT('Ctrl Pts',(92.7370598254484,-1.50654568553652,-0.941030498096524));
#6090=CARTESIAN_POINT('Ctrl Pts',(92.7378832328774,-1.49992910649765,-0.951541380102056));
#6091=CARTESIAN_POINT('Ctrl Pts',(92.7415219872807,-1.469979318751,-0.998029863197726));
#6092=CARTESIAN_POINT('Ctrl Pts',(92.7442688029124,-1.44545620347339,-1.03322786521234));
#6093=CARTESIAN_POINT('Ctrl Pts',(92.7555152196971,-1.33824239732307,-1.17581190044576));
#6094=CARTESIAN_POINT('Ctrl Pts',(92.7636216677633,-1.24467545659362,-1.27444640557481));
#6095=CARTESIAN_POINT('Ctrl Pts',(92.7760144671006,-1.09258281290789,-1.40188574127089));
#6096=CARTESIAN_POINT('Ctrl Pts',(92.7800049738278,-1.0422607701702,-1.43969165025828));
#6097=CARTESIAN_POINT('Ctrl Pts',(92.7853902078503,-0.973565239913303,-1.48580910498352));
#6098=CARTESIAN_POINT('Ctrl Pts',(92.7866916361762,-0.956903272501679,-1.4965941493721));
#6099=CARTESIAN_POINT('Ctrl Pts',(92.788876208919,-0.928860779391038,-1.51408588928242));
#6100=CARTESIAN_POINT('Ctrl Pts',(92.7897535146276,-0.917579621045383,-1.52094906247328));
#6101=CARTESIAN_POINT('Ctrl Pts',(92.7914886556546,-0.895236858220022,-1.53420279096481));
#6102=CARTESIAN_POINT('Ctrl Pts',(92.7923461417386,-0.884180746007873,-1.54060106118081));
#6103=CARTESIAN_POINT('Ctrl Pts',(92.7942475062959,-0.859639328325736,-1.55445220728275));
#6104=CARTESIAN_POINT('Ctrl Pts',(92.7952932825241,-0.846124247725795,-1.56184991941853));
#6105=CARTESIAN_POINT('Ctrl Pts',(92.798955337192,-0.798751502935135,-1.58698487436863));
#6106=CARTESIAN_POINT('Ctrl Pts',(92.8016031939177,-0.764421013818563,-1.60380331742119));
#6107=CARTESIAN_POINT('Ctrl Pts',(92.8133738097908,-0.611553288329752,-1.67266947766562));
#6108=CARTESIAN_POINT('Ctrl Pts',(92.8228685654091,-0.488084820807003,-1.71277101390206));
#6109=CARTESIAN_POINT('Ctrl Pts',(92.8375011641981,-0.291813139110086,-1.75355573015371));
#6110=CARTESIAN_POINT('Ctrl Pts',(92.8426510358254,-0.221434373987975,-1.76382577436859));
#6111=CARTESIAN_POINT('Ctrl Pts',(92.8488633136582,-0.133105667517972,-1.77134300593023));
#6112=CARTESIAN_POINT('Ctrl Pts',(92.8500845265591,-0.115565717665967,-1.77257377467411));
#6113=CARTESIAN_POINT('Ctrl Pts',(92.8518909360196,-0.0893148708898787,
-1.77402444886132));
#6114=CARTESIAN_POINT('Ctrl Pts',(92.8524860078789,-0.0806165145990328,
-1.77444100407357));
#6115=CARTESIAN_POINT('Ctrl Pts',(92.8535091260019,-0.0655671513773256,
-1.77505080921174));
#6116=CARTESIAN_POINT('Ctrl Pts',(92.8539387730379,-0.0592178169983456,
-1.77527397327142));
#6117=CARTESIAN_POINT('Ctrl Pts',(92.8549487071626,-0.0442234059140566,
-1.77572045444784));
#6118=CARTESIAN_POINT('Ctrl Pts',(92.855527385033,-0.0355777341403585,-1.77591471490798));
#6119=CARTESIAN_POINT('Ctrl Pts',(92.8572520826953,-0.00966083257458799,
-1.77630770135782));
#6120=CARTESIAN_POINT('Ctrl Pts',(92.8583883024626,0.00761279225494029,
-1.77631767472473));
#6121=CARTESIAN_POINT('Ctrl Pts',(92.86653258003,0.132619545578985,-1.77456620537457));
#6122=CARTESIAN_POINT('Ctrl Pts',(92.8731165972371,0.240008591932103,-1.76325698748452));
#6123=CARTESIAN_POINT('Ctrl Pts',(92.8821534255,0.384422170338835,-1.73460092324287));
#6124=CARTESIAN_POINT('Ctrl Pts',(92.8845754883257,0.422855596923087,-1.72563432677218));
#6125=CARTESIAN_POINT('Ctrl Pts',(92.8904142863441,0.514030905315646,-1.70113386405873));
#6126=CARTESIAN_POINT('Ctrl Pts',(92.8938453141875,0.566410003937744,-1.68441777622951));
#6127=CARTESIAN_POINT('Ctrl Pts',(92.8997656804178,0.653591557548651,-1.6520681557862));
#6128=CARTESIAN_POINT('Ctrl Pts',(92.9022179913669,0.688819078532507,-1.6376932136476));
#6129=CARTESIAN_POINT('Ctrl Pts',(92.9058012086586,0.738810826708043,-1.61539519226944));
#6130=CARTESIAN_POINT('Ctrl Pts',(92.9069016064861,0.753968355934791,-1.60837643341001));
#6131=CARTESIAN_POINT('Ctrl Pts',(92.9088478377335,0.780420239781259,-1.59567168918139));
#6132=CARTESIAN_POINT('Ctrl Pts',(92.9096904685797,0.79175722852988,-1.59007684318077));
#6133=CARTESIAN_POINT('Ctrl Pts',(92.9114597920135,0.815315333711167,-1.57813642326924));
#6134=CARTESIAN_POINT('Ctrl Pts',(92.912387216655,0.827524271661795,-1.57176882048247));
#6135=CARTESIAN_POINT('Ctrl Pts',(92.9148481840782,0.859546591391078,-1.55459098129583));
#6136=CARTESIAN_POINT('Ctrl Pts',(92.9163900352327,0.879229531531933,-1.54354423676119));
#6137=CARTESIAN_POINT('Ctrl Pts',(92.9248754401273,0.985450544687864,-1.48123839899402));
#6138=CARTESIAN_POINT('Ctrl Pts',(92.9320681726743,1.06771204575358,-1.42308289105365));
#6139=CARTESIAN_POINT('Ctrl Pts',(92.9447646069896,1.20108617267584,-1.3106915638036));
#6140=CARTESIAN_POINT('Ctrl Pts',(92.9501936567461,1.25454713468574,-1.25961573684614));
#6141=CARTESIAN_POINT('Ctrl Pts',(92.9598962218267,1.34522951642781,-1.16146180282468));
#6142=CARTESIAN_POINT('Ctrl Pts',(92.9641854274155,1.38354927611218,-1.11553971861347));
#6143=CARTESIAN_POINT('Ctrl Pts',(92.9692602804409,1.42742427844582,-1.05721259236665));
#6144=CARTESIAN_POINT('Ctrl Pts',(92.9701720244142,1.43524690480812,-1.04656814613235));
#6145=CARTESIAN_POINT('Ctrl Pts',(92.9716101838399,1.44750095043408,-1.02949791328233));
#6146=CARTESIAN_POINT('Ctrl Pts',(92.9721415668433,1.45200984371182,-1.02312871851253));
#6147=CARTESIAN_POINT('Ctrl Pts',(92.9731559433584,1.46058343567568,-1.01084695361096));
#6148=CARTESIAN_POINT('Ctrl Pts',(92.9736393323113,1.4646544827768,-1.00493919428011));
#6149=CARTESIAN_POINT('Ctrl Pts',(92.9747147103402,1.47367541374086,-0.991677074690893));
#6150=CARTESIAN_POINT('Ctrl Pts',(92.9753054572041,1.47860633269386,-0.984309893588972));
#6151=CARTESIAN_POINT('Ctrl Pts',(92.9773833078538,1.49585248192924,-0.958120726478997));
#6152=CARTESIAN_POINT('Ctrl Pts',(92.9788521920085,1.50786571471827,-0.939101205229439));
#6153=CARTESIAN_POINT('Ctrl Pts',(92.9886090336211,1.58614626039876,-0.809789372513874));
#6154=CARTESIAN_POINT('Ctrl Pts',(92.996351921846,1.64062870818219,-0.692794488604774));
#6155=CARTESIAN_POINT('Ctrl Pts',(93.0094907831567,1.70913289062676,-0.490976106703148));
#6156=CARTESIAN_POINT('Ctrl Pts',(93.014756121613,1.73053336059814,-0.409200099982136));
#6157=CARTESIAN_POINT('Ctrl Pts',(93.0218643634416,1.75076118881186,-0.300933470738367));
#6158=CARTESIAN_POINT('Ctrl Pts',(93.0235399162205,1.75493522141452,-0.275550273559126));
#6159=CARTESIAN_POINT('Ctrl Pts',(93.0261822486872,1.76058766833873,-0.235803422187769));
#6160=CARTESIAN_POINT('Ctrl Pts',(93.0271370818637,1.7624447312373,-0.221496592505313));
#6161=CARTESIAN_POINT('Ctrl Pts',(93.0289308379924,1.76558742425185,-0.194735308690751));
#6162=CARTESIAN_POINT('Ctrl Pts',(93.0297683470956,1.7669160494045,-0.182286734644646));
#6163=CARTESIAN_POINT('Ctrl Pts',(93.0316562258704,1.76960065690939,-0.154336330564025));
#6164=CARTESIAN_POINT('Ctrl Pts',(93.0327087908997,1.77088472937446,-0.138828801814831));
#6165=CARTESIAN_POINT('Ctrl Pts',(93.0354350894068,1.77366549006005,-0.0988682382603739));
#6166=CARTESIAN_POINT('Ctrl Pts',(93.0371180501293,1.77486027676062,-0.0743982061153983));
#6167=CARTESIAN_POINT('Ctrl Pts',(93.0388710464405,1.77557080561487,-0.0491223100769542));
#6168=CARTESIAN_POINT('Ctrl Pts',(93.0389258516589,1.77559248579042,-0.0483323025080003));
#6169=CARTESIAN_POINT('Ctrl Pts',(93.0389806716277,1.77561363837854,-0.0475422938458683));
#6170=CARTESIAN_POINT('Origin',(88.3562164250559,0.,0.));
#6171=CARTESIAN_POINT('',(93.938045236354,1.77561363622783,-0.0475423741708462));
#6172=CARTESIAN_POINT('',(93.7915308013958,1.77561364010973,-0.0475422291890938));
#6173=CARTESIAN_POINT('',(88.3562164250559,1.77561363837197,-0.0475422940912398));
#6174=CARTESIAN_POINT('',(93.3790868291138,3.82645600525644E-5,1.77624999958785));
#6175=CARTESIAN_POINT('Ctrl Pts',(93.938045236354,1.77561363622783,-0.0475423741708462));
#6176=CARTESIAN_POINT('Ctrl Pts',(93.9320040216653,1.77340196817429,-0.130143801279928));
#6177=CARTESIAN_POINT('Ctrl Pts',(93.9259827141224,1.76542829118073,-0.212520978178856));
#6178=CARTESIAN_POINT('Ctrl Pts',(93.9189430774626,1.74880132298718,-0.311564728677188));
#6179=CARTESIAN_POINT('Ctrl Pts',(93.9177108384249,1.74560292013426,-0.329012389570148));
#6180=CARTESIAN_POINT('Ctrl Pts',(93.9158914723543,1.74043938351934,-0.354980524151267));
#6181=CARTESIAN_POINT('Ctrl Pts',(93.9152942701028,1.73867194715723,-0.363538565386476));
#6182=CARTESIAN_POINT('Ctrl Pts',(93.9142211954599,1.73536307937548,-0.378983967867905));
#6183=CARTESIAN_POINT('Ctrl Pts',(93.9137441574733,1.73384369704369,-0.385875502480605));
#6184=CARTESIAN_POINT('Ctrl Pts',(93.9126651008141,1.73029650687055,-0.401520593850451));
#6185=CARTESIAN_POINT('Ctrl Pts',(93.9120645188153,1.72824331213126,-0.410268024280801));
#6186=CARTESIAN_POINT('Ctrl Pts',(93.9102023132568,1.72163309880907,-0.437499655893678));
#6187=CARTESIAN_POINT('Ctrl Pts',(93.9089529366966,1.71684507731633,-0.455927108119867));
#6188=CARTESIAN_POINT('Ctrl Pts',(93.9059971615295,1.70469268330158,-0.499787745425835));
#6189=CARTESIAN_POINT('Ctrl Pts',(93.9043032002053,1.69705400952092,-0.525140715300347));
#6190=CARTESIAN_POINT('Ctrl Pts',(93.8976356766913,1.66442135475245,-0.625286486790069));
#6191=CARTESIAN_POINT('Ctrl Pts',(93.8928080019055,1.63502490232017,-0.698553404615874));
#6192=CARTESIAN_POINT('Ctrl Pts',(93.8811612913827,1.55280905710831,-0.869565360747237));
#6193=CARTESIAN_POINT('Ctrl Pts',(93.8743435594647,1.49551655721073,-0.964772756437486));
#6194=CARTESIAN_POINT('Ctrl Pts',(93.8656231815207,1.41518924734116,-1.07373352421836));
#6195=CARTESIAN_POINT('Ctrl Pts',(93.8640310575246,1.40024560860681,-1.09314977429124));
#6196=CARTESIAN_POINT('Ctrl Pts',(93.8614022300274,1.37516165013015,-1.12438278616003));
#6197=CARTESIAN_POINT('Ctrl Pts',(93.860374909867,1.36525880250877,-1.13638663766106));
#6198=CARTESIAN_POINT('Ctrl Pts',(93.8585094737317,1.34710640653279,-1.15781049174282));
#6199=CARTESIAN_POINT('Ctrl Pts',(93.8576736701088,1.33891245749085,-1.16727641228749));
#6200=CARTESIAN_POINT('Ctrl Pts',(93.8558657023713,1.32106227848848,-1.18746227684354));
#6201=CARTESIAN_POINT('Ctrl Pts',(93.854892236438,1.31137418965857,-1.19815270973303));
#6202=CARTESIAN_POINT('Ctrl Pts',(93.852167665216,1.28405328395881,-1.22757194110003));
#6203=CARTESIAN_POINT('Ctrl Pts',(93.8504047869165,1.26614286407437,-1.24603685078672));
#6204=CARTESIAN_POINT('Ctrl Pts',(93.8427821983548,1.18774993255499,-1.32342099599285));
#6205=CARTESIAN_POINT('Ctrl Pts',(93.8367592011628,1.1235169424988,-1.37836828469259));
#6206=CARTESIAN_POINT('Ctrl Pts',(93.8212964989863,0.952147037806917,-1.50500371886784));
#6207=CARTESIAN_POINT('Ctrl Pts',(93.8117473829804,0.840662388396832,-1.57000265675587));
#6208=CARTESIAN_POINT('Ctrl Pts',(93.8010731118007,0.702582103987041,-1.63154793593117));
#6209=CARTESIAN_POINT('Ctrl Pts',(93.7995005288713,0.681858372751672,-1.64031690684089));
#6210=CARTESIAN_POINT('Ctrl Pts',(93.7973372793348,0.65274327787238,-1.65198937038501));
#6211=CARTESIAN_POINT('Ctrl Pts',(93.796729103392,0.644489271345008,-1.65522694941303));
#6212=CARTESIAN_POINT('Ctrl Pts',(93.7956352028668,0.629512374601053,-1.66097251948509));
#6213=CARTESIAN_POINT('Ctrl Pts',(93.7951482643689,0.622797877921894,-1.66350183377455));
#6214=CARTESIAN_POINT('Ctrl Pts',(93.7941369295977,0.608749083073824,-1.668696948887));
#6215=CARTESIAN_POINT('Ctrl Pts',(93.7936129674733,0.60141227312868,-1.67135520969737));
#6216=CARTESIAN_POINT('Ctrl Pts',(93.7922095065985,0.581611016536679,-1.67838229469115));
#6217=CARTESIAN_POINT('Ctrl Pts',(93.7913351096576,0.569114687547398,-1.68266069063211));
#6218=CARTESIAN_POINT('Ctrl Pts',(93.7865443292087,0.499845642432611,-1.70551649918976));
#6219=CARTESIAN_POINT('Ctrl Pts',(93.7827644038038,0.442205434573861,-1.72136228336056));
#6220=CARTESIAN_POINT('Ctrl Pts',(93.7744414191052,0.311726065367402,-1.75024304915061));
#6221=CARTESIAN_POINT('Ctrl Pts',(93.7699362214605,0.238653546971698,-1.76169492882366));
#6222=CARTESIAN_POINT('Ctrl Pts',(93.7592068748755,0.0649472156665822,-1.77790874772957));
#6223=CARTESIAN_POINT('Ctrl Pts',(93.7529613073609,-0.0357842304775489,
-1.77873368640014));
#6224=CARTESIAN_POINT('Ctrl Pts',(93.7449809601596,-0.158548078522177,-1.76930390121176));
#6225=CARTESIAN_POINT('Ctrl Pts',(93.74350540095,-0.181022977274753,-1.76714583281572));
#6226=CARTESIAN_POINT('Ctrl Pts',(93.7411082494639,-0.217130638805094,-1.76298270003029));
#6227=CARTESIAN_POINT('Ctrl Pts',(93.7401951249918,-0.230792296317716,-1.76124632371576));
#6228=CARTESIAN_POINT('Ctrl Pts',(93.738434051685,-0.256954154033847,-1.7576115767237));
#6229=CARTESIAN_POINT('Ctrl Pts',(93.7375869460015,-0.269457024522909,-1.75573824630454));
#6230=CARTESIAN_POINT('Ctrl Pts',(93.7356108454345,-0.298427873986478,-1.75108074952302));
#6231=CARTESIAN_POINT('Ctrl Pts',(93.7344787718251,-0.31487846980857,-1.74819750121955));
#6232=CARTESIAN_POINT('Ctrl Pts',(93.7307449589138,-0.36864215321565,-1.73799103540254));
#6233=CARTESIAN_POINT('Ctrl Pts',(93.7281130893119,-0.405758784505321,-1.7297020849127));
#6234=CARTESIAN_POINT('Ctrl Pts',(93.721593863067,-0.495768168326045,-1.70654457585489));
#6235=CARTESIAN_POINT('Ctrl Pts',(93.7176713089756,-0.548289936558882,-1.69040162929042));
#6236=CARTESIAN_POINT('Ctrl Pts',(93.7109035364631,-0.636404528595163,-1.65878006568367));
#6237=CARTESIAN_POINT('Ctrl Pts',(93.708084219214,-0.672395254245937,-1.64452013650389));
#6238=CARTESIAN_POINT('Ctrl Pts',(93.6973167712531,-0.807563790766749,-1.58578542617183));
#6239=CARTESIAN_POINT('Ctrl Pts',(93.6893190562768,-0.903059490742636,-1.53341513067342));
#6240=CARTESIAN_POINT('Ctrl Pts',(93.6805019194833,-1.0074357216936,-1.463021946694));
#6241=CARTESIAN_POINT('Ctrl Pts',(93.6793076720034,-1.02155711672744,-1.45319684214763));
#6242=CARTESIAN_POINT('Ctrl Pts',(93.6775329577856,-1.04254900703042,-1.43813426825716));
#6243=CARTESIAN_POINT('Ctrl Pts',(93.6769430978779,-1.04952721898671,-1.43304962581714));
#6244=CARTESIAN_POINT('Ctrl Pts',(93.6759251672233,-1.06157630512161,-1.42413489037724));
#6245=CARTESIAN_POINT('Ctrl Pts',(93.67549555619,-1.06666396515449,-1.42032828112927));
#6246=CARTESIAN_POINT('Ctrl Pts',(93.6744806943274,-1.07868764781347,-1.41123106262069));
#6247=CARTESIAN_POINT('Ctrl Pts',(93.6738971130666,-1.08560525780212,-1.40591656434271));
#6248=CARTESIAN_POINT('Ctrl Pts',(93.6721422362356,-1.10640654405852,-1.38969076356396));
#6249=CARTESIAN_POINT('Ctrl Pts',(93.6709812543199,-1.12016740256564,-1.37862282997714));
#6250=CARTESIAN_POINT('Ctrl Pts',(93.6651607267225,-1.18899510136212,-1.32155321326461));
#6251=CARTESIAN_POINT('Ctrl Pts',(93.6606817891378,-1.2414092592409,-1.27244550061471));
#6252=CARTESIAN_POINT('Ctrl Pts',(93.6481322897824,-1.38107371344113,-1.12472171908964));
#6253=CARTESIAN_POINT('Ctrl Pts',(93.64018721298,-1.46053336418497,-1.01941360888621));
#6254=CARTESIAN_POINT('Ctrl Pts',(93.629452946566,-1.54646306402993,-0.874572502762036));
#6255=CARTESIAN_POINT('Ctrl Pts',(93.6270726174005,-1.5642923033565,-0.842267390571588));
#6256=CARTESIAN_POINT('Ctrl Pts',(93.6235871731112,-1.58854659193674,-0.794890356955141));
#6257=CARTESIAN_POINT('Ctrl Pts',(93.622510641265,-1.5957900482274,-0.780246785797454));
#6258=CARTESIAN_POINT('Ctrl Pts',(93.6205892437427,-1.60827389349649,-0.754107877552704));
#6259=CARTESIAN_POINT('Ctrl Pts',(93.6197472674936,-1.61359563377497,-0.742652492098289));
#6260=CARTESIAN_POINT('Ctrl Pts',(93.6179758703421,-1.6244786988911,-0.718556683492309));
#6261=CARTESIAN_POINT('Ctrl Pts',(93.6170456812708,-1.63001567041215,-0.705906258640449));
#6262=CARTESIAN_POINT('Ctrl Pts',(93.6145691188102,-1.64428507611031,-0.672241385998971));
#6263=CARTESIAN_POINT('Ctrl Pts',(93.613014246432,-1.65276188417493,-0.651122079812201));
#6264=CARTESIAN_POINT('Ctrl Pts',(93.6095527734262,-1.67057024239244,-0.604163563689118));
#6265=CARTESIAN_POINT('Ctrl Pts',(93.6076404817285,-1.6797126333686,-0.57825934860139));
#6266=CARTESIAN_POINT('Ctrl Pts',(93.6015572786598,-1.70662140550392,-0.495983965454961));
#6267=CARTESIAN_POINT('Ctrl Pts',(93.5973239914352,-1.72217608872023,-0.438936328486937));
#6268=CARTESIAN_POINT('Ctrl Pts',(93.5846665985152,-1.7596541039577,-0.268383065021125));
#6269=CARTESIAN_POINT('Ctrl Pts',(93.5761140902391,-1.77338156229753,-0.153394345805444));
#6270=CARTESIAN_POINT('Ctrl Pts',(93.5653547064575,-1.77658990258446,-0.00301404823629758));
#6271=CARTESIAN_POINT('Ctrl Pts',(93.5628899757895,-1.77630657168885,0.0318764618742547));
#6272=CARTESIAN_POINT('Ctrl Pts',(93.5596680361613,-1.774559399598,0.0783447079826956));
#6273=CARTESIAN_POINT('Ctrl Pts',(93.5588686561726,-1.77400917811231,0.0899467069330056));
#6274=CARTESIAN_POINT('Ctrl Pts',(93.5576162994511,-1.77296102903341,0.108251589740391));
#6275=CARTESIAN_POINT('Ctrl Pts',(93.5571593327062,-1.77253880812099,0.114958230110525));
#6276=CARTESIAN_POINT('Ctrl Pts',(93.5562075753711,-1.77157561560948,0.128987642825595));
#6277=CARTESIAN_POINT('Ctrl Pts',(93.5557132402909,-1.77102728244535,0.136309726393413));
#6278=CARTESIAN_POINT('Ctrl Pts',(93.5544808293402,-1.76953970340671,0.154646361069168));
#6279=CARTESIAN_POINT('Ctrl Pts',(93.5537458725701,-1.76854298921556,0.165656179447372));
#6280=CARTESIAN_POINT('Ctrl Pts',(93.5508397881039,-1.76416570170394,0.209450866852258));
#6281=CARTESIAN_POINT('Ctrl Pts',(93.5487088337633,-1.75997552144474,0.242150319740251));
#6282=CARTESIAN_POINT('Ctrl Pts',(93.5428621565831,-1.74578335828127,0.332809238409397));
#6283=CARTESIAN_POINT('Ctrl Pts',(93.5392166058674,-1.73380960088183,0.390418678743127));
#6284=CARTESIAN_POINT('Ctrl Pts',(93.5268157923828,-1.6830938510655,0.58530846024065));
#6285=CARTESIAN_POINT('Ctrl Pts',(93.5181791435398,-1.63071217137066,0.71844605225803));
#6286=CARTESIAN_POINT('Ctrl Pts',(93.5073803504127,-1.55130555524469,0.865516791338427));
#6287=CARTESIAN_POINT('Ctrl Pts',(93.5057779949659,-1.5391804827255,0.886899987323495));
#6288=CARTESIAN_POINT('Ctrl Pts',(93.5032165485324,-1.51929128506586,0.920338720983961));
#6289=CARTESIAN_POINT('Ctrl Pts',(93.502267971553,-1.51181792878284,0.932564153379881));
#6290=CARTESIAN_POINT('Ctrl Pts',(93.5004876003179,-1.49759709416095,0.955207322603171));
#6291=CARTESIAN_POINT('Ctrl Pts',(93.4996572158886,-1.49088670474775,0.96564740236655));
#6292=CARTESIAN_POINT('Ctrl Pts',(93.4977710677138,-1.47547387399292,0.989083166695137));
#6293=CARTESIAN_POINT('Ctrl Pts',(93.4967129711615,-1.46670818130958,1.0020358012658));
#6294=CARTESIAN_POINT('Ctrl Pts',(93.4934754822273,-1.43953490224797,1.04106783774419));
#6295=CARTESIAN_POINT('Ctrl Pts',(93.4912760415947,-1.42059521647486,1.06676706908511));
#6296=CARTESIAN_POINT('Ctrl Pts',(93.4834010547684,-1.35114595929353,1.15587139016386));
#6297=CARTESIAN_POINT('Ctrl Pts',(93.477590588653,-1.29700616966977,1.21630838152252));
#6298=CARTESIAN_POINT('Ctrl Pts',(93.4646098790515,-1.16909880101702,1.34080956590284));
#6299=CARTESIAN_POINT('Ctrl Pts',(93.4574212913631,-1.0937855026046,1.4029240500182));
#6300=CARTESIAN_POINT('Ctrl Pts',(93.447431567054,-0.979698571696433,1.48221965593684));
#6301=CARTESIAN_POINT('Ctrl Pts',(93.4444868008816,-0.944818467454322,1.50469367654985));
#6302=CARTESIAN_POINT('Ctrl Pts',(93.4407546436979,-0.898616901716072,1.53222156787718));
#6303=CARTESIAN_POINT('Ctrl Pts',(93.4399072166342,-0.887987771924987,1.53840599561718));
#6304=CARTESIAN_POINT('Ctrl Pts',(93.43854652272,-0.870681856791702,1.54823609610075));
#6305=CARTESIAN_POINT('Ctrl Pts',(93.4380291376247,-0.864044592340077,1.55195001626316));
#6306=CARTESIAN_POINT('Ctrl Pts',(93.4370148880427,-0.850916603994066,1.5591855311238));
#6307=CARTESIAN_POINT('Ctrl Pts',(93.4365178964449,-0.844427428477376,1.5627094768021));
#6308=CARTESIAN_POINT('Ctrl Pts',(93.4352692836025,-0.827987626292969,1.57150480404216));
#6309=CARTESIAN_POINT('Ctrl Pts',(93.4345209589256,-0.818008285627792,1.5767223342951));
#6310=CARTESIAN_POINT('Ctrl Pts',(93.4314840568817,-0.777025429479143,1.59765568726248));
#6311=CARTESIAN_POINT('Ctrl Pts',(93.4292403758418,-0.745611308637735,1.612555848503));
#6312=CARTESIAN_POINT('Ctrl Pts',(93.4229490148593,-0.655011100536116,1.6523144714842));
#6313=CARTESIAN_POINT('Ctrl Pts',(93.4189849535115,-0.594885739416275,1.67490141431019));
#6314=CARTESIAN_POINT('Ctrl Pts',(93.4069910764914,-0.408801994032356,1.73351753081802));
#6315=CARTESIAN_POINT('Ctrl Pts',(93.3990256278216,-0.279986124400423,1.75892182844338));
#6316=CARTESIAN_POINT('Ctrl Pts',(93.3888759361916,-0.122991419722221,1.77218727789034));
#6317=CARTESIAN_POINT('Ctrl Pts',(93.3871422672075,-0.0963835139330152,
1.77383334469483));
#6318=CARTESIAN_POINT('Ctrl Pts',(93.3844889443492,-0.0560514774909538,
1.77541832429632));
#6319=CARTESIAN_POINT('Ctrl Pts',(93.3835829948779,-0.0423477859082393,
1.77579802955084));
#6320=CARTESIAN_POINT('Ctrl Pts',(93.3820343143278,-0.0190449371209913,
1.77617382839407));
#6321=CARTESIAN_POINT('Ctrl Pts',(93.3813941425469,-0.00944758569584646,
1.77625080269604));
#6322=CARTESIAN_POINT('Ctrl Pts',(93.3807515265229,0.000149729197527163,
1.77624999368928));
#6323=CARTESIAN_POINT('Ctrl Pts',(93.1883366943682,1.77561363837197,-0.0475422940912359));
#6324=CARTESIAN_POINT('Ctrl Pts',(93.1925001087569,1.77726738439512,0.0142219528650102));
#6325=CARTESIAN_POINT('Ctrl Pts',(93.1966635231455,1.77569212163206,0.0759763082135405));
#6326=CARTESIAN_POINT('Ctrl Pts',(93.2008269375341,1.77093077259767,0.13736178932519));
#6327=CARTESIAN_POINT('Ctrl Pts',(93.205125747123,1.7660145833899,0.200743540500161));
#6328=CARTESIAN_POINT('Ctrl Pts',(93.2094245567119,1.75768143007869,0.263990072622322));
#6329=CARTESIAN_POINT('Ctrl Pts',(93.2137233663007,1.74594638510628,0.326703662107288));
#6330=CARTESIAN_POINT('Ctrl Pts',(93.2181506282696,1.73386068620864,0.391291191263542));
#6331=CARTESIAN_POINT('Ctrl Pts',(93.2225778902384,1.71816647917446,0.45531287608599));
#6332=CARTESIAN_POINT('Ctrl Pts',(93.2270051522073,1.69893806927726,0.518337244716658));
#6333=CARTESIAN_POINT('Ctrl Pts',(93.2312921458582,1.68031887038518,0.579364821144228));
#6334=CARTESIAN_POINT('Ctrl Pts',(93.235579139509,1.65838623789395,0.639456812182291));
#6335=CARTESIAN_POINT('Ctrl Pts',(93.2398661331599,1.63325941068488,0.698231881189398));
#6336=CARTESIAN_POINT('Ctrl Pts',(93.2441505065298,1.60814794140566,0.756971025908113));
#6337=CARTESIAN_POINT('Ctrl Pts',(93.2484348798996,1.57984634677411,0.814394382467918));
#6338=CARTESIAN_POINT('Ctrl Pts',(93.2527192532695,1.54852263283247,0.870138907362264));
#6339=CARTESIAN_POINT('Ctrl Pts',(93.2570025501981,1.51720678891874,0.925869426543002));
#6340=CARTESIAN_POINT('Ctrl Pts',(93.2612858471267,1.48287057976837,0.979921512287453));
#6341=CARTESIAN_POINT('Ctrl Pts',(93.2655691440553,1.44572785001253,1.03195690132784));
#6342=CARTESIAN_POINT('Ctrl Pts',(93.269852906609,1.40858108257572,1.08399794698801));
#6343=CARTESIAN_POINT('Ctrl Pts',(93.2741366691627,1.36862748439017,1.13402145265898));
#6344=CARTESIAN_POINT('Ctrl Pts',(93.2784204317164,1.32612293023111,1.18171994838679));
#6345=CARTESIAN_POINT('Ctrl Pts',(93.282708952196,1.28357116675154,1.22947142228638));
#6346=CARTESIAN_POINT('Ctrl Pts',(93.2869974726756,1.23846313195367,1.27489235892395));
#6347=CARTESIAN_POINT('Ctrl Pts',(93.2912859931552,1.19109269473216,1.31771099071674));
#6348=CARTESIAN_POINT('Ctrl Pts',(93.2955773939946,1.14369044143279,1.36055838139382));
#6349=CARTESIAN_POINT('Ctrl Pts',(93.299868794834,1.0940231544451,1.40079967367227));
#6350=CARTESIAN_POINT('Ctrl Pts',(93.3041601956733,1.04241672098266,1.43820424221171));
#6351=CARTESIAN_POINT('Ctrl Pts',(93.3084588322712,0.990723273581195,1.47567187883449));
#6352=CARTESIAN_POINT('Ctrl Pts',(93.3127574688691,0.93708458160194,1.51029298062953));
#6353=CARTESIAN_POINT('Ctrl Pts',(93.317056105467,0.88185327564548,1.5418815981564));
#6354=CARTESIAN_POINT('Ctrl Pts',(93.3180299548291,0.869340710126261,1.54903794978745));
#6355=CARTESIAN_POINT('Ctrl Pts',(93.3190038041912,0.856746490809696,1.55603885512491));
#6356=CARTESIAN_POINT('Ctrl Pts',(93.3199776535533,0.844074858812542,1.56288249565365));
#6357=CARTESIAN_POINT('Ctrl Pts',(93.3245053479899,0.785160944681927,1.59470046910347));
#6358=CARTESIAN_POINT('Ctrl Pts',(93.3290330424265,0.724353261935751,1.62323346819936));
#6359=CARTESIAN_POINT('Ctrl Pts',(93.333560736863,0.662032291516035,1.64826493850049));
#6360=CARTESIAN_POINT('Ctrl Pts',(93.3380747387602,0.599899790604014,1.67322070926015));
#6361=CARTESIAN_POINT('Ctrl Pts',(93.3425887406574,0.536263505898929,1.69469587559583));
#6362=CARTESIAN_POINT('Ctrl Pts',(93.3471027425546,0.471526535092008,1.71252059526422));
#6363=CARTESIAN_POINT('Ctrl Pts',(93.3516083627061,0.406909769999983,1.73031221741286));
#6364=CARTESIAN_POINT('Ctrl Pts',(93.3561139828576,0.341196788975856,1.74446675420195));
#6365=CARTESIAN_POINT('Ctrl Pts',(93.3606196030091,0.274808832373806,1.7548630055219));
#6366=CARTESIAN_POINT('Ctrl Pts',(93.3651149452393,0.208572315568176,1.76523554160397));
#6367=CARTESIAN_POINT('Ctrl Pts',(93.3696102874694,0.141664306510061,1.77186679104811));
#6368=CARTESIAN_POINT('Ctrl Pts',(93.3741056296996,0.074517532603036,1.77468622574098));
#6369=CARTESIAN_POINT('Ctrl Pts',(93.3757660295043,0.0497161972259653,1.77572761226371));
#6370=CARTESIAN_POINT('Ctrl Pts',(93.3774264293091,0.0248823982268752,1.77624946438737));
#6371=CARTESIAN_POINT('Ctrl Pts',(93.3790868291138,3.82645600525644E-5,
1.77624999958785));
#6372=CARTESIAN_POINT('Ctrl Pts',(93.0389806716277,1.77561363837854,-0.0475422938458682));
#6373=CARTESIAN_POINT('Ctrl Pts',(93.0466237494881,1.77856276223817,0.0626018351563203));
#6374=CARTESIAN_POINT('Ctrl Pts',(93.0545765376933,1.77125660689251,0.172765614818531));
#6375=CARTESIAN_POINT('Ctrl Pts',(93.068382024661,1.74130926464116,0.359325238365741));
#6376=CARTESIAN_POINT('Ctrl Pts',(93.0741668361496,1.72365754904715,0.436208821378193));
#6377=CARTESIAN_POINT('Ctrl Pts',(93.0817185902019,1.69333538960863,0.537009883556233));
#6378=CARTESIAN_POINT('Ctrl Pts',(93.0836009048678,1.68514662888125,0.562179103241644));
#6379=CARTESIAN_POINT('Ctrl Pts',(93.0867963251137,1.67010711882088,0.605118550747016));
#6380=CARTESIAN_POINT('Ctrl Pts',(93.0881205895987,1.66352758768491,0.62297856036129));
#6381=CARTESIAN_POINT('Ctrl Pts',(93.0900474752986,1.6534214197674,0.649108907844275));
#6382=CARTESIAN_POINT('Ctrl Pts',(93.0906619087197,1.65011728296532,0.657463099214146));
#6383=CARTESIAN_POINT('Ctrl Pts',(93.0917523113015,1.64410472969126,0.672334364873515));
#6384=CARTESIAN_POINT('Ctrl Pts',(93.0922296507737,1.64142070206472,0.678860769387451));
#6385=CARTESIAN_POINT('Ctrl Pts',(93.0932928280349,1.63532580289314,0.693433448442733));
#6386=CARTESIAN_POINT('Ctrl Pts',(93.0938774328868,1.63189437433871,0.701470732161606));
#6387=CARTESIAN_POINT('Ctrl Pts',(93.0956387291118,1.62131778469842,0.725746109868362));
#6388=CARTESIAN_POINT('Ctrl Pts',(93.0968049954689,1.61398831044527,0.741903341082248));
#6389=CARTESIAN_POINT('Ctrl Pts',(93.1047041262956,1.56220333582018,0.851657850319834));
#6390=CARTESIAN_POINT('Ctrl Pts',(93.1110490402436,1.50986815566692,0.941331004573779));
#6391=CARTESIAN_POINT('Ctrl Pts',(93.1200228189697,1.4254240247358,1.06067981485194));
#6392=CARTESIAN_POINT('Ctrl Pts',(93.1226336321318,1.39960222412412,1.09452676607996));
#6393=CARTESIAN_POINT('Ctrl Pts',(93.1286739926768,1.33760416451959,1.17000746062796));
#6394=CARTESIAN_POINT('Ctrl Pts',(93.1321148882407,1.3006567244868,1.21094747294155));
#6395=CARTESIAN_POINT('Ctrl Pts',(93.1380503393777,1.2350399161863,1.27718187378748));
#6396=CARTESIAN_POINT('Ctrl Pts',(93.1405076003237,1.20734906293717,1.30338982700217));
#6397=CARTESIAN_POINT('Ctrl Pts',(93.1440967365837,1.16633388764828,1.33977936901729));
#6398=CARTESIAN_POINT('Ctrl Pts',(93.1451979582635,1.15367405164561,1.35069598579465));
#6399=CARTESIAN_POINT('Ctrl Pts',(93.1471451291475,1.13117113455504,1.36955313878082));
#6400=CARTESIAN_POINT('Ctrl Pts',(93.1479878656392,1.12139367336679,1.37757037960178));
#6401=CARTESIAN_POINT('Ctrl Pts',(93.1497568955079,1.10079583096589,1.39409542129661));
#6402=CARTESIAN_POINT('Ctrl Pts',(93.1506839155591,1.08996052049543,1.40258317055842));
#6403=CARTESIAN_POINT('Ctrl Pts',(93.1531425857835,1.06112159496285,1.42463791358823));
#6404=CARTESIAN_POINT('Ctrl Pts',(93.1546825163166,1.04295696024656,1.43798919382491));
#6405=CARTESIAN_POINT('Ctrl Pts',(93.1631519334932,0.942546572237878,1.5088889249118));
#6406=CARTESIAN_POINT('Ctrl Pts',(93.1703295816794,0.855802658799709,1.55972293240777));
#6407=CARTESIAN_POINT('Ctrl Pts',(93.1829456264651,0.699390325727027,1.63439359383794));
#6408=CARTESIAN_POINT('Ctrl Pts',(93.1883083752161,0.631661842850541,1.66174381072569));
#6409=CARTESIAN_POINT('Ctrl Pts',(93.1965977045116,0.523415087176101,1.69787916630162));
#6410=CARTESIAN_POINT('Ctrl Pts',(93.1995634411815,0.483943349750302,1.70954855634834));
#6411=CARTESIAN_POINT('Ctrl Pts',(93.2043298501154,0.418829790881935,1.72636230725136));
#6412=CARTESIAN_POINT('Ctrl Pts',(93.2061592774517,0.39341747326498,1.73233024449381));
#6413=CARTESIAN_POINT('Ctrl Pts',(93.2086617840972,0.357949607195601,1.73983884321208));
#6414=CARTESIAN_POINT('Ctrl Pts',(93.2093583023446,0.347999775919662,1.74185627707938));
#6415=CARTESIAN_POINT('Ctrl Pts',(93.2105393151326,0.330985775916135,1.74515443636864));
#6416=CARTESIAN_POINT('Ctrl Pts',(93.2110261277689,0.323930248719547,1.74647782473955));
#6417=CARTESIAN_POINT('Ctrl Pts',(93.2120494716762,0.309005802074096,1.74918360935026));
#6418=CARTESIAN_POINT('Ctrl Pts',(93.2125854386499,0.301135333264894,1.75055574097804));
#6419=CARTESIAN_POINT('Ctrl Pts',(93.2140575032005,0.279378771753651,1.75419768812772));
#6420=CARTESIAN_POINT('Ctrl Pts',(93.214987610092,0.265474211724137,1.75635574435876));
#6421=CARTESIAN_POINT('Ctrl Pts',(93.2213928145935,0.168751189816154,1.77019269873321));
#6422=CARTESIAN_POINT('Ctrl Pts',(93.2265983032021,0.0852129682182508,1.77617609730427));
#6423=CARTESIAN_POINT('Ctrl Pts',(93.2407250864887,-0.144055467551346,1.77637676561385));
#6424=CARTESIAN_POINT('Ctrl Pts',(93.2495338211782,-0.289113125374711,1.75860060391683));
#6425=CARTESIAN_POINT('Ctrl Pts',(93.2605080780151,-0.4538127190016,1.71746960217272));
#6426=CARTESIAN_POINT('Ctrl Pts',(93.2620838103519,-0.477130983352542,1.71113814513665));
#6427=CARTESIAN_POINT('Ctrl Pts',(93.264612310666,-0.513972209549877,1.7003232964099));
#6428=CARTESIAN_POINT('Ctrl Pts',(93.2655550279725,-0.527583389219831,1.69614931301314));
#6429=CARTESIAN_POINT('Ctrl Pts',(93.2672547881802,-0.551892759826345,1.68837372453526));
#6430=CARTESIAN_POINT('Ctrl Pts',(93.2680097951912,-0.562609682777856,1.68483286611478));
#6431=CARTESIAN_POINT('Ctrl Pts',(93.2697910016446,-0.587698442062218,1.67627750860635));
#6432=CARTESIAN_POINT('Ctrl Pts',(93.2708199062474,-0.602040812719904,1.67117999607776));
#6433=CARTESIAN_POINT('Ctrl Pts',(93.2738750850129,-0.644175749433544,1.6555917661869));
#6434=CARTESIAN_POINT('Ctrl Pts',(93.275918225121,-0.671771467834419,1.64458791262244));
#6435=CARTESIAN_POINT('Ctrl Pts',(93.280695107706,-0.734925129995118,1.61755054030976));
#6436=CARTESIAN_POINT('Ctrl Pts',(93.2834437773362,-0.77025579586377,1.60102789692105));
#6437=CARTESIAN_POINT('Ctrl Pts',(93.2941859788216,-0.904557204985671,1.53274623472518));
#6438=CARTESIAN_POINT('Ctrl Pts',(93.3024022874923,-0.999101206697713,1.47286365211513));
#6439=CARTESIAN_POINT('Ctrl Pts',(93.3156278665941,-1.14261128187062,1.3617566443569));
#6440=CARTESIAN_POINT('Ctrl Pts',(93.3206690177548,-1.19527162885448,1.31577716091648));
#6441=CARTESIAN_POINT('Ctrl Pts',(93.3264999739985,-1.25499901315944,1.25707378632538));
#6442=CARTESIAN_POINT('Ctrl Pts',(93.3274598810676,-1.26479194367088,1.2472202678825));
#6443=CARTESIAN_POINT('Ctrl Pts',(93.3289559176588,-1.28000663913058,1.23154791946167));
#6444=CARTESIAN_POINT('Ctrl Pts',(93.3294976887397,-1.28550641137482,1.22580608038096));
#6445=CARTESIAN_POINT('Ctrl Pts',(93.330523869171,-1.29590785623306,1.21479982883754));
#6446=CARTESIAN_POINT('Ctrl Pts',(93.3310087594534,-1.3008163297648,1.20954234069556));
#6447=CARTESIAN_POINT('Ctrl Pts',(93.3321781411007,-1.31263466118435,1.19672851856032));
#6448=CARTESIAN_POINT('Ctrl Pts',(93.3328601930549,-1.31951149890743,1.18914184085805));
#6449=CARTESIAN_POINT('Ctrl Pts',(93.3353048740101,-1.34408221630503,1.16155926800799));
#6450=CARTESIAN_POINT('Ctrl Pts',(93.3370417718139,-1.36139125708832,1.1412234510216));
#6451=CARTESIAN_POINT('Ctrl Pts',(93.3414876257601,-1.40507187595266,1.08749564385176));
#6452=CARTESIAN_POINT('Ctrl Pts',(93.3441607592581,-1.43071480980057,1.05353184774018));
#6453=CARTESIAN_POINT('Ctrl Pts',(93.3546129212042,-1.52713830710726,0.915797181125603));
#6454=CARTESIAN_POINT('Ctrl Pts',(93.3621693425301,-1.58804692661192,0.805570345203826));
#6455=CARTESIAN_POINT('Ctrl Pts',(93.3733550079706,-1.65715815662269,0.641586219267288));
#6456=CARTESIAN_POINT('Ctrl Pts',(93.376695272091,-1.67534926650564,0.592461040548626));
#6457=CARTESIAN_POINT('Ctrl Pts',(93.3813605582293,-1.69722382044454,0.524276612993916));
#6458=CARTESIAN_POINT('Ctrl Pts',(93.3826238986236,-1.70280601142582,0.505852056916281));
#6459=CARTESIAN_POINT('Ctrl Pts',(93.3846759496079,-1.71131911804834,0.476014363890488));
#6460=CARTESIAN_POINT('Ctrl Pts',(93.3854585118966,-1.71443794937603,0.46465611455767));
#6461=CARTESIAN_POINT('Ctrl Pts',(93.3871002172263,-1.72071371056454,0.440877097683268));
#6462=CARTESIAN_POINT('Ctrl Pts',(93.3879599878179,-1.72384963068021,0.428451543188662));
#6463=CARTESIAN_POINT('Ctrl Pts',(93.3900243410106,-1.731018996276,0.398690436958075));
#6464=CARTESIAN_POINT('Ctrl Pts',(93.3912328771392,-1.73492679956393,0.381326356077841));
#6465=CARTESIAN_POINT('Ctrl Pts',(93.3955459623566,-1.74784996919096,0.319585661271104));
#6466=CARTESIAN_POINT('Ctrl Pts',(93.398695155381,-1.75542804394449,0.274929546853203));
#6467=CARTESIAN_POINT('Ctrl Pts',(93.406937362782,-1.770546130218,0.159176547786722));
#6468=CARTESIAN_POINT('Ctrl Pts',(93.4120961228154,-1.77551538882601,0.0878298788422582));
#6469=CARTESIAN_POINT('Ctrl Pts',(93.4255817991173,-1.77722167887632,-0.0971453400352781));
#6470=CARTESIAN_POINT('Ctrl Pts',(93.4339665626487,-1.76738188837031,-0.210518445142822));
#6471=CARTESIAN_POINT('Ctrl Pts',(93.4434999581633,-1.74286401574749,-0.343448354249441));
#6472=CARTESIAN_POINT('Ctrl Pts',(93.445010113681,-1.73855312700722,-0.364643493459479));
#6473=CARTESIAN_POINT('Ctrl Pts',(93.4471023568821,-1.73196136502418,-0.394271479965715));
#6474=CARTESIAN_POINT('Ctrl Pts',(93.4477005507389,-1.73000398653356,-0.402773365964168));
#6475=CARTESIAN_POINT('Ctrl Pts',(93.4487821202922,-1.72633057425892,-0.418207852105489));
#6476=CARTESIAN_POINT('Ctrl Pts',(93.4492666190073,-1.72463522216319,-0.425145171894172));
#6477=CARTESIAN_POINT('Ctrl Pts',(93.450280305827,-1.72098210251948,-0.439712065679702));
#6478=CARTESIAN_POINT('Ctrl Pts',(93.4508089853319,-1.7190153660746,-0.447339105302079));
#6479=CARTESIAN_POINT('Ctrl Pts',(93.4522393713453,-1.71352838647735,-0.468047030342525));
#6480=CARTESIAN_POINT('Ctrl Pts',(93.4531356340948,-1.7099090572664,-0.481101441839765));
#6481=CARTESIAN_POINT('Ctrl Pts',(93.4584283933487,-1.68747505807705,-0.558564504130073));
#6482=CARTESIAN_POINT('Ctrl Pts',(93.4626521376049,-1.66517018725408,-0.621913758129473));
#6483=CARTESIAN_POINT('Ctrl Pts',(93.4760225337471,-1.58217667853029,-0.820864970033614));
#6484=CARTESIAN_POINT('Ctrl Pts',(93.4849280538535,-1.5080766132944,-0.950161368031937));
#6485=CARTESIAN_POINT('Ctrl Pts',(93.4965570197942,-1.39869702116139,-1.09536396913253));
#6486=CARTESIAN_POINT('Ctrl Pts',(93.4987141172584,-1.37789269710149,-1.1214218959304));
#6487=CARTESIAN_POINT('Ctrl Pts',(93.5019425616299,-1.34610353782138,-1.15901772057991));
#6488=CARTESIAN_POINT('Ctrl Pts',(93.5029914300477,-1.33567633931577,-1.17101900086306));
#6489=CARTESIAN_POINT('Ctrl Pts',(93.504880058373,-1.31673426360768,-1.1922383842779));
#6490=CARTESIAN_POINT('Ctrl Pts',(93.5057172442871,-1.30828004865463,-1.20150937837215));
#6491=CARTESIAN_POINT('Ctrl Pts',(93.5075107369181,-1.29005145660743,-1.22107856956718));
#6492=CARTESIAN_POINT('Ctrl Pts',(93.5084681545735,-1.28025044974474,-1.23135064025902));
#6493=CARTESIAN_POINT('Ctrl Pts',(93.5111001692026,-1.25312363174504,-1.25910725599619));
#6494=CARTESIAN_POINT('Ctrl Pts',(93.5127852651667,-1.23555641318794,-1.27635032899491));
#6495=CARTESIAN_POINT('Ctrl Pts',(93.5218488338579,-1.14005899625464,-1.36626622226673));
#6496=CARTESIAN_POINT('Ctrl Pts',(93.5295048007982,-1.05607827440354,-1.43216956662259));
#6497=CARTESIAN_POINT('Ctrl Pts',(93.5459087231474,-0.867457826424393,-1.55453499842616));
#6498=CARTESIAN_POINT('Ctrl Pts',(93.554644472928,-0.762010315445193,-1.60885248446999));
#6499=CARTESIAN_POINT('Ctrl Pts',(93.5640575430095,-0.63682928793766,-1.65824496356577));
#6500=CARTESIAN_POINT('Ctrl Pts',(93.5651842445911,-0.621638060831142,-1.66399941979958));
#6501=CARTESIAN_POINT('Ctrl Pts',(93.5668863550844,-0.598338813046932,-1.67246157628475));
#6502=CARTESIAN_POINT('Ctrl Pts',(93.5674698869663,-0.59028709819039,-1.67532033017041));
#6503=CARTESIAN_POINT('Ctrl Pts',(93.5685252967295,-0.575601581414987,-1.68041538968882));
#6504=CARTESIAN_POINT('Ctrl Pts',(93.5689982214751,-0.568974956954876,-1.68267066415234));
#6505=CARTESIAN_POINT('Ctrl Pts',(93.5700857405124,-0.553631414401922,-1.68779160622621));
#6506=CARTESIAN_POINT('Ctrl Pts',(93.5706986989563,-0.544905417766542,-1.69062897880467));
#6507=CARTESIAN_POINT('Ctrl Pts',(93.5726417421401,-0.517011230177523,-1.69946073265534));
#6508=CARTESIAN_POINT('Ctrl Pts',(93.5739580130385,-0.497762445931506,-1.70519794290838));
#6509=CARTESIAN_POINT('Ctrl Pts',(93.5771055971458,-0.45100612753277,-1.71827466120828));
#6510=CARTESIAN_POINT('Ctrl Pts',(93.5789221977344,-0.423410869793095,-1.72528193366303));
#6511=CARTESIAN_POINT('Ctrl Pts',(93.5864529072088,-0.307103322391783,-1.7518569824724));
#6512=CARTESIAN_POINT('Ctrl Pts',(93.5919807602588,-0.217121954785275,-1.76526923050722));
#6513=CARTESIAN_POINT('Ctrl Pts',(93.6034323668234,-0.031289950246743,-1.77853790610811));
#6514=CARTESIAN_POINT('Ctrl Pts',(93.6093462555186,0.0643074665533043,-1.77764951328542));
#6515=CARTESIAN_POINT('Ctrl Pts',(93.6170688878634,0.183693455887243,-1.76689486791421));
#6516=CARTESIAN_POINT('Ctrl Pts',(93.6186564506637,0.207973532173791,-1.76420171106395));
#6517=CARTESIAN_POINT('Ctrl Pts',(93.6212792864363,0.247596116703773,-1.75897746360971));
#6518=CARTESIAN_POINT('Ctrl Pts',(93.622305249987,0.26297504176311,-1.75674404973668));
#6519=CARTESIAN_POINT('Ctrl Pts',(93.6241692168645,0.290685503937775,-1.75234776705317));
#6520=CARTESIAN_POINT('Ctrl Pts',(93.6250049240221,0.303027362236372,-1.75025574212245));
#6521=CARTESIAN_POINT('Ctrl Pts',(93.6268138063119,0.329558085912075,-1.74546959092179));
#6522=CARTESIAN_POINT('Ctrl Pts',(93.627788295605,0.343738184161768,-1.74273252797948));
#6523=CARTESIAN_POINT('Ctrl Pts',(93.6305189196209,0.383149258995308,-1.73462563824325));
#6524=CARTESIAN_POINT('Ctrl Pts',(93.6322869135237,0.408298102118649,-1.72887882671141));
#6525=CARTESIAN_POINT('Ctrl Pts',(93.6399524352542,0.515715186706416,-1.70185836465579));
#6526=CARTESIAN_POINT('Ctrl Pts',(93.646015449824,0.59651342424197,-1.67524688746557));
#6527=CARTESIAN_POINT('Ctrl Pts',(93.6617358188239,0.796845963813567,-1.5929308214231));
#6528=CARTESIAN_POINT('Ctrl Pts',(93.6715102805786,0.912666063389049,-1.52952104056577));
#6529=CARTESIAN_POINT('Ctrl Pts',(93.6820724513716,1.03551523099174,-1.44329915502099));
#6530=CARTESIAN_POINT('Ctrl Pts',(93.6833591176944,1.05044680101376,-1.43246843854411));
#6531=CARTESIAN_POINT('Ctrl Pts',(93.6852547382454,1.07243127297097,-1.41599318964344));
#6532=CARTESIAN_POINT('Ctrl Pts',(93.6858742416867,1.07961372362891,-1.41052464169013));
#6533=CARTESIAN_POINT('Ctrl Pts',(93.6869822492554,1.09246113672489,-1.40058729792259));
#6534=CARTESIAN_POINT('Ctrl Pts',(93.6874720699532,1.09814114573778,-1.39613829746063));
#6535=CARTESIAN_POINT('Ctrl Pts',(93.6884812926179,1.10984817240773,-1.38685284213382));
#6536=CARTESIAN_POINT('Ctrl Pts',(93.6890003402096,1.11587098882433,-1.38201147374414));
#6537=CARTESIAN_POINT('Ctrl Pts',(93.6903759192982,1.13183075071594,-1.36901005624242));
#6538=CARTESIAN_POINT('Ctrl Pts',(93.6912276931076,1.14171122872236,-1.36078098031617));
#6539=CARTESIAN_POINT('Ctrl Pts',(93.6955973104938,1.1923269147887,-1.31768565801692));
#6540=CARTESIAN_POINT('Ctrl Pts',(93.6990056079059,1.23156152335528,-1.28109186312229));
#6541=CARTESIAN_POINT('Ctrl Pts',(93.7131781827097,1.39013393825072,-1.11916259639066));
#6542=CARTESIAN_POINT('Ctrl Pts',(93.7234471422347,1.49247095608509,-0.978534931265175));
#6543=CARTESIAN_POINT('Ctrl Pts',(93.7361748205297,1.58428348972868,-0.803563249856688));
#6544=CARTESIAN_POINT('Ctrl Pts',(93.7377718249348,1.59524952152713,-0.781566978706564));
#6545=CARTESIAN_POINT('Ctrl Pts',(93.7404070213544,1.61241713724336,-0.74526362825554));
#6546=CARTESIAN_POINT('Ctrl Pts',(93.7414357501652,1.61889315340659,-0.731089482967122));
#6547=CARTESIAN_POINT('Ctrl Pts',(93.7433026555409,1.6302346246133,-0.705376425318109));
#6548=CARTESIAN_POINT('Ctrl Pts',(93.7441385023704,1.635166192292,-0.693867669271847));
#6549=CARTESIAN_POINT('Ctrl Pts',(93.7459453364531,1.64551086646122,-0.669003512251526));
#6550=CARTESIAN_POINT('Ctrl Pts',(93.7469176118721,1.65088390892722,-0.655632525840628));
#6551=CARTESIAN_POINT('Ctrl Pts',(93.7496353783921,1.6653640157855,-0.618291375512968));
#6552=CARTESIAN_POINT('Ctrl Pts',(93.7513925471767,1.67411530134087,-0.594187990619681));
#6553=CARTESIAN_POINT('Ctrl Pts',(93.7596819553197,1.71255342333467,-0.480719815585401));
#6554=CARTESIAN_POINT('Ctrl Pts',(93.7664229787929,1.73562130111621,-0.389287305957905));
#6555=CARTESIAN_POINT('Ctrl Pts',(93.7793509740582,1.76526961856507,-0.214146429622917));
#6556=CARTESIAN_POINT('Ctrl Pts',(93.7854943907676,1.77338001039965,-0.130964135309562));
#6557=CARTESIAN_POINT('Ctrl Pts',(93.7915308013958,1.77561364010973,-0.0475422291890938));
#6558=CARTESIAN_POINT('Origin',(88.3562164250559,0.,0.));
#6559=CARTESIAN_POINT('',(94.6900676319115,1.77561363837053,-0.0475422941449777));
#6560=CARTESIAN_POINT('',(94.5412649413994,1.77561364082572,-0.0475422024484503));
#6561=CARTESIAN_POINT('',(88.3562164250559,1.77561363837197,-0.0475422940912398));
#6562=CARTESIAN_POINT('Ctrl Pts',(94.6900676319115,1.77561363837053,-0.0475422941449777));
#6563=CARTESIAN_POINT('Ctrl Pts',(94.6893507188366,1.77532856922536,-0.0581890807830827));
#6564=CARTESIAN_POINT('Ctrl Pts',(94.6886308105993,1.77494775027251,-0.0688329602318011));
#6565=CARTESIAN_POINT('Ctrl Pts',(94.6861831815559,1.77333438493924,-0.104856300293904));
#6566=CARTESIAN_POINT('Ctrl Pts',(94.684441590984,1.77165305712317,-0.130211417406875));
#6567=CARTESIAN_POINT('Ctrl Pts',(94.672685378898,1.75677823088517,-0.299449024897515));
#6568=CARTESIAN_POINT('Ctrl Pts',(94.6621304716666,1.72661593432615,-0.441272503813269));
#6569=CARTESIAN_POINT('Ctrl Pts',(94.6455425341743,1.65275463930097,-0.655965845456816));
#6570=CARTESIAN_POINT('Ctrl Pts',(94.6395427093636,1.62045850308286,-0.732124515511155));
#6571=CARTESIAN_POINT('Ctrl Pts',(94.632811709424,1.57661523445818,-0.818257267904971));
#6572=CARTESIAN_POINT('Ctrl Pts',(94.6318428774882,1.57010851206846,-0.830674331617518));
#6573=CARTESIAN_POINT('Ctrl Pts',(94.6303361219136,1.5596689104266,-0.850035645395027));
#6574=CARTESIAN_POINT('Ctrl Pts',(94.6297924283201,1.55583523908449,-0.857032335277985));
#6575=CARTESIAN_POINT('Ctrl Pts',(94.6287649541035,1.5484605815015,-0.870278968726304));
#6576=CARTESIAN_POINT('Ctrl Pts',(94.6282806669416,1.54492867308116,-0.876533543389885));
#6577=CARTESIAN_POINT('Ctrl Pts',(94.6271159235648,1.53630071661163,-0.891598427471945));
#6578=CARTESIAN_POINT('Ctrl Pts',(94.6264378566784,1.53116661300014,-0.900386840922093));
#6579=CARTESIAN_POINT('Ctrl Pts',(94.6241488730038,1.51346745543387,-0.930094504792485));
#6580=CARTESIAN_POINT('Ctrl Pts',(94.6225587920112,1.500546390029,-0.950799768317442));
#6581=CARTESIAN_POINT('Ctrl Pts',(94.6109807819324,1.4021882411966,-1.10141077228003));
#6582=CARTESIAN_POINT('Ctrl Pts',(94.6017564364994,1.30044293397444,-1.21987593943647));
#6583=CARTESIAN_POINT('Ctrl Pts',(94.587963495248,1.13560490190286,-1.36739958152182));
#6584=CARTESIAN_POINT('Ctrl Pts',(94.5838025110408,1.08426244929982,-1.40845789016199));
#6585=CARTESIAN_POINT('Ctrl Pts',(94.5782210040343,1.01439392352613,-1.45824321403634));
#6586=CARTESIAN_POINT('Ctrl Pts',(94.5769030623765,0.997823487867752,-1.46963142879174));
#6587=CARTESIAN_POINT('Ctrl Pts',(94.5746984269852,0.970012038421088,-1.48805795181153));
#6588=CARTESIAN_POINT('Ctrl Pts',(94.5738178060399,0.958878854639757,-1.4952562150192));
#6589=CARTESIAN_POINT('Ctrl Pts',(94.5720818626744,0.93689257722526,-1.50912511848459));
#6590=CARTESIAN_POINT('Ctrl Pts',(94.5712269505008,0.926046222199189,-1.51580496904516));
#6591=CARTESIAN_POINT('Ctrl Pts',(94.5691478006734,0.899629571228397,-1.5316846102644));
#6592=CARTESIAN_POINT('Ctrl Pts',(94.56791928755,0.883989078416313,-1.54076421872661));
#6593=CARTESIAN_POINT('Ctrl Pts',(94.5636696552796,0.829797306962036,-1.57112683751982));
#6594=CARTESIAN_POINT('Ctrl Pts',(94.5606070933443,0.790597533044739,-1.59121276569145));
#6595=CARTESIAN_POINT('Ctrl Pts',(94.5487779965292,0.638703686695453,-1.66204423178195));
#6596=CARTESIAN_POINT('Ctrl Pts',(94.5397031430995,0.521579601218354,-1.70243379138357));
#6597=CARTESIAN_POINT('Ctrl Pts',(94.5256520476236,0.333967789323071,-1.74593742228245));
#6598=CARTESIAN_POINT('Ctrl Pts',(94.5206527168306,0.265843401143473,-1.7576009467397));
#6599=CARTESIAN_POINT('Ctrl Pts',(94.5145985063424,0.179954812375146,-1.76719599453683));
#6600=CARTESIAN_POINT('Ctrl Pts',(94.51339303078,0.162674405236508,-1.76887040560473));
#6601=CARTESIAN_POINT('Ctrl Pts',(94.5116051043233,0.136735611545647,-1.77100042786057));
#6602=CARTESIAN_POINT('Ctrl Pts',(94.5110130608204,0.12809447879119,-1.77164639682497));
#6603=CARTESIAN_POINT('Ctrl Pts',(94.5099449968422,0.112404824509095,-1.77270388391908));
#6604=CARTESIAN_POINT('Ctrl Pts',(94.5094678728085,0.105358286915062,-1.77313663876991));
#6605=CARTESIAN_POINT('Ctrl Pts',(94.50838327894,0.089255181541533,-1.77402925500626));
#6606=CARTESIAN_POINT('Ctrl Pts',(94.507777313679,0.0801974592629025,-1.77446179488423));
#6607=CARTESIAN_POINT('Ctrl Pts',(94.5059255905719,0.0523467292729324,-1.77557807713393));
#6608=CARTESIAN_POINT('Ctrl Pts',(94.5046916092063,0.0335451859166894,-1.77603279178416));
#6609=CARTESIAN_POINT('Ctrl Pts',(94.4959055546058,-0.101737711041205,-1.77715538839417));
#6610=CARTESIAN_POINT('Ctrl Pts',(94.4888337047168,-0.218042611905205,-1.76666248030984));
#6611=CARTESIAN_POINT('Ctrl Pts',(94.4772276850087,-0.403639267370296,-1.73129570381198));
#6612=CARTESIAN_POINT('Ctrl Pts',(94.4727598165035,-0.473884813714225,-1.71340059811568));
#6613=CARTESIAN_POINT('Ctrl Pts',(94.465292932081,-0.586319443726679,-1.67731302049721));
#6614=CARTESIAN_POINT('Ctrl Pts',(94.4623647378626,-0.629243204801126,-1.66168646304877));
#6615=CARTESIAN_POINT('Ctrl Pts',(94.4582165786619,-0.688041670339702,-1.63767561272757));
#6616=CARTESIAN_POINT('Ctrl Pts',(94.4570426939154,-0.70446547492639,-1.63067811324624));
#6617=CARTESIAN_POINT('Ctrl Pts',(94.455011021815,-0.732502024566366,-1.61823030589288));
#6618=CARTESIAN_POINT('Ctrl Pts',(94.4541573588965,-0.7441665278786,-1.61289947081182));
#6619=CARTESIAN_POINT('Ctrl Pts',(94.4525119703957,-0.766421460956895,-1.6024358607059));
#6620=CARTESIAN_POINT('Ctrl Pts',(94.4517209782419,-0.77702064512725,-1.59732321367596));
#6621=CARTESIAN_POINT('Ctrl Pts',(94.4496304809519,-0.804766808166873,-1.58359800028559));
#6622=CARTESIAN_POINT('Ctrl Pts',(94.4483249879578,-0.821825984324407,-1.57481244694178));
#6623=CARTESIAN_POINT('Ctrl Pts',(94.4434575053143,-0.88442219282675,-1.54128104622225));
#6624=CARTESIAN_POINT('Ctrl Pts',(94.4398360799854,-0.929008174541551,-1.51482433084457));
#6625=CARTESIAN_POINT('Ctrl Pts',(94.4271947209366,-1.07794586309346,-1.4173964114197));
#6626=CARTESIAN_POINT('Ctrl Pts',(94.4178878589543,-1.17585590146043,-1.33728696467246));
#6627=CARTESIAN_POINT('Ctrl Pts',(94.4056201385905,-1.29437266646587,-1.21716050776564));
#6628=CARTESIAN_POINT('Ctrl Pts',(94.4025450538604,-1.32320413351825,-1.18575358721403));
#6629=CARTESIAN_POINT('Ctrl Pts',(94.3976258957773,-1.36823721063815,-1.13300733898302));
#6630=CARTESIAN_POINT('Ctrl Pts',(94.3957509476169,-1.3851349601193,-1.11228594502442));
#6631=CARTESIAN_POINT('Ctrl Pts',(94.3931976575987,-1.40785265865109,-1.08310659393943));
#6632=CARTESIAN_POINT('Ctrl Pts',(94.3924946593182,-1.41407593190208,-1.07496896412983));
#6633=CARTESIAN_POINT('Ctrl Pts',(94.391306135188,-1.42454884714041,-1.06102610229231));
#6634=CARTESIAN_POINT('Ctrl Pts',(94.390818216899,-1.42883419686183,-1.05524814772104));
#6635=CARTESIAN_POINT('Ctrl Pts',(94.3897963916073,-1.43778092291671,-1.04303080777599));
#6636=CARTESIAN_POINT('Ctrl Pts',(94.389263009363,-1.44243433239643,-1.03658595938198));
#6637=CARTESIAN_POINT('Ctrl Pts',(94.3878058151533,-1.45509552981737,-1.01880017295125));
#6638=CARTESIAN_POINT('Ctrl Pts',(94.3868877959095,-1.46301406768841,-1.00739598004195));
#6639=CARTESIAN_POINT('Ctrl Pts',(94.3814164753894,-1.50979026480077,-0.938314368615776));
#6640=CARTESIAN_POINT('Ctrl Pts',(94.377047863597,-1.5453713826048,-0.878481684298969));
#6641=CARTESIAN_POINT('Ctrl Pts',(94.365808397107,-1.62880740975325,-0.717337255263666));
#6642=CARTESIAN_POINT('Ctrl Pts',(94.3590454624897,-1.67075320347701,-0.613327101261384));
#6643=CARTESIAN_POINT('Ctrl Pts',(94.3495897174998,-1.71375539714512,-0.468647005802481));
#6644=CARTESIAN_POINT('Ctrl Pts',(94.3471190248123,-1.72363898506094,-0.430878089029393));
#6645=CARTESIAN_POINT('Ctrl Pts',(94.3427032352319,-1.73884417224729,-0.363825095701174));
#6646=CARTESIAN_POINT('Ctrl Pts',(94.3407740140183,-1.74468912146665,-0.33467515565165));
#6647=CARTESIAN_POINT('Ctrl Pts',(94.337821830731,-1.75241740741335,-0.290394749305998));
#6648=CARTESIAN_POINT('Ctrl Pts',(94.336815974141,-1.75484213526017,-0.275363280772692));
#6649=CARTESIAN_POINT('Ctrl Pts',(94.3350537127347,-1.75872740736911,-0.249137263893315));
#6650=CARTESIAN_POINT('Ctrl Pts',(94.3343001116945,-1.76027504385336,-0.237956360619245));
#6651=CARTESIAN_POINT('Ctrl Pts',(94.3325884618629,-1.76353318301943,-0.212643813446523));
#6652=CARTESIAN_POINT('Ctrl Pts',(94.3316284728975,-1.76518056626541,-0.198504979566883));
#6653=CARTESIAN_POINT('Ctrl Pts',(94.3290252186059,-1.76916411776666,-0.160329551780577));
#6654=CARTESIAN_POINT('Ctrl Pts',(94.3273720755818,-1.77118023882369,-0.136263356070453));
#6655=CARTESIAN_POINT('Ctrl Pts',(94.3156374423573,-1.78190649835909,0.0332598718152109));
#6656=CARTESIAN_POINT('Ctrl Pts',(94.3050002933125,-1.77317629156353,0.179239185134527));
#6657=CARTESIAN_POINT('Ctrl Pts',(94.2887489612861,-1.73279864228695,0.39794817120223));
#6658=CARTESIAN_POINT('Ctrl Pts',(94.2831701989557,-1.71398765014958,0.47244305254472));
#6659=CARTESIAN_POINT('Ctrl Pts',(94.2765104011753,-1.68482978432634,0.562799568571997));
#6660=CARTESIAN_POINT('Ctrl Pts',(94.2752463043161,-1.67897938637629,0.580019862442365));
#6661=CARTESIAN_POINT('Ctrl Pts',(94.2733896120474,-1.66989862683795,0.605458924886001));
#6662=CARTESIAN_POINT('Ctrl Pts',(94.2727863537017,-1.66687000579552,0.613747770479729));
#6663=CARTESIAN_POINT('Ctrl Pts',(94.2717072831879,-1.66130891905485,0.628622715697216));
#6664=CARTESIAN_POINT('Ctrl Pts',(94.2712302331037,-1.65879886427694,0.635216636647327));
#6665=CARTESIAN_POINT('Ctrl Pts',(94.2701571770449,-1.65303607590358,0.650088368204042));
#6666=CARTESIAN_POINT('Ctrl Pts',(94.2695625324339,-1.64976039424339,0.658356897702939));
#6667=CARTESIAN_POINT('Ctrl Pts',(94.2677382642813,-1.6394617170447,0.683793378087505));
#6668=CARTESIAN_POINT('Ctrl Pts',(94.2665201854244,-1.63223156185939,0.700876808455042));
#6669=CARTESIAN_POINT('Ctrl Pts',(94.256608396622,-1.57060314459081,0.840363578805335));
#6670=CARTESIAN_POINT('Ctrl Pts',(94.2485557334798,-1.50277959030219,0.956383076887852));
#6671=CARTESIAN_POINT('Ctrl Pts',(94.2350372554962,-1.37142176960472,1.13205785874908));
#6672=CARTESIAN_POINT('Ctrl Pts',(94.2297162348126,-1.31543982584207,1.19664879509923));
#6673=CARTESIAN_POINT('Ctrl Pts',(94.2225401240605,-1.23674222722124,1.27522585634183));
#6674=CARTESIAN_POINT('Ctrl Pts',(94.2208564144403,-1.21805327461654,1.2930887171653));
#6675=CARTESIAN_POINT('Ctrl Pts',(94.2182040679773,-1.18831805343466,1.32029283383892));
#6676=CARTESIAN_POINT('Ctrl Pts',(94.2172475301206,-1.17753577151877,1.32991821147911));
#6677=CARTESIAN_POINT('Ctrl Pts',(94.2154522205512,-1.15719859193177,1.34763205839611));
#6678=CARTESIAN_POINT('Ctrl Pts',(94.2146148843366,-1.14767326845435,1.3557532227556));
#6679=CARTESIAN_POINT('Ctrl Pts',(94.2127295784184,-1.12614285228857,1.37372027078897));
#6680=CARTESIAN_POINT('Ctrl Pts',(94.2116794405166,-1.11409302617292,1.38351068244152));
#6681=CARTESIAN_POINT('Ctrl Pts',(94.2089639720216,-1.08279773853364,1.40826394574645));
#6682=CARTESIAN_POINT('Ctrl Pts',(94.2072895382155,-1.06337033869011,1.42299040885461));
#6683=CARTESIAN_POINT('Ctrl Pts',(94.1974899910886,-0.948971506818882,1.5060565745101));
#6684=CARTESIAN_POINT('Ctrl Pts',(94.1890276594979,-0.847751034353264,1.56526766842386));
#6685=CARTESIAN_POINT('Ctrl Pts',(94.175033136049,-0.673806282369953,1.64517257531713));
#6686=CARTESIAN_POINT('Ctrl Pts',(94.1695745905638,-0.604257828579552,1.67196923334007));
#6687=CARTESIAN_POINT('Ctrl Pts',(94.1623978404426,-0.508746285298949,1.70202823864681));
#6688=CARTESIAN_POINT('Ctrl Pts',(94.1605737214393,-0.48409674181734,1.70920255962396));
#6689=CARTESIAN_POINT('Ctrl Pts',(94.1574660661137,-0.441326924526078,1.7206512582471));
#6690=CARTESIAN_POINT('Ctrl Pts',(94.1561721174691,-0.423279337843018,1.72517966524375));
#6691=CARTESIAN_POINT('Ctrl Pts',(94.1542805455314,-0.396493761742497,1.73145489147676));
#6692=CARTESIAN_POINT('Ctrl Pts',(94.1536716955606,-0.387809074147365,1.7334207437585));
#6693=CARTESIAN_POINT('Ctrl Pts',(94.1525869896593,-0.372216694057411,1.7368271580589));
#6694=CARTESIAN_POINT('Ctrl Pts',(94.1521098294717,-0.365314815660281,1.73829195892311));
#6695=CARTESIAN_POINT('Ctrl Pts',(94.1510418766553,-0.349771159297787,1.74149415369455));
#6696=CARTESIAN_POINT('Ctrl Pts',(94.1504523796679,-0.34112498197185,1.74320839435481));
#6697=CARTESIAN_POINT('Ctrl Pts',(94.1486606026384,-0.314655763585711,1.74825185262594));
#6698=CARTESIAN_POINT('Ctrl Pts',(94.1474692822927,-0.296793587058729,1.75137272416074));
#6699=CARTESIAN_POINT('Ctrl Pts',(94.1402507099039,-0.18719141575427,1.76879728195943));
#6700=CARTESIAN_POINT('Ctrl Pts',(94.1345305521696,-0.0944832916806178,
1.77616485190593));
#6701=CARTESIAN_POINT('Ctrl Pts',(94.1211072459206,0.124062194002053,1.7763635018049));
#6702=CARTESIAN_POINT('Ctrl Pts',(94.1134354308902,0.249382072983139,1.76314017233794));
#6703=CARTESIAN_POINT('Ctrl Pts',(94.1037857514685,0.395758592039518,1.7317670536397));
#6704=CARTESIAN_POINT('Ctrl Pts',(94.102222699047,0.419159227200112,1.7262524279553));
#6705=CARTESIAN_POINT('Ctrl Pts',(94.0996319497146,0.457381321142991,1.71642197715427));
#6706=CARTESIAN_POINT('Ctrl Pts',(94.0986131679651,0.472271655514866,1.71238475083716));
#6707=CARTESIAN_POINT('Ctrl Pts',(94.0967567477616,0.499138899895942,1.70472313198146));
#6708=CARTESIAN_POINT('Ctrl Pts',(94.0959213179238,0.511133810466153,1.70116513370024));
#6709=CARTESIAN_POINT('Ctrl Pts',(94.0941067450424,0.536973714200472,1.6932023973668));
#6710=CARTESIAN_POINT('Ctrl Pts',(94.0931262177289,0.550804168837922,1.68875394119343));
#6711=CARTESIAN_POINT('Ctrl Pts',(94.0903605171287,0.589434477825859,1.67580378598754));
#6712=CARTESIAN_POINT('Ctrl Pts',(94.0885629837096,0.614102057187853,1.66692227421533));
#6713=CARTESIAN_POINT('Ctrl Pts',(94.08064705375,0.720779724255802,1.62582395349118));
#6714=CARTESIAN_POINT('Ctrl Pts',(94.0743500233791,0.800514041173156,1.5880806627173));
#6715=CARTESIAN_POINT('Ctrl Pts',(94.0636341060031,0.928736585387347,1.51526802133098));
#6716=CARTESIAN_POINT('Ctrl Pts',(94.0592811121909,0.978860053808308,1.48338180427142));
#6717=CARTESIAN_POINT('Ctrl Pts',(94.049209552882,1.09138927152295,1.40360499193183));
#6718=CARTESIAN_POINT('Ctrl Pts',(94.0435138787308,1.15240853706415,1.3539552333509));
#6719=CARTESIAN_POINT('Ctrl Pts',(94.0370631143474,1.2202189990265,1.29086273863887));
#6720=CARTESIAN_POINT('Ctrl Pts',(94.0360931201038,1.23038027722571,1.28118125961192));
#6721=CARTESIAN_POINT('Ctrl Pts',(94.0345849706424,1.24613892918658,1.26580627822359));
#6722=CARTESIAN_POINT('Ctrl Pts',(94.0340410286497,1.25181423795601,1.26019398696335));
#6723=CARTESIAN_POINT('Ctrl Pts',(94.0330133879427,1.26252392649933,1.24945947219386));
#6724=CARTESIAN_POINT('Ctrl Pts',(94.032529179365,1.26756529886373,1.24434474824296));
#6725=CARTESIAN_POINT('Ctrl Pts',(94.0313650360795,1.27967052803989,1.23191348153976));
#6726=CARTESIAN_POINT('Ctrl Pts',(94.0306874842556,1.28670295459727,1.22456645604751));
#6727=CARTESIAN_POINT('Ctrl Pts',(94.0282786440752,1.31163905321841,1.19806282812318));
#6728=CARTESIAN_POINT('Ctrl Pts',(94.0265721063015,1.32918211883409,1.17856973272622));
#6729=CARTESIAN_POINT('Ctrl Pts',(94.0222259608199,1.37331018923433,1.12729727115831));
#6730=CARTESIAN_POINT('Ctrl Pts',(94.0196201925805,1.39922737645146,1.09496264935401));
#6731=CARTESIAN_POINT('Ctrl Pts',(94.0121665066269,1.47082950822803,0.99893166328431));
#6732=CARTESIAN_POINT('Ctrl Pts',(94.0073958457916,1.51346045508009,0.93308201223802));
#6733=CARTESIAN_POINT('Ctrl Pts',(93.9967111760042,1.59791977048567,0.781517385489466));
#6734=CARTESIAN_POINT('Ctrl Pts',(93.9907839085201,1.63747641358145,0.694827125005744));
#6735=CARTESIAN_POINT('Ctrl Pts',(93.9831734663719,1.67747553060869,0.584494698040664));
#6736=CARTESIAN_POINT('Ctrl Pts',(93.9817200599898,1.684658625819,0.563456697769412));
#6737=CARTESIAN_POINT('Ctrl Pts',(93.9793500497264,1.69562690680731,0.529245785857968));
#6738=CARTESIAN_POINT('Ctrl Pts',(93.9784415591389,1.69965789995779,0.516153769966571));
#6739=CARTESIAN_POINT('Ctrl Pts',(93.9766834126647,1.70712392480102,0.490869026476544));
#6740=CARTESIAN_POINT('Ctrl Pts',(93.9758345308789,1.71058075560855,0.478683569731445));
#6741=CARTESIAN_POINT('Ctrl Pts',(93.9738450847763,1.71833685726729,0.45018559306448));
#6742=CARTESIAN_POINT('Ctrl Pts',(93.9727013100048,1.72253458634699,0.433846963532261));
#6743=CARTESIAN_POINT('Ctrl Pts',(93.9688837436778,1.73567971159305,0.379481262805467));
#6744=CARTESIAN_POINT('Ctrl Pts',(93.966177910031,1.74360480179457,0.341221293699562));
#6745=CARTESIAN_POINT('Ctrl Pts',(93.9594249809633,1.75999662247539,0.246451595404281));
#6746=CARTESIAN_POINT('Ctrl Pts',(93.9553391945997,1.76701020958113,0.189737654203443));
#6747=CARTESIAN_POINT('Ctrl Pts',(93.9483782134909,1.77419824065539,0.0938560027675912));
#6748=CARTESIAN_POINT('Ctrl Pts',(93.9455312101927,1.7758324567088,0.054838590856963));
#6749=CARTESIAN_POINT('Ctrl Pts',(93.9411336659243,1.77636761854763,-0.00532194227614969));
#6750=CARTESIAN_POINT('Ctrl Pts',(93.9395886383419,1.77617867042149,-0.0264394646778253));
#6751=CARTESIAN_POINT('Ctrl Pts',(93.938045236354,1.77561363622783,-0.0475423741708462));
#6752=CARTESIAN_POINT('',(93.9795659395437,0.000115947507982164,1.77624999621567));
#6753=CARTESIAN_POINT('Ctrl Pts',(93.7915308013958,1.77561364010973,-0.0475422291890938));
#6754=CARTESIAN_POINT('Ctrl Pts',(93.7928573604259,1.77610450162403,-0.0292094666102127));
#6755=CARTESIAN_POINT('Ctrl Pts',(93.7941784581398,1.77631154895408,-0.0108651108999133));
#6756=CARTESIAN_POINT('Ctrl Pts',(93.7980361553455,1.77608444226741,0.0430336293841766));
#6757=CARTESIAN_POINT('Ctrl Pts',(93.8005493957931,1.77486745046972,0.0785733486572298));
#6758=CARTESIAN_POINT('Ctrl Pts',(93.8038236861351,1.77183360385389,0.125723749035798));
#6759=CARTESIAN_POINT('Ctrl Pts',(93.8046285780797,1.77096757914434,0.137384980726422));
#6760=CARTESIAN_POINT('Ctrl Pts',(93.8058874411011,1.76942135888394,0.155748107009445));
#6761=CARTESIAN_POINT('Ctrl Pts',(93.8063454709787,1.76881810978186,0.162455890798343));
#6762=CARTESIAN_POINT('Ctrl Pts',(93.8072973684724,1.76747881301121,0.176455123791574));
#6763=CARTESIAN_POINT('Ctrl Pts',(93.8077907979097,1.76673577018263,0.183745710675326));
#6764=CARTESIAN_POINT('Ctrl Pts',(93.8090176475938,1.7647663778025,0.201951305055927));
#6765=CARTESIAN_POINT('Ctrl Pts',(93.8097480090473,1.76348384235142,0.212860167457891));
#6766=CARTESIAN_POINT('Ctrl Pts',(93.812610738017,1.75802323951052,0.25586279455385));
#6767=CARTESIAN_POINT('Ctrl Pts',(93.8147044347149,1.75306930253835,0.287853799522207));
#6768=CARTESIAN_POINT('Ctrl Pts',(93.8204090383504,1.73696583841422,0.375865112932617));
#6769=CARTESIAN_POINT('Ctrl Pts',(93.8239538103413,1.72398465243174,0.431512135220726));
#6770=CARTESIAN_POINT('Ctrl Pts',(93.8364607367806,1.66840000086416,0.62672147590001));
#6771=CARTESIAN_POINT('Ctrl Pts',(93.8452834387934,1.61133507624045,0.761533810506193));
#6772=CARTESIAN_POINT('Ctrl Pts',(93.8562719304892,1.52637631443935,0.908747203367535));
#6773=CARTESIAN_POINT('Ctrl Pts',(93.857845444609,1.51389298538698,0.929394464576138));
#6774=CARTESIAN_POINT('Ctrl Pts',(93.8603712013899,1.49338508334739,0.961804304282125));
#6775=CARTESIAN_POINT('Ctrl Pts',(93.8613134316003,1.48563266934305,0.973736144355019));
#6776=CARTESIAN_POINT('Ctrl Pts',(93.8630127762464,1.47147483562486,0.994963960133127));
#6777=CARTESIAN_POINT('Ctrl Pts',(93.8637678611087,1.46512249966352,1.00429454079167));
#6778=CARTESIAN_POINT('Ctrl Pts',(93.8655498658519,1.44999036387896,1.02607212574692));
#6779=CARTESIAN_POINT('Ctrl Pts',(93.8665794986688,1.44113865174967,1.03846782509942));
#6780=CARTESIAN_POINT('Ctrl Pts',(93.8696391498019,1.41452427399495,1.07474219791824));
#6781=CARTESIAN_POINT('Ctrl Pts',(93.8716861089007,1.39632044878063,1.09828900201252));
#6782=CARTESIAN_POINT('Ctrl Pts',(93.8764736987312,1.35285618195068,1.15168238188039));
#6783=CARTESIAN_POINT('Ctrl Pts',(93.8792293519519,1.32718531840914,1.1811735293513));
#6784=CARTESIAN_POINT('Ctrl Pts',(93.8900232902046,1.22408627105126,1.29200820653384));
#6785=CARTESIAN_POINT('Ctrl Pts',(93.8982868212188,1.13998935857522,1.36678178112968));
#6786=CARTESIAN_POINT('Ctrl Pts',(93.9114994856624,0.993669003969397,1.47392637938748));
#6787=CARTESIAN_POINT('Ctrl Pts',(93.9164843357838,0.935588284761137,1.51146077610724));
#6788=CARTESIAN_POINT('Ctrl Pts',(93.922260891919,0.863396848085454,1.55235377511014));
#6789=CARTESIAN_POINT('Ctrl Pts',(93.9232191022768,0.851250909193058,1.55904723466866));
#6790=CARTESIAN_POINT('Ctrl Pts',(93.9247131027331,0.83202422117582,1.5693511039708));
#6791=CARTESIAN_POINT('Ctrl Pts',(93.9252545100866,0.824995802865499,1.57305725376944));
#6792=CARTESIAN_POINT('Ctrl Pts',(93.926280454821,0.811556197828013,1.58002922829377));
#6793=CARTESIAN_POINT('Ctrl Pts',(93.9267654682168,0.805149753671243,1.58330341387512));
#6794=CARTESIAN_POINT('Ctrl Pts',(93.9279357653475,0.789567228979204,1.59114824537304));
#6795=CARTESIAN_POINT('Ctrl Pts',(93.9286185998461,0.780370972218809,1.5956786349831));
#6796=CARTESIAN_POINT('Ctrl Pts',(93.9310695456324,0.747007764903059,1.61175706163288));
#6797=CARTESIAN_POINT('Ctrl Pts',(93.9328117523522,0.722618314996183,1.62283837202576));
#6798=CARTESIAN_POINT('Ctrl Pts',(93.937275144223,0.658686546528779,1.65015834980396));
#6799=CARTESIAN_POINT('Ctrl Pts',(93.9399601517045,0.618791118764905,1.6655295168743));
#6800=CARTESIAN_POINT('Ctrl Pts',(93.9514338938808,0.444256618011175,1.72563669884012));
#6801=CARTESIAN_POINT('Ctrl Pts',(93.9599404123782,0.30509109801814,1.75559272208157));
#6802=CARTESIAN_POINT('Ctrl Pts',(93.9712136706598,0.128318363072791,1.77196819027313));
#6803=CARTESIAN_POINT('Ctrl Pts',(93.9735051847306,0.0927049881957018,1.77418781121198));
#6804=CARTESIAN_POINT('Ctrl Pts',(93.9765702297719,0.0456782895515519,1.77569902331361));
#6805=CARTESIAN_POINT('Ctrl Pts',(93.9773146368292,0.0343028600437258,1.7759551885171));
#6806=CARTESIAN_POINT('Ctrl Pts',(93.9785620793822,0.0153229027538503,1.7762001822216));
#6807=CARTESIAN_POINT('Ctrl Pts',(93.9790632566766,0.00771940838996888,
1.77624949988782));
#6808=CARTESIAN_POINT('Ctrl Pts',(93.9795659395437,0.000115947507982164,
1.77624999621567));
#6809=CARTESIAN_POINT('Ctrl Pts',(93.9795659773891,0.000115375067715305,
1.77624999625295));
#6810=CARTESIAN_POINT('Ctrl Pts',(93.9799864663399,-0.00624483932767286,
1.77625040937619));
#6811=CARTESIAN_POINT('Ctrl Pts',(93.9804080037495,-0.0126049561014548,
1.77621666149281));
#6812=CARTESIAN_POINT('Ctrl Pts',(93.9813988129797,-0.0275156646565273,
1.77605745346026));
#6813=CARTESIAN_POINT('Ctrl Pts',(93.9819689297411,-0.0360657251495172,
1.77590440307868));
#6814=CARTESIAN_POINT('Ctrl Pts',(93.98343137621,-0.0579197181264248,1.77535532127359));
#6815=CARTESIAN_POINT('Ctrl Pts',(93.9843264205943,-0.0712207125656861,
1.77487148939002));
#6816=CARTESIAN_POINT('Ctrl Pts',(93.9865529071123,-0.104117071083033,1.77330449236378));
#6817=CARTESIAN_POINT('Ctrl Pts',(93.9878897449017,-0.123701896461083,1.77204598528339));
#6818=CARTESIAN_POINT('Ctrl Pts',(93.9933456945305,-0.2029310194927,1.76563497522455));
#6819=CARTESIAN_POINT('Ctrl Pts',(93.9975467803286,-0.262312007469336,1.7577937473307));
#6820=CARTESIAN_POINT('Ctrl Pts',(94.0054540066584,-0.371190145239888,1.73777663948774));
#6821=CARTESIAN_POINT('Ctrl Pts',(94.0091355111197,-0.420781041899192,1.72643926139459));
#6822=CARTESIAN_POINT('Ctrl Pts',(94.0178024421711,-0.535457364390115,1.69498748429302));
#6823=CARTESIAN_POINT('Ctrl Pts',(94.0228014371669,-0.600010798160375,1.67322569972188));
#6824=CARTESIAN_POINT('Ctrl Pts',(94.0321368688422,-0.719254663214412,1.62523645610704));
#6825=CARTESIAN_POINT('Ctrl Pts',(94.0364784444672,-0.774169849893795,1.59980729644811));
#6826=CARTESIAN_POINT('Ctrl Pts',(94.0416052622191,-0.839404867044646,1.56545167934388));
#6827=CARTESIAN_POINT('Ctrl Pts',(94.0425195532581,-0.85105502554311,1.55914876165928));
#6828=CARTESIAN_POINT('Ctrl Pts',(94.0439607772313,-0.86946219420347,1.54892238990078));
#6829=CARTESIAN_POINT('Ctrl Pts',(94.0444927125386,-0.876265440262095,1.54508380394872));
#6830=CARTESIAN_POINT('Ctrl Pts',(94.0455073951989,-0.889265132637704,1.53763552431227));
#6831=CARTESIAN_POINT('Ctrl Pts',(94.045990545695,-0.895465337666658,1.53403302203291));
#6832=CARTESIAN_POINT('Ctrl Pts',(94.0470646539551,-0.909267801341845,1.52590118690606));
#6833=CARTESIAN_POINT('Ctrl Pts',(94.0476543797019,-0.916858479024284,1.52135232747974));
#6834=CARTESIAN_POINT('Ctrl Pts',(94.0496987468193,-0.943201959374167,1.50529670814512));
#6835=CARTESIAN_POINT('Ctrl Pts',(94.0511360833147,-0.961775557561119,1.4934979071862));
#6836=CARTESIAN_POINT('Ctrl Pts',(94.0608948230114,-1.08779375687798,1.41011910048729));
#6837=CARTESIAN_POINT('Ctrl Pts',(94.068663302468,-1.18738682820815,1.32734764794752));
#6838=CARTESIAN_POINT('Ctrl Pts',(94.0818336518972,-1.3358705542575,1.173736001161));
#6839=CARTESIAN_POINT('Ctrl Pts',(94.0871037402546,-1.39018901868765,1.10886360070515));
#6840=CARTESIAN_POINT('Ctrl Pts',(94.0942177698618,-1.45475314108468,1.01951927736893));
#6841=CARTESIAN_POINT('Ctrl Pts',(94.0958940188898,-1.46936975471025,0.998337955199077));
#6842=CARTESIAN_POINT('Ctrl Pts',(94.0985372043243,-1.49145570736709,0.964796418837553));
#6843=CARTESIAN_POINT('Ctrl Pts',(94.0994921812177,-1.49924355441912,0.952649463705689));
#6844=CARTESIAN_POINT('Ctrl Pts',(94.1012860649156,-1.51351036467539,0.929788773823545));
#6845=CARTESIAN_POINT('Ctrl Pts',(94.102123556014,-1.52002574889904,0.919098741559542));
#6846=CARTESIAN_POINT('Ctrl Pts',(94.1040112050055,-1.53438316400193,0.894971730459357));
#6847=CARTESIAN_POINT('Ctrl Pts',(94.1050635558847,-1.54216266457929,0.881498940082484));
#6848=CARTESIAN_POINT('Ctrl Pts',(94.107788904356,-1.56172906747557,0.846561279386078));
#6849=CARTESIAN_POINT('Ctrl Pts',(94.1094711183245,-1.5732505281921,0.82495233290072));
#6850=CARTESIAN_POINT('Ctrl Pts',(94.1189551939107,-1.63510497615374,0.702930518248901));
#6851=CARTESIAN_POINT('Ctrl Pts',(94.1270649341482,-1.67626391742539,0.598173178856525));
#6852=CARTESIAN_POINT('Ctrl Pts',(94.1409556276356,-1.72872753119102,0.415473076769958));
#6853=CARTESIAN_POINT('Ctrl Pts',(94.1466655916062,-1.74526506333845,0.339363410515984));
#6854=CARTESIAN_POINT('Ctrl Pts',(94.154131582678,-1.76064256187031,0.236416361928378));
#6855=CARTESIAN_POINT('Ctrl Pts',(94.156000806987,-1.76394835736683,0.210336076608996));
#6856=CARTESIAN_POINT('Ctrl Pts',(94.1591765177528,-1.76863780204441,0.165357040272354));
#6857=CARTESIAN_POINT('Ctrl Pts',(94.1604939932711,-1.77030018113251,0.146492204976438));
#6858=CARTESIAN_POINT('Ctrl Pts',(94.1624129760162,-1.77230472580304,0.118660887134308));
#6859=CARTESIAN_POINT('Ctrl Pts',(94.163026163234,-1.77288111461821,0.109713305489057));
#6860=CARTESIAN_POINT('Ctrl Pts',(94.1641152832622,-1.77379002903949,0.0937165263173397));
#6861=CARTESIAN_POINT('Ctrl Pts',(94.1645925717111,-1.77414832911114,0.0866692890639678));
#6862=CARTESIAN_POINT('Ctrl Pts',(94.1656567692218,-1.77485708536297,0.0708734117247586));
#6863=CARTESIAN_POINT('Ctrl Pts',(94.1662424317102,-1.77518486814393,0.0621241173604022));
#6864=CARTESIAN_POINT('Ctrl Pts',(94.1680103058163,-1.77598353932047,0.0355561584982368));
#6865=CARTESIAN_POINT('Ctrl Pts',(94.1691819780722,-1.77625094277533,0.0177318981764129));
#6866=CARTESIAN_POINT('Ctrl Pts',(94.1767779208922,-1.77624475354874,-0.0989854299933978));
#6867=CARTESIAN_POINT('Ctrl Pts',(94.1828502268093,-1.76798094835211,-0.197716617637565));
#6868=CARTESIAN_POINT('Ctrl Pts',(94.1965998990649,-1.73075146818123,-0.418571406489691));
#6869=CARTESIAN_POINT('Ctrl Pts',(94.2042570865877,-1.69700328735534,-0.539330991453883));
#6870=CARTESIAN_POINT('Ctrl Pts',(94.2138923540971,-1.64203770939722,-0.677751697054265));
#6871=CARTESIAN_POINT('Ctrl Pts',(94.2154520239907,-1.63277075284724,-0.699781953129171));
#6872=CARTESIAN_POINT('Ctrl Pts',(94.2179522869917,-1.61735525944735,-0.734454479384979));
#6873=CARTESIAN_POINT('Ctrl Pts',(94.2188830107744,-1.61149606112767,-0.747222753522626));
#6874=CARTESIAN_POINT('Ctrl Pts',(94.2206566495629,-1.60010728451435,-0.77128387329668));
#6875=CARTESIAN_POINT('Ctrl Pts',(94.2214984711711,-1.59460802119548,-0.78259017362021));
#6876=CARTESIAN_POINT('Ctrl Pts',(94.2234312522828,-1.58177197788939,-0.808283531765959));
#6877=CARTESIAN_POINT('Ctrl Pts',(94.2245248616109,-1.5743581755155,-0.822630635731021));
#6878=CARTESIAN_POINT('Ctrl Pts',(94.2274354808607,-1.55423614550455,-0.860301994549673));
#6879=CARTESIAN_POINT('Ctrl Pts',(94.2292639374394,-1.5411990215746,-0.883444939763982));
#6880=CARTESIAN_POINT('Ctrl Pts',(94.2429048972358,-1.4410785883627,-1.05220938852991));
#6881=CARTESIAN_POINT('Ctrl Pts',(94.255477346546,-1.33405470352637,-1.1849591379934));
#6882=CARTESIAN_POINT('Ctrl Pts',(94.2716191486411,-1.17080256151959,-1.33683724113822));
#6883=CARTESIAN_POINT('Ctrl Pts',(94.2754351091337,-1.13010476343109,-1.37141416390176));
#6884=CARTESIAN_POINT('Ctrl Pts',(94.2800361410189,-1.07775614595733,-1.4119740331767));
#6885=CARTESIAN_POINT('Ctrl Pts',(94.2809220133478,-1.0675192599132,-1.41972942293127));
#6886=CARTESIAN_POINT('Ctrl Pts',(94.2823290258082,-1.05099206811049,-1.43197045773407));
#6887=CARTESIAN_POINT('Ctrl Pts',(94.2828547849573,-1.04475527278908,-1.43652711244484));
#6888=CARTESIAN_POINT('Ctrl Pts',(94.2838662854216,-1.03263391462063,-1.44526237872308));
#6889=CARTESIAN_POINT('Ctrl Pts',(94.2843523422996,-1.02675332044446,-1.4494460204602));
#6890=CARTESIAN_POINT('Ctrl Pts',(94.2854415199169,-1.01345385765933,-1.45878612710112));
#6891=CARTESIAN_POINT('Ctrl Pts',(94.2860432880951,-1.00602070449744,-1.46392214170211));
#6892=CARTESIAN_POINT('Ctrl Pts',(94.288174498974,-0.97940562305954,-1.48201364950666));
#6893=CARTESIAN_POINT('Ctrl Pts',(94.2896846547853,-0.960009133399487,-1.4946512696149));
#6894=CARTESIAN_POINT('Ctrl Pts',(94.2994140133874,-0.831983168734802,-1.57454458702625));
#6895=CARTESIAN_POINT('Ctrl Pts',(94.307103738188,-0.716602985685367,-1.63029889325728));
#6896=CARTESIAN_POINT('Ctrl Pts',(94.3201771133632,-0.516852715869432,-1.70147808438705));
#6897=CARTESIAN_POINT('Ctrl Pts',(94.3254324990652,-0.435574582192307,-1.72407565167617));
#6898=CARTESIAN_POINT('Ctrl Pts',(94.3325286132007,-0.32781886934016,-1.74592648756649));
#6899=CARTESIAN_POINT('Ctrl Pts',(94.3342027055609,-0.302525532545672,-1.75048641927848));
#6900=CARTESIAN_POINT('Ctrl Pts',(94.3368432488757,-0.262897848178668,-1.75674607638215));
#6901=CARTESIAN_POINT('Ctrl Pts',(94.3377977805717,-0.248626005484601,-1.7588226585455));
#6902=CARTESIAN_POINT('Ctrl Pts',(94.3395912693935,-0.221920577800965,-1.76237682160551));
#6903=CARTESIAN_POINT('Ctrl Pts',(94.3404288165683,-0.209493518106686,-1.76389717846503));
#6904=CARTESIAN_POINT('Ctrl Pts',(94.3423171787955,-0.181580944289874,-1.76701294550767));
#6905=CARTESIAN_POINT('Ctrl Pts',(94.3433701941917,-0.166088607430766,-1.76853638256265));
#6906=CARTESIAN_POINT('Ctrl Pts',(94.3460984909525,-0.12614695295972,-1.77193460327382));
#6907=CARTESIAN_POINT('Ctrl Pts',(94.3477830224392,-0.101675936882023,-1.77350703171133));
#6908=CARTESIAN_POINT('Ctrl Pts',(94.3570688884535,0.0321363423118928,-1.77932691128762));
#6909=CARTESIAN_POINT('Ctrl Pts',(94.3649607784222,0.1416419557808,-1.77396938100256));
#6910=CARTESIAN_POINT('Ctrl Pts',(94.3787911940914,0.329085510764859,-1.74732855232778));
#6911=CARTESIAN_POINT('Ctrl Pts',(94.3846621399857,0.407382231093236,-1.7307498218207));
#6912=CARTESIAN_POINT('Ctrl Pts',(94.3923123967429,0.509953960203574,-1.70168213987478));
#6913=CARTESIAN_POINT('Ctrl Pts',(94.394209585663,0.535444238820346,-1.69383433808562));
#6914=CARTESIAN_POINT('Ctrl Pts',(94.3974273775047,0.578909960521693,-1.67937298799806));
#6915=CARTESIAN_POINT('Ctrl Pts',(94.3987593336871,0.596972593103999,-1.67303740912064));
#6916=CARTESIAN_POINT('Ctrl Pts',(94.4006951674767,0.62337693245032,-1.66329381825862));
#6917=CARTESIAN_POINT('Ctrl Pts',(94.4013110078691,0.631800100755204,-1.66011257669175));
#6918=CARTESIAN_POINT('Ctrl Pts',(94.4024028632148,0.646781927089882,-1.65432373099171));
#6919=CARTESIAN_POINT('Ctrl Pts',(94.402880265026,0.653349647123499,-1.65174093362369));
#6920=CARTESIAN_POINT('Ctrl Pts',(94.4039423113655,0.667998671628792,-1.64587906207647));
#6921=CARTESIAN_POINT('Ctrl Pts',(94.4045257381725,0.676071406820056,-1.64257954850405));
#6922=CARTESIAN_POINT('Ctrl Pts',(94.4062797246879,0.700404904422821,-1.63242409693122));
#6923=CARTESIAN_POINT('Ctrl Pts',(94.4074399857254,0.716588657862136,-1.62538494386275));
#6924=CARTESIAN_POINT('Ctrl Pts',(94.4152914120526,0.826455729855655,-1.57563798835702));
#6925=CARTESIAN_POINT('Ctrl Pts',(94.4215989434173,0.916388648129644,-1.52509064329707));
#6926=CARTESIAN_POINT('Ctrl Pts',(94.4330105864461,1.06993965989721,-1.42027149192713));
#6927=CARTESIAN_POINT('Ctrl Pts',(94.4380953728761,1.13507386099655,-1.36877615768248));
#6928=CARTESIAN_POINT('Ctrl Pts',(94.4464479671082,1.2330181228705,-1.27952677679979));
#6929=CARTESIAN_POINT('Ctrl Pts',(94.4496191159074,1.26824979647491,-1.24461409073309));
#6930=CARTESIAN_POINT('Ctrl Pts',(94.4540527565757,1.31447050987135,-1.19480914062528));
#6931=CARTESIAN_POINT('Ctrl Pts',(94.4552599246653,1.32675798727047,-1.18114978113743));
#6932=CARTESIAN_POINT('Ctrl Pts',(94.457331060941,1.34732043012408,-1.15756580730417));
#6933=CARTESIAN_POINT('Ctrl Pts',(94.4581904725254,1.35570317701682,-1.14773682542959));
#6934=CARTESIAN_POINT('Ctrl Pts',(94.4598346093449,1.37145199675288,-1.12885766402803));
#6935=CARTESIAN_POINT('Ctrl Pts',(94.4606184760101,1.3788375838117,-1.11982458948292));
#6936=CARTESIAN_POINT('Ctrl Pts',(94.4624620199673,1.39591755225327,-1.09850947408002));
#6937=CARTESIAN_POINT('Ctrl Pts',(94.4635245125744,1.40553956938392,-1.08617096666951));
#6938=CARTESIAN_POINT('Ctrl Pts',(94.4672702895434,1.43868045069771,-1.0424958885603));
#6939=CARTESIAN_POINT('Ctrl Pts',(94.4699868438229,1.46132293428499,-1.01051174273858));
#6940=CARTESIAN_POINT('Ctrl Pts',(94.4817551455758,1.5535018962888,-0.870718259878636));
#6941=CARTESIAN_POINT('Ctrl Pts',(94.4911663835455,1.61229931143434,-0.756307146531691));
#6942=CARTESIAN_POINT('Ctrl Pts',(94.5056833479908,1.68358186870427,-0.570621332588836));
#6943=CARTESIAN_POINT('Ctrl Pts',(94.5108035080017,1.70494874963744,-0.503198064602601));
#6944=CARTESIAN_POINT('Ctrl Pts',(94.5169846278853,1.72653493725547,-0.41767062453911));
#6945=CARTESIAN_POINT('Ctrl Pts',(94.5182027613506,1.73057485073023,-0.400602526405938));
#6946=CARTESIAN_POINT('Ctrl Pts',(94.5200055535634,1.73623963466528,-0.374982233421327));
#6947=CARTESIAN_POINT('Ctrl Pts',(94.5206000320464,1.73805540695714,-0.366473948232745));
#6948=CARTESIAN_POINT('Ctrl Pts',(94.5216225307759,1.74108889726297,-0.35172983136979));
#6949=CARTESIAN_POINT('Ctrl Pts',(94.522052145146,1.74233574687794,-0.345500464503926));
#6950=CARTESIAN_POINT('Ctrl Pts',(94.5230625809734,1.74520244171498,-0.33076792472615));
#6951=CARTESIAN_POINT('Ctrl Pts',(94.5236417864844,1.74679358884587,-0.322259442687384));
#6952=CARTESIAN_POINT('Ctrl Pts',(94.5253697244878,1.75138057275906,-0.296698336754262));
#6953=CARTESIAN_POINT('Ctrl Pts',(94.5265086023851,1.75418945361529,-0.279612641735894));
#6954=CARTESIAN_POINT('Ctrl Pts',(94.5323275997515,1.76739053090824,-0.191262000545466));
#6955=CARTESIAN_POINT('Ctrl Pts',(94.5368220546751,1.77368748547977,-0.119480554701164));
#6956=CARTESIAN_POINT('Ctrl Pts',(94.5412649413994,1.77561364082571,-0.0475422024484629));
#6957=CARTESIAN_POINT('Origin',(88.3562164250559,0.,0.));
#6958=CARTESIAN_POINT('',(95.4381488292622,1.77561363320029,-0.0475424872431835));
#6959=CARTESIAN_POINT('',(95.2889037169497,1.77561363837295,-0.0475422940546111));
#6960=CARTESIAN_POINT('',(88.3562164250559,1.77561363837197,-0.0475422940912398));
#6961=CARTESIAN_POINT('',(94.877703379636,0.000780936357206753,1.77624982832889));
#6962=CARTESIAN_POINT('Ctrl Pts',(95.4381488292622,1.77561363320029,-0.0475424872432087));
#6963=CARTESIAN_POINT('Ctrl Pts',(95.4324265684948,1.77311855787188,-0.14072839370037));
#6964=CARTESIAN_POINT('Ctrl Pts',(95.4267129126685,1.76329062656178,-0.23361968687051));
#6965=CARTESIAN_POINT('Ctrl Pts',(95.4181001991702,1.73839047815768,-0.367259235214042));
#6966=CARTESIAN_POINT('Ctrl Pts',(95.415363519225,1.72907800086031,-0.408863812839485));
#6967=CARTESIAN_POINT('Ctrl Pts',(95.4114150747514,1.71375977071512,-0.467343100896787));
#6968=CARTESIAN_POINT('Ctrl Pts',(95.4102423138545,1.70898123014907,-0.48452579138951));
#6969=CARTESIAN_POINT('Ctrl Pts',(95.4082203867911,1.70035980048995,-0.513811021492881));
#6970=CARTESIAN_POINT('Ctrl Pts',(95.4073754145735,1.69664431831655,-0.525949864298036));
#6971=CARTESIAN_POINT('Ctrl Pts',(95.4056345502037,1.68876217890978,-0.550748561096265));
#6972=CARTESIAN_POINT('Ctrl Pts',(95.4047382763972,1.68458251974351,-0.563403400592129));
#6973=CARTESIAN_POINT('Ctrl Pts',(95.4024548818364,1.67363046476664,-0.595351317138518));
#6974=CARTESIAN_POINT('Ctrl Pts',(95.4010615152036,1.66666676205364,-0.614576249658972));
#6975=CARTESIAN_POINT('Ctrl Pts',(95.3948711223093,1.63451435575078,-0.698772012019242));
#6976=CARTESIAN_POINT('Ctrl Pts',(95.3899601326701,1.60584997808338,-0.762340582429073));
#6977=CARTESIAN_POINT('Ctrl Pts',(95.379491207287,1.53822869151577,-0.891463177412685));
#6978=CARTESIAN_POINT('Ctrl Pts',(95.3739253392272,1.49863404050213,-0.95652957657421));
#6979=CARTESIAN_POINT('Ctrl Pts',(95.3621965732459,1.406629878176,-1.08791791780787));
#6980=CARTESIAN_POINT('Ctrl Pts',(95.3560482676687,1.35340640349611,-1.153458606964));
#6981=CARTESIAN_POINT('Ctrl Pts',(95.3488597086622,1.28330396284671,-1.22822012633944));
#6982=CARTESIAN_POINT('Ctrl Pts',(95.3475975998636,1.27068138661002,-1.24127459387855));
#6983=CARTESIAN_POINT('Ctrl Pts',(95.3457432337999,1.25163345025343,-1.26037912773783));
#6984=CARTESIAN_POINT('Ctrl Pts',(95.3451403506945,1.24536005250626,-1.26657814105094));
#6985=CARTESIAN_POINT('Ctrl Pts',(95.3440616550468,1.23398505957614,-1.27765203267675));
#6986=CARTESIAN_POINT('Ctrl Pts',(95.3435846090548,1.22890033680306,-1.28254349260462));
#6987=CARTESIAN_POINT('Ctrl Pts',(95.3425111959618,1.21733650987806,-1.29353588048967));
#6988=CARTESIAN_POINT('Ctrl Pts',(95.3419161947615,1.21084055905947,-1.29961855996351));
#6989=CARTESIAN_POINT('Ctrl Pts',(95.340089662298,1.19064337292863,-1.31824790754539));
#6990=CARTESIAN_POINT('Ctrl Pts',(95.3388697170535,1.17679032263864,-1.33062909583091));
#6991=CARTESIAN_POINT('Ctrl Pts',(95.3359971949416,1.14337911723777,-1.3595604051435));
#6992=CARTESIAN_POINT('Ctrl Pts',(95.3343561330884,1.12365180937099,-1.37590953463755));
#6993=CARTESIAN_POINT('Ctrl Pts',(95.3280301460383,1.04544808387427,-1.43791710686284));
#6994=CARTESIAN_POINT('Ctrl Pts',(95.3234763279384,0.984485070895921,-1.48032359163911));
#6995=CARTESIAN_POINT('Ctrl Pts',(95.3117173079998,0.8206856662562,-1.5796566653085));
#6996=CARTESIAN_POINT('Ctrl Pts',(95.3045236388273,0.714552717393068,-1.63041427106398));
#6997=CARTESIAN_POINT('Ctrl Pts',(95.2953923173135,0.581280246780326,-1.67862180093765));
#6998=CARTESIAN_POINT('Ctrl Pts',(95.2938084948094,0.55819782951024,-1.68643795233282));
#6999=CARTESIAN_POINT('Ctrl Pts',(95.2911905369467,0.520160386320609,-1.69845170778107));
#7000=CARTESIAN_POINT('Ctrl Pts',(95.2901656501701,0.505297737654125,-1.70293253006258));
#7001=CARTESIAN_POINT('Ctrl Pts',(95.2883027951456,0.478347950686195,-1.71067354575598));
#7002=CARTESIAN_POINT('Ctrl Pts',(95.2874671097045,0.466281327707187,-1.71400188206105));
#7003=CARTESIAN_POINT('Ctrl Pts',(95.2856573164783,0.440206130705083,-1.72089847978718));
#7004=CARTESIAN_POINT('Ctrl Pts',(95.2846818838194,0.426187240246583,-1.72442379650137));
#7005=CARTESIAN_POINT('Ctrl Pts',(95.2819458810918,0.386973398435257,-1.73377748471631));
#7006=CARTESIAN_POINT('Ctrl Pts',(95.2801733761199,0.361692759244073,-1.73922712799075));
#7007=CARTESIAN_POINT('Ctrl Pts',(95.2724702045185,0.252407513237492,-1.76029960562492));
#7008=CARTESIAN_POINT('Ctrl Pts',(95.2663721128103,0.167465750790382,-1.77039989114934));
#7009=CARTESIAN_POINT('Ctrl Pts',(95.2502794786399,-0.0539681222458069,
-1.78065043690025));
#7010=CARTESIAN_POINT('Ctrl Pts',(95.2401534524402,-0.190348536188963,-1.77127031495713));
#7011=CARTESIAN_POINT('Ctrl Pts',(95.2294194565397,-0.341075672795629,-1.7432790718566));
#7012=CARTESIAN_POINT('Ctrl Pts',(95.2282364246516,-0.357787611082151,-1.73992603745408));
#7013=CARTESIAN_POINT('Ctrl Pts',(95.2264749211728,-0.382858767488722,-1.73451930867552));
#7014=CARTESIAN_POINT('Ctrl Pts',(95.2258872538383,-0.39125502491633,-1.73264467830611));
#7015=CARTESIAN_POINT('Ctrl Pts',(95.2248714263039,-0.405830275616796,-1.72927911123142));
#7016=CARTESIAN_POINT('Ctrl Pts',(95.2244417518351,-0.412015189842297,-1.72781594608054));
#7017=CARTESIAN_POINT('Ctrl Pts',(95.2234246377326,-0.426702631661668,-1.72425798532218));
#7018=CARTESIAN_POINT('Ctrl Pts',(95.2228388937294,-0.435197684934671,-1.72213347883878));
#7019=CARTESIAN_POINT('Ctrl Pts',(95.2210705796401,-0.460941621132549,-1.71549257925249));
#7020=CARTESIAN_POINT('Ctrl Pts',(95.2198985562175,-0.478139116346774,-1.71077906598479));
#7021=CARTESIAN_POINT('Ctrl Pts',(95.2139645498719,-0.565704351290179,-1.68535540345595));
#7022=CARTESIAN_POINT('Ctrl Pts',(95.2093910930455,-0.634818876754864,-1.66055762226319));
#7023=CARTESIAN_POINT('Ctrl Pts',(95.1964484978259,-0.827522332025799,-1.57761952223652));
#7024=CARTESIAN_POINT('Ctrl Pts',(95.1882053118219,-0.946195693212456,-1.50943297655982));
#7025=CARTESIAN_POINT('Ctrl Pts',(95.1773965769074,-1.08192796637439,-1.40909334553449));
#7026=CARTESIAN_POINT('Ctrl Pts',(95.1753002530244,-1.10742900901853,-1.38914108732498));
#7027=CARTESIAN_POINT('Ctrl Pts',(95.1721452626445,-1.14448339748857,-1.35848041529037));
#7028=CARTESIAN_POINT('Ctrl Pts',(95.1711075719997,-1.15646340909492,-1.34829657077988));
#7029=CARTESIAN_POINT('Ctrl Pts',(95.1692310386833,-1.1777459144769,-1.32971262710737));
#7030=CARTESIAN_POINT('Ctrl Pts',(95.1683946341747,-1.1870977852663,-1.32137047951509));
#7031=CARTESIAN_POINT('Ctrl Pts',(95.1665939707368,-1.20693971270538,-1.30329023789246));
#7032=CARTESIAN_POINT('Ctrl Pts',(95.1656285045734,-1.2174018435071,-1.29352295874421));
#7033=CARTESIAN_POINT('Ctrl Pts',(95.1629502542297,-1.24593206827136,-1.2662348676838));
#7034=CARTESIAN_POINT('Ctrl Pts',(95.1612263429251,-1.26374696918884,-1.24845542310128));
#7035=CARTESIAN_POINT('Ctrl Pts',(95.152399111382,-1.3521648206803,-1.15638149238669));
#7036=CARTESIAN_POINT('Ctrl Pts',(95.1450425094611,-1.41660991090255,-1.07646553338749));
#7037=CARTESIAN_POINT('Ctrl Pts',(95.1291959644627,-1.53791981979782,-0.896137958312464));
#7038=CARTESIAN_POINT('Ctrl Pts',(95.1207117506653,-1.59264583236027,-0.794822480818138));
#7039=CARTESIAN_POINT('Ctrl Pts',(95.1111707321944,-1.64521340136675,-0.669897867529944));
#7040=CARTESIAN_POINT('Ctrl Pts',(95.1097315091766,-1.65288882786989,-0.650729516065684));
#7041=CARTESIAN_POINT('Ctrl Pts',(95.107678260501,-1.66349102358425,-0.622853029380883));
#7042=CARTESIAN_POINT('Ctrl Pts',(95.1070500096327,-1.6666869153076,-0.614249963288017));
#7043=CARTESIAN_POINT('Ctrl Pts',(95.1059441935771,-1.67222882539966,-0.59896986072012));
#7044=CARTESIAN_POINT('Ctrl Pts',(95.105465104336,-1.67460181617816,-0.592303049118153));
#7045=CARTESIAN_POINT('Ctrl Pts',(95.1044188508592,-1.67972256448044,-0.577639726472503));
#7046=CARTESIAN_POINT('Ctrl Pts',(95.1038526772859,-1.68245314035489,-0.569637590997079));
#7047=CARTESIAN_POINT('Ctrl Pts',(95.1022038725421,-1.69028172873587,-0.546147945574999));
#7048=CARTESIAN_POINT('Ctrl Pts',(95.1011298050568,-1.69522391876263,-0.530608907419999));
#7049=CARTESIAN_POINT('Ctrl Pts',(95.0937191628379,-1.72814746321451,-0.421933043930216));
#7050=CARTESIAN_POINT('Ctrl Pts',(95.0877332835159,-1.74865625657932,-0.326691590553083));
#7051=CARTESIAN_POINT('Ctrl Pts',(95.0741434425496,-1.7773404623019,-0.10726553706973));
#7052=CARTESIAN_POINT('Ctrl Pts',(95.0665668041369,-1.7804916892154,0.0170396937590265));
#7053=CARTESIAN_POINT('Ctrl Pts',(95.0570192499336,-1.76876145063724,0.164709809400757));
#7054=CARTESIAN_POINT('Ctrl Pts',(95.0554504160024,-1.7663606362436,0.188723087792008));
#7055=CARTESIAN_POINT('Ctrl Pts',(95.0528520911397,-1.76162105744444,0.228022254037951));
#7056=CARTESIAN_POINT('Ctrl Pts',(95.0518316076365,-1.7595705262178,0.24334016606842));
#7057=CARTESIAN_POINT('Ctrl Pts',(95.0499733997698,-1.75549850328728,0.271008562644912));
#7058=CARTESIAN_POINT('Ctrl Pts',(95.0491379047138,-1.75354584950283,0.283368269175139));
#7059=CARTESIAN_POINT('Ctrl Pts',(95.0473246935836,-1.74904765090326,0.310011037129568));
#7060=CARTESIAN_POINT('Ctrl Pts',(95.0463456100258,-1.74645738825423,0.324285518475907));
#7061=CARTESIAN_POINT('Ctrl Pts',(95.0435883381943,-1.73871557095237,0.364162329949569));
#7062=CARTESIAN_POINT('Ctrl Pts',(95.0417979111599,-1.73317400411456,0.389684210974678));
#7063=CARTESIAN_POINT('Ctrl Pts',(95.0339428759946,-1.70666171999534,0.499998706699272));
#7064=CARTESIAN_POINT('Ctrl Pts',(95.0277028843341,-1.68001816416497,0.583290644364273));
#7065=CARTESIAN_POINT('Ctrl Pts',(95.0117066079709,-1.59767699582025,0.787491680522473));
#7066=CARTESIAN_POINT('Ctrl Pts',(95.0018426481373,-1.53432409620246,0.904747022041888));
#7067=CARTESIAN_POINT('Ctrl Pts',(94.9912894596819,-1.44838529901362,1.02837604788023));
#7068=CARTESIAN_POINT('Ctrl Pts',(94.990059980716,-1.43806675187335,1.04275660960599));
#7069=CARTESIAN_POINT('Ctrl Pts',(94.9882438534851,-1.42233915655661,1.06399793819069));
#7070=CARTESIAN_POINT('Ctrl Pts',(94.9876471802424,-1.4170919966957,1.07097645620828));
#7071=CARTESIAN_POINT('Ctrl Pts',(94.9865746236708,-1.4075107247553,1.08352546255025));
#7072=CARTESIAN_POINT('Ctrl Pts',(94.9860975810893,-1.40319468065931,1.0891090672964));
#7073=CARTESIAN_POINT('Ctrl Pts',(94.9850179752984,-1.39330297239163,1.10174941113212));
#7074=CARTESIAN_POINT('Ctrl Pts',(94.9844168555606,-1.38770686901168,1.10878969702321));
#7075=CARTESIAN_POINT('Ctrl Pts',(94.9825511889574,-1.37007076034943,1.13063446331415));
#7076=CARTESIAN_POINT('Ctrl Pts',(94.9812989542025,-1.35784506876156,1.14528818177321));
#7077=CARTESIAN_POINT('Ctrl Pts',(94.9783350577334,-1.32804496998012,1.17985843991184));
#7078=CARTESIAN_POINT('Ctrl Pts',(94.9766359253695,-1.31025504095858,1.19958378468223));
#7079=CARTESIAN_POINT('Ctrl Pts',(94.969934113325,-1.2375955262759,1.27660230793023));
#7080=CARTESIAN_POINT('Ctrl Pts',(94.965078843049,-1.17935497475244,1.33059372196977));
#7081=CARTESIAN_POINT('Ctrl Pts',(94.9534424500203,-1.03201372128253,1.44988470252031));
#7082=CARTESIAN_POINT('Ctrl Pts',(94.9466620620704,-0.940068495925,1.5111206372368));
#7083=CARTESIAN_POINT('Ctrl Pts',(94.9379825175937,-0.821473912657809,1.57506995714734));
#7084=CARTESIAN_POINT('Ctrl Pts',(94.936389783875,-0.79966367959214,1.5862542876717));
#7085=CARTESIAN_POINT('Ctrl Pts',(94.9337601581515,-0.763636625949545,1.60379718300328));
#7086=CARTESIAN_POINT('Ctrl Pts',(94.9327326594191,-0.749554841324666,1.61042659404732));
#7087=CARTESIAN_POINT('Ctrl Pts',(94.9308670335171,-0.723991625699923,1.62205330861708));
#7088=CARTESIAN_POINT('Ctrl Pts',(94.9300312208673,-0.712540902645496,1.62711593266471));
#7089=CARTESIAN_POINT('Ctrl Pts',(94.9282233853606,-0.687783848757428,1.6377501399672));
#7090=CARTESIAN_POINT('Ctrl Pts',(94.9272500623634,-0.674461325399115,1.64328148614164));
#7091=CARTESIAN_POINT('Ctrl Pts',(94.9245263212566,-0.637207859443691,1.65821932763941));
#7092=CARTESIAN_POINT('Ctrl Pts',(94.9227641418537,-0.613138655464252,1.6672690434214));
#7093=CARTESIAN_POINT('Ctrl Pts',(94.915147377191,-0.509293203912989,1.70376089238181));
#7094=CARTESIAN_POINT('Ctrl Pts',(94.9091298018082,-0.427823702698999,1.72601971223949));
#7095=CARTESIAN_POINT('Ctrl Pts',(94.8945833023764,-0.23118032335632,1.76496585089555));
#7096=CARTESIAN_POINT('Ctrl Pts',(94.8859871579056,-0.11533655142876,1.77630087991323));
#7097=CARTESIAN_POINT('Ctrl Pts',(94.877703379636,0.000780936357206753,
1.77624982832889));
#7098=CARTESIAN_POINT('Ctrl Pts',(94.8777032004959,0.000783447447140647,
1.7762498272231));
#7099=CARTESIAN_POINT('Ctrl Pts',(94.875703743125,0.0288107681561156,1.77623746526111));
#7100=CARTESIAN_POINT('Ctrl Pts',(94.8737250593201,0.0568359658703815,1.77556174085671));
#7101=CARTESIAN_POINT('Ctrl Pts',(94.8710993587005,0.0945567494872465,1.77375810203675));
#7102=CARTESIAN_POINT('Ctrl Pts',(94.870426291296,0.10427439127338,1.77321336702983));
#7103=CARTESIAN_POINT('Ctrl Pts',(94.8692666882143,0.121108806098811,1.77213082045504));
#7104=CARTESIAN_POINT('Ctrl Pts',(94.8687783067807,0.128227617541035,1.77162994730939));
#7105=CARTESIAN_POINT('Ctrl Pts',(94.8678277550067,0.142143366094598,1.77056652966511));
#7106=CARTESIAN_POINT('Ctrl Pts',(94.8673654011623,0.148940475069296,1.77000771579285));
#7107=CARTESIAN_POINT('Ctrl Pts',(94.8663652577609,0.163708107271948,1.76870794332323));
#7108=CARTESIAN_POINT('Ctrl Pts',(94.8658282854875,0.171677059085947,1.76795224111264));
#7109=CARTESIAN_POINT('Ctrl Pts',(94.8643505085288,0.193710050634295,1.76571245320849));
#7110=CARTESIAN_POINT('Ctrl Pts',(94.8634157709342,0.207762242826518,1.76411420625861));
#7111=CARTESIAN_POINT('Ctrl Pts',(94.8586703207988,0.279595805800326,1.75507383565549));
#7112=CARTESIAN_POINT('Ctrl Pts',(94.8549859291996,0.337010668443167,1.74495937527194));
#7113=CARTESIAN_POINT('Ctrl Pts',(94.84421111473,0.505731147393458,1.70659583264059));
#7114=CARTESIAN_POINT('Ctrl Pts',(94.8372918228665,0.614903438240659,1.67036769308429));
#7115=CARTESIAN_POINT('Ctrl Pts',(94.8260972895909,0.778940256290118,1.59765394461424));
#7116=CARTESIAN_POINT('Ctrl Pts',(94.8219990014537,0.836579443054001,1.5682408995006));
#7117=CARTESIAN_POINT('Ctrl Pts',(94.8164896090179,0.90978577643737,1.52569800683077));
#7118=CARTESIAN_POINT('Ctrl Pts',(94.8151776146235,0.926916987703905,1.51535125028546));
#7119=CARTESIAN_POINT('Ctrl Pts',(94.8129802009186,0.955083961327412,1.4976828596905));
#7120=CARTESIAN_POINT('Ctrl Pts',(94.8121007696611,0.96621948330322,1.49052313479004));
#7121=CARTESIAN_POINT('Ctrl Pts',(94.8103651199301,0.987921238072749,1.47622433141034));
#7122=CARTESIAN_POINT('Ctrl Pts',(94.809509289856,0.998492694527664,1.46909461014019));
#7123=CARTESIAN_POINT('Ctrl Pts',(94.8076161708394,1.02158779773059,1.45315411566405));
#7124=CARTESIAN_POINT('Ctrl Pts',(94.806577045216,1.0340760059473,1.44429404921418));
#7125=CARTESIAN_POINT('Ctrl Pts',(94.802998916464,1.07642500819074,1.41341769880217));
#7126=CARTESIAN_POINT('Ctrl Pts',(94.8004304361012,1.10570805280832,1.39062925916566));
#7127=CARTESIAN_POINT('Ctrl Pts',(94.7886790829253,1.23464563109819,1.28364008405797));
#7128=CARTESIAN_POINT('Ctrl Pts',(94.7791128656865,1.32554221729754,1.18954188861098));
#7129=CARTESIAN_POINT('Ctrl Pts',(94.764381381594,1.44896646288052,1.02988187557092));
#7130=CARTESIAN_POINT('Ctrl Pts',(94.7592062256311,1.48918810011262,0.970814732654317));
#7131=CARTESIAN_POINT('Ctrl Pts',(94.7529674294456,1.53476904779362,0.894348050746785));
#7132=CARTESIAN_POINT('Ctrl Pts',(94.7517435890676,1.5435647888861,0.87908035308186));
#7133=CARTESIAN_POINT('Ctrl Pts',(94.7499340809887,1.55637005957131,0.856067904802723));
#7134=CARTESIAN_POINT('Ctrl Pts',(94.7493384906121,1.56055181923945,0.848420914107435));
#7135=CARTESIAN_POINT('Ctrl Pts',(94.748314815403,1.56768464611979,0.835146264809442));
#7136=CARTESIAN_POINT('Ctrl Pts',(94.7478851241269,1.57066197592887,0.829533238696455));
#7137=CARTESIAN_POINT('Ctrl Pts',(94.7468755652192,1.57761741955346,0.81624874218973));
#7138=CARTESIAN_POINT('Ctrl Pts',(94.7462973013654,1.58156974962538,0.808564076914775));
#7139=CARTESIAN_POINT('Ctrl Pts',(94.7446107894178,1.59299710025869,0.785941038893312));
#7140=CARTESIAN_POINT('Ctrl Pts',(94.7435115015725,1.60031790311815,0.770925247035328));
#7141=CARTESIAN_POINT('Ctrl Pts',(94.7350147950301,1.65577918666664,0.652972084690577));
#7142=CARTESIAN_POINT('Ctrl Pts',(94.7280933940864,1.69415909453756,0.545719051896373));
#7143=CARTESIAN_POINT('Ctrl Pts',(94.714985142822,1.74651125830193,0.33872130499129));
#7144=CARTESIAN_POINT('Ctrl Pts',(94.7088334531639,1.76278532830978,0.240039130214569));
#7145=CARTESIAN_POINT('Ctrl Pts',(94.7004472569654,1.77312909141282,0.109696185932724));
#7146=CARTESIAN_POINT('Ctrl Pts',(94.6984427640807,1.77476974884387,0.0788173959524371));
#7147=CARTESIAN_POINT('Ctrl Pts',(94.6953990870834,1.77602050079453,0.0324658310265796));
#7148=CARTESIAN_POINT('Ctrl Pts',(94.6943787048488,1.77623572074468,0.0170143637278835));
#7149=CARTESIAN_POINT('Ctrl Pts',(94.6925206034954,1.77626031955146,-0.0109503858670986));
#7150=CARTESIAN_POINT('Ctrl Pts',(94.6916851124531,1.77613910528311,-0.0234627078840527));
#7151=CARTESIAN_POINT('Ctrl Pts',(94.6905865700469,1.7758075807968,-0.0398293953416206));
#7152=CARTESIAN_POINT('Ctrl Pts',(94.6903272973286,1.77571689021663,-0.0436860354302763));
#7153=CARTESIAN_POINT('Ctrl Pts',(94.6900676319115,1.77561363837053,-0.0475422941449777));
#7154=CARTESIAN_POINT('Ctrl Pts',(94.5412649413994,1.77561364082571,-0.0475422024484629));
#7155=CARTESIAN_POINT('Ctrl Pts',(94.5434435753088,1.77655815902118,-0.0122661886016114));
#7156=CARTESIAN_POINT('Ctrl Pts',(94.5456095196027,1.77645169809017,0.0230475721265798));
#7157=CARTESIAN_POINT('Ctrl Pts',(94.5527068568138,1.77265305223877,0.13861651702398));
#7158=CARTESIAN_POINT('Ctrl Pts',(94.5576379267421,1.76457463705705,0.218606026469179));
#7159=CARTESIAN_POINT('Ctrl Pts',(94.5657720795508,1.74295772007151,0.345729776074744));
#7160=CARTESIAN_POINT('Ctrl Pts',(94.5688853545426,1.73283620115693,0.393330323373668));
#7161=CARTESIAN_POINT('Ctrl Pts',(94.5732511454832,1.71624881524957,0.458134480433476));
#7162=CARTESIAN_POINT('Ctrl Pts',(94.5744506205441,1.71145078563001,0.475745063641914));
#7163=CARTESIAN_POINT('Ctrl Pts',(94.5765125960301,1.70280106133474,0.505666802134386));
#7164=CARTESIAN_POINT('Ctrl Pts',(94.5773706405815,1.69908501689463,0.518015887451013));
#7165=CARTESIAN_POINT('Ctrl Pts',(94.5790149050942,1.69174492462631,0.541479281216473));
#7166=CARTESIAN_POINT('Ctrl Pts',(94.5798002946744,1.68814496518447,0.552600458880006));
#7167=CARTESIAN_POINT('Ctrl Pts',(94.5816516457733,1.67944135714042,0.578609072298788));
#7168=CARTESIAN_POINT('Ctrl Pts',(94.5827204840958,1.67424916718845,0.593465608874096));
#7169=CARTESIAN_POINT('Ctrl Pts',(94.5865124798222,1.6552470192782,0.645601887097282));
#7170=CARTESIAN_POINT('Ctrl Pts',(94.5892699932211,1.64038456002125,0.682482638773605));
#7171=CARTESIAN_POINT('Ctrl Pts',(94.6010434200455,1.57262699252526,0.83559018769827));
#7172=CARTESIAN_POINT('Ctrl Pts',(94.6104123635189,1.50852229504532,0.946424030956493));
#7173=CARTESIAN_POINT('Ctrl Pts',(94.6235364062967,1.40228318021252,1.09150726091316));
#7174=CARTESIAN_POINT('Ctrl Pts',(94.6273238652075,1.36961682322703,1.1322264051728));
#7175=CARTESIAN_POINT('Ctrl Pts',(94.6325255392511,1.32144277379587,1.18713453414243));
#7176=CARTESIAN_POINT('Ctrl Pts',(94.6339994282064,1.30740627510489,1.20257570203997));
#7177=CARTESIAN_POINT('Ctrl Pts',(94.6365701166745,1.2821876951167,1.22935435805946));
#7178=CARTESIAN_POINT('Ctrl Pts',(94.6376733263133,1.27111931151023,1.24079537525619));
#7179=CARTESIAN_POINT('Ctrl Pts',(94.6393404165796,1.25399393429083,1.25802759555352));
#7180=CARTESIAN_POINT('Ctrl Pts',(94.6399121397877,1.2480476146365,1.26392696672909));
#7181=CARTESIAN_POINT('Ctrl Pts',(94.6409614888597,1.23699376369573,1.27473946701458));
#7182=CARTESIAN_POINT('Ctrl Pts',(94.6414399693347,1.2318984362493,1.27966422375792));
#7183=CARTESIAN_POINT('Ctrl Pts',(94.642540041456,1.22005809701332,1.29097193205022));
#7184=CARTESIAN_POINT('Ctrl Pts',(94.6431599607674,1.21329233301522,1.2973326534049));
#7185=CARTESIAN_POINT('Ctrl Pts',(94.6451883213664,1.19085916085582,1.31809382820894));
#7186=CARTESIAN_POINT('Ctrl Pts',(94.6465809711968,1.17498219071284,1.33226642609027));
#7187=CARTESIAN_POINT('Ctrl Pts',(94.6564081460819,1.05988575192336,1.4313488550651));
#7188=CARTESIAN_POINT('Ctrl Pts',(94.6642639264257,0.951812226279923,1.50538350037581));
#7189=CARTESIAN_POINT('Ctrl Pts',(94.6775415222494,0.761795526559401,1.60683530918759));
#7190=CARTESIAN_POINT('Ctrl Pts',(94.6828276127812,0.684250487879997,1.64135646493972));
#7191=CARTESIAN_POINT('Ctrl Pts',(94.689961140598,0.580311036885342,1.67897804010269));
#7192=CARTESIAN_POINT('Ctrl Pts',(94.6916397317116,0.555892524882368,1.68722006550244));
#7193=CARTESIAN_POINT('Ctrl Pts',(94.6942857863076,0.517528764756738,1.69924584836991));
#7194=CARTESIAN_POINT('Ctrl Pts',(94.6952412464933,0.503701418451321,1.70339582478594));
#7195=CARTESIAN_POINT('Ctrl Pts',(94.6970355597131,0.477792442568631,1.71082879107591));
#7196=CARTESIAN_POINT('Ctrl Pts',(94.6978729907988,0.465723642820633,1.71415350689919));
#7197=CARTESIAN_POINT('Ctrl Pts',(94.6997598697513,0.438589493482345,1.72132072206722));
#7198=CARTESIAN_POINT('Ctrl Pts',(94.700811502654,0.423506969534449,1.72509350236888));
#7199=CARTESIAN_POINT('Ctrl Pts',(94.7035336668793,0.384580720599134,1.73428936766983));
#7200=CARTESIAN_POINT('Ctrl Pts',(94.7052133781941,0.360671714155253,1.73941879735231));
#7201=CARTESIAN_POINT('Ctrl Pts',(94.7147798457699,0.225174148445743,1.76557474098718));
#7202=CARTESIAN_POINT('Ctrl Pts',(94.7229820693175,0.111894069949005,1.77635281458003));
#7203=CARTESIAN_POINT('Ctrl Pts',(94.7389518392365,-0.106611507095988,1.77615348264895));
#7204=CARTESIAN_POINT('Ctrl Pts',(94.746668989523,-0.211395605660704,1.76674918023911));
#7205=CARTESIAN_POINT('Ctrl Pts',(94.7552634553239,-0.332087971155573,1.74501927664064));
#7206=CARTESIAN_POINT('Ctrl Pts',(94.7564877600887,-0.349387274758901,1.7416381046173));
#7207=CARTESIAN_POINT('Ctrl Pts',(94.7582978003044,-0.375162915506406,1.73620068701901));
#7208=CARTESIAN_POINT('Ctrl Pts',(94.7588934669821,-0.383678520159998,1.73433873277692));
#7209=CARTESIAN_POINT('Ctrl Pts',(94.7599650217581,-0.399063629366382,1.73085588382814));
#7210=CARTESIAN_POINT('Ctrl Pts',(94.7604420572206,-0.40593748644609,1.72925667033796));
#7211=CARTESIAN_POINT('Ctrl Pts',(94.7615226513983,-0.421563592899136,1.72552292000326));
#7212=CARTESIAN_POINT('Ctrl Pts',(94.7621247540477,-0.430309341109339,1.72336272735353));
#7213=CARTESIAN_POINT('Ctrl Pts',(94.7639968300216,-0.457608564069119,1.71639906499678));
#7214=CARTESIAN_POINT('Ctrl Pts',(94.7652543697975,-0.476101663996281,1.71136162943988));
#7215=CARTESIAN_POINT('Ctrl Pts',(94.768233372978,-0.520168319588268,1.6985884189086));
#7216=CARTESIAN_POINT('Ctrl Pts',(94.7699421344828,-0.545656460626269,1.6905729428433));
#7217=CARTESIAN_POINT('Ctrl Pts',(94.7767083201064,-0.646906959570245,1.65620312853243));
#7218=CARTESIAN_POINT('Ctrl Pts',(94.7816154567932,-0.721030108955061,1.62530449470644));
#7219=CARTESIAN_POINT('Ctrl Pts',(94.7932330923504,-0.890396752790922,1.54082733611291));
#7220=CARTESIAN_POINT('Ctrl Pts',(94.7999437074288,-0.983278404503882,1.48327855500644));
#7221=CARTESIAN_POINT('Ctrl Pts',(94.8085468900542,-1.08986526937704,1.4028040514305));
#7222=CARTESIAN_POINT('Ctrl Pts',(94.8101405954477,-1.10912869219456,1.38762349454655));
#7223=CARTESIAN_POINT('Ctrl Pts',(94.81277147336,-1.14009642816649,1.36216245883458));
#7224=CARTESIAN_POINT('Ctrl Pts',(94.8137992365312,-1.15199107933619,1.35211795238197));
#7225=CARTESIAN_POINT('Ctrl Pts',(94.8156651144676,-1.17321025229277,1.3337160531245));
#7226=CARTESIAN_POINT('Ctrl Pts',(94.8165009112172,-1.1825814461775,1.32541386585446));
#7227=CARTESIAN_POINT('Ctrl Pts',(94.8183084541581,-1.20255644791122,1.30733699456991));
#7228=CARTESIAN_POINT('Ctrl Pts',(94.8192814975433,-1.21313048100066,1.2975309023102));
#7229=CARTESIAN_POINT('Ctrl Pts',(94.8220037216389,-1.24220958108485,1.26989748804954));
#7230=CARTESIAN_POINT('Ctrl Pts',(94.8237646428141,-1.26044833168126,1.2517963716943));
#7231=CARTESIAN_POINT('Ctrl Pts',(94.8313711261778,-1.33677242489935,1.17268863172378));
#7232=CARTESIAN_POINT('Ctrl Pts',(94.8373791575991,-1.39086350194149,1.10799562186814));
#7233=CARTESIAN_POINT('Ctrl Pts',(94.8527475346567,-1.51483987673093,0.936270947243736));
#7234=CARTESIAN_POINT('Ctrl Pts',(94.8622145351851,-1.57816049923806,0.825078083531655));
#7235=CARTESIAN_POINT('Ctrl Pts',(94.8728821540885,-1.63831439447118,0.686682823221446));
#7236=CARTESIAN_POINT('Ctrl Pts',(94.8745129533067,-1.64718470709737,0.665124065403948));
#7237=CARTESIAN_POINT('Ctrl Pts',(94.8767467116256,-1.6589098163154,0.634952236839583));
#7238=CARTESIAN_POINT('Ctrl Pts',(94.8773684449951,-1.66212650423166,0.626483530869504));
#7239=CARTESIAN_POINT('Ctrl Pts',(94.8784792478827,-1.66779130427911,0.611218780106395));
#7240=CARTESIAN_POINT('Ctrl Pts',(94.8789696540811,-1.6702630139578,0.604431719198467));
#7241=CARTESIAN_POINT('Ctrl Pts',(94.879978543617,-1.67528848118149,0.590366039129934));
#7242=CARTESIAN_POINT('Ctrl Pts',(94.8804966876522,-1.67783634156848,0.583085561431611));
#7243=CARTESIAN_POINT('Ctrl Pts',(94.8818671320378,-1.68448380497436,0.563686118329876));
#7244=CARTESIAN_POINT('Ctrl Pts',(94.8827147370964,-1.68850013209264,0.551538807908548));
#7245=CARTESIAN_POINT('Ctrl Pts',(94.88701432694,-1.70835896923778,0.489225139120706));
#7246=CARTESIAN_POINT('Ctrl Pts',(94.8903609323159,-1.72209994049072,0.438411365064706));
#7247=CARTESIAN_POINT('Ctrl Pts',(94.9036857741804,-1.76849888945552,0.230598326965006));
#7248=CARTESIAN_POINT('Ctrl Pts',(94.9132243868449,-1.78209093110531,0.0701343464581758));
#7249=CARTESIAN_POINT('Ctrl Pts',(94.9257522701928,-1.77214205701239,-0.126007263530086));
#7250=CARTESIAN_POINT('Ctrl Pts',(94.9280811972879,-1.76921778330781,-0.161967437868291));
#7251=CARTESIAN_POINT('Ctrl Pts',(94.9315050673402,-1.7633968524475,-0.21391131945955));
#7252=CARTESIAN_POINT('Ctrl Pts',(94.9325728633011,-1.7613725929161,-0.229984938382008));
#7253=CARTESIAN_POINT('Ctrl Pts',(94.9344843034777,-1.75738192392362,-0.258518663800589));
#7254=CARTESIAN_POINT('Ctrl Pts',(94.9353251626267,-1.75550209055475,-0.270989892894573));
#7255=CARTESIAN_POINT('Ctrl Pts',(94.9371000712876,-1.75127545796363,-0.297137798532043));
#7256=CARTESIAN_POINT('Ctrl Pts',(94.9380349504658,-1.74890088713878,-0.310809055377591));
#7257=CARTESIAN_POINT('Ctrl Pts',(94.9405382663113,-1.74215142742212,-0.347138235356091));
#7258=CARTESIAN_POINT('Ctrl Pts',(94.9421155343129,-1.73749488418756,-0.369740436532594));
#7259=CARTESIAN_POINT('Ctrl Pts',(94.9519300734694,-1.70606385045465,-0.508559700312585));
#7260=CARTESIAN_POINT('Ctrl Pts',(94.9605275135835,-1.66808572455898,-0.621906143790832));
#7261=CARTESIAN_POINT('Ctrl Pts',(94.9770561318937,-1.57505260064922,-0.828080069001339));
#7262=CARTESIAN_POINT('Ctrl Pts',(94.9849239146365,-1.52233277957435,-0.921419479417054));
#7263=CARTESIAN_POINT('Ctrl Pts',(94.9936347948144,-1.45166570501596,-1.02373434210288));
#7264=CARTESIAN_POINT('Ctrl Pts',(94.9948400755776,-1.44159244751381,-1.03787118367639));
#7265=CARTESIAN_POINT('Ctrl Pts',(94.9966277598574,-1.42618238120057,-1.0588403779074));
#7266=CARTESIAN_POINT('Ctrl Pts',(94.9972197526479,-1.42100048785081,-1.06578457100507));
#7267=CARTESIAN_POINT('Ctrl Pts',(94.9982397279222,-1.41193145563184,-1.07775413845314));
#7268=CARTESIAN_POINT('Ctrl Pts',(94.9986692760981,-1.40806797023224,-1.08279684743485));
#7269=CARTESIAN_POINT('Ctrl Pts',(94.9996819527362,-1.3988548921779,-1.09468926274514));
#7270=CARTESIAN_POINT('Ctrl Pts',(95.0002634368031,-1.3934819848297,-1.10152056595514));
#7271=CARTESIAN_POINT('Ctrl Pts',(95.0020054073728,-1.37714420552958,-1.12198212815959));
#7272=CARTESIAN_POINT('Ctrl Pts',(95.003155801247,-1.36602755333219,-1.13549057186784));
#7273=CARTESIAN_POINT('Ctrl Pts',(95.0088694110335,-1.30927830354811,-1.20240970909248));
#7274=CARTESIAN_POINT('Ctrl Pts',(95.0132593202433,-1.26070049116031,-1.25324985570592));
#7275=CARTESIAN_POINT('Ctrl Pts',(95.0254475237736,-1.11616753847906,-1.38757954873728));
#7276=CARTESIAN_POINT('Ctrl Pts',(95.033121635433,-1.01409527658672,-1.46383623508831));
#7277=CARTESIAN_POINT('Ctrl Pts',(95.0437489087865,-0.87001800323518,-1.54911679932686));
#7278=CARTESIAN_POINT('Ctrl Pts',(95.0463448859884,-0.834584722617513,-1.56849040086878));
#7279=CARTESIAN_POINT('Ctrl Pts',(95.0500169875117,-0.784389482339222,-1.5937526773605));
#7280=CARTESIAN_POINT('Ctrl Pts',(95.0510572721582,-0.770160762154759,-1.60067699127721));
#7281=CARTESIAN_POINT('Ctrl Pts',(95.0528788410603,-0.745245153024947,-1.61239289303791));
#7282=CARTESIAN_POINT('Ctrl Pts',(95.053657105732,-0.734599715248548,-1.61727067208922));
#7283=CARTESIAN_POINT('Ctrl Pts',(95.0552988179213,-0.712148975299129,-1.62729029012666));
#7284=CARTESIAN_POINT('Ctrl Pts',(95.0561629772106,-0.700334476037257,-1.63240970895281));
#7285=CARTESIAN_POINT('Ctrl Pts',(95.0582553817403,-0.671742383278715,-1.64443161667852));
#7286=CARTESIAN_POINT('Ctrl Pts',(95.0594878620959,-0.654912963943813,-1.65120626767301));
#7287=CARTESIAN_POINT('Ctrl Pts',(95.0639998206859,-0.593367912671106,-1.67489221659939));
#7288=CARTESIAN_POINT('Ctrl Pts',(95.0673296359578,-0.54808159029031,-1.69025301140629));
#7289=CARTESIAN_POINT('Ctrl Pts',(95.0762308901081,-0.427409082755968,-1.72582469587156));
#7290=CARTESIAN_POINT('Ctrl Pts',(95.0818829023581,-0.351219060787104,-1.74292638970081));
#7291=CARTESIAN_POINT('Ctrl Pts',(95.0956950600995,-0.164373503566121,-1.7721152392473));
#7292=CARTESIAN_POINT('Ctrl Pts',(95.1038795333791,-0.0532130267965422,
-1.77892754413776));
#7293=CARTESIAN_POINT('Ctrl Pts',(95.1128575780263,0.0749361269299614,-1.77475082035718));
#7294=CARTESIAN_POINT('Ctrl Pts',(95.1140434384957,0.0920021229135656,-1.77394801522403));
#7295=CARTESIAN_POINT('Ctrl Pts',(95.1158082619779,0.117648740364889,-1.77237043935367));
#7296=CARTESIAN_POINT('Ctrl Pts',(95.116396470495,0.126239103854104,-1.77177930252482));
#7297=CARTESIAN_POINT('Ctrl Pts',(95.117412798325,0.141161734065333,-1.77064333324257));
#7298=CARTESIAN_POINT('Ctrl Pts',(95.1178424384907,0.147495688575089,-1.77012696540166));
#7299=CARTESIAN_POINT('Ctrl Pts',(95.1188589253252,0.162541516793648,-1.76881905046448));
#7300=CARTESIAN_POINT('Ctrl Pts',(95.1194440832824,0.171250480059544,-1.76799713210154));
#7301=CARTESIAN_POINT('Ctrl Pts',(95.121208817696,0.19764592661323,-1.76530915916036));
#7302=CARTESIAN_POINT('Ctrl Pts',(95.1223779094459,0.215311383646996,-1.7632417324343));
#7303=CARTESIAN_POINT('Ctrl Pts',(95.1282817616309,0.305238573714238,-1.75134562496465));
#7304=CARTESIAN_POINT('Ctrl Pts',(95.1328301145104,0.376884303222874,-1.73733780508449));
#7305=CARTESIAN_POINT('Ctrl Pts',(95.1456670787031,0.578221806123637,-1.68492652615933));
#7306=CARTESIAN_POINT('Ctrl Pts',(95.1538297663241,0.70465086388769,-1.63608765895191));
#7307=CARTESIAN_POINT('Ctrl Pts',(95.1645894126931,0.853676717625577,-1.55801106405439));
#7308=CARTESIAN_POINT('Ctrl Pts',(95.166733008376,0.882595328091569,-1.54181311344165));
#7309=CARTESIAN_POINT('Ctrl Pts',(95.1699593513328,0.924850222355441,-1.51656679347856));
#7310=CARTESIAN_POINT('Ctrl Pts',(95.1710201463706,0.938544807379738,-1.50813009687887));
#7311=CARTESIAN_POINT('Ctrl Pts',(95.1729218754768,0.962730480610808,-1.49277325131496));
#7312=CARTESIAN_POINT('Ctrl Pts',(95.1737600907851,0.973266381157452,-1.48592546768418));
#7313=CARTESIAN_POINT('Ctrl Pts',(95.1755468440813,0.995456352245029,-1.4711659004954));
#7314=CARTESIAN_POINT('Ctrl Pts',(95.1764963968491,1.00709068531736,-1.4632261573744));
#7315=CARTESIAN_POINT('Ctrl Pts',(95.1790833471573,1.0383520440042,-1.44134267528383));
#7316=CARTESIAN_POINT('Ctrl Pts',(95.1807306461126,1.05779138225488,-1.42713733299095));
#7317=CARTESIAN_POINT('Ctrl Pts',(95.1844334598677,1.10043622175063,-1.39462450664985));
#7318=CARTESIAN_POINT('Ctrl Pts',(95.1864960078317,1.12348517127626,-1.37612437235903));
#7319=CARTESIAN_POINT('Ctrl Pts',(95.1932713126165,1.1969259695372,-1.31410228372658));
#7320=CARTESIAN_POINT('Ctrl Pts',(95.1980634804437,1.24533103709929,-1.26832396499313));
#7321=CARTESIAN_POINT('Ctrl Pts',(95.2102229721831,1.36010362625739,-1.14686153849779));
#7322=CARTESIAN_POINT('Ctrl Pts',(95.2176419270819,1.42282901537072,-1.06805032390844));
#7323=CARTESIAN_POINT('Ctrl Pts',(95.2275189585559,1.49919773066883,-0.953340656220574));
#7324=CARTESIAN_POINT('Ctrl Pts',(95.2301563675644,1.51886618126048,-0.921682275466301));
#7325=CARTESIAN_POINT('Ctrl Pts',(95.2335640464393,1.54347746721085,-0.879137448296057));
#7326=CARTESIAN_POINT('Ctrl Pts',(95.2343825668173,1.54932606729685,-0.868788870410129));
#7327=CARTESIAN_POINT('Ctrl Pts',(95.235708401415,1.55870284709006,-0.851801615550708));
#7328=CARTESIAN_POINT('Ctrl Pts',(95.2362194709419,1.56229343614907,-0.845198072931727));
#7329=CARTESIAN_POINT('Ctrl Pts',(95.2372323281931,1.56936369097838,-0.831995980060367));
#7330=CARTESIAN_POINT('Ctrl Pts',(95.2377341406856,1.57284391557293,-0.825397920617801));
#7331=CARTESIAN_POINT('Ctrl Pts',(95.2390112958784,1.58163952950383,-0.808464914562898));
#7332=CARTESIAN_POINT('Ctrl Pts',(95.2397830249633,1.58689535073497,-0.798099168716691));
#7333=CARTESIAN_POINT('Ctrl Pts',(95.2430663341115,1.6089794240698,-0.753463235619792));
#7334=CARTESIAN_POINT('Ctrl Pts',(95.2455233506389,1.6248034083339,-0.718704390900775));
#7335=CARTESIAN_POINT('Ctrl Pts',(95.252726840723,1.66854897756847,-0.613766708088673));
#7336=CARTESIAN_POINT('Ctrl Pts',(95.2573583214528,1.69313063363843,-0.542287244323431));
#7337=CARTESIAN_POINT('Ctrl Pts',(95.2690837777104,1.74361902570175,-0.358050339677971));
#7338=CARTESIAN_POINT('Ctrl Pts',(95.2761699902226,1.76320571122477,-0.24394500650331));
#7339=CARTESIAN_POINT('Ctrl Pts',(95.2851838045764,1.77334698114173,-0.104405221888593));
#7340=CARTESIAN_POINT('Ctrl Pts',(95.2867703384516,1.77461426961264,-0.0800254182370063));
#7341=CARTESIAN_POINT('Ctrl Pts',(95.2885492368346,1.77546315899532,-0.0529330183040422));
#7342=CARTESIAN_POINT('Ctrl Pts',(95.2887263841943,1.77554146783561,-0.050237725415923));
#7343=CARTESIAN_POINT('Ctrl Pts',(95.2889037169497,1.77561363837295,-0.0475422940546111));
#7344=CARTESIAN_POINT('Origin',(88.3562164250559,0.,0.));
#7345=CARTESIAN_POINT('',(96.1869838792616,1.77561363799551,-0.0475423081512957));
#7346=CARTESIAN_POINT('',(96.0403469459233,1.77561363956144,-0.0475422496666916));
#7347=CARTESIAN_POINT('',(88.3562164250559,1.77561363837197,-0.0475422940912398));
#7348=CARTESIAN_POINT('Ctrl Pts',(96.1869838792616,1.77561363799551,-0.0475423081512957));
#7349=CARTESIAN_POINT('Ctrl Pts',(96.1859735229126,1.77523265929886,-0.0617711286663794));
#7350=CARTESIAN_POINT('Ctrl Pts',(96.1849689213711,1.77468059977411,-0.0759971484777021));
#7351=CARTESIAN_POINT('Ctrl Pts',(96.1827450801735,1.77306860399109,-0.107694088353561));
#7352=CARTESIAN_POINT('Ctrl Pts',(96.1815296802457,1.77192153164029,-0.125157638420296));
#7353=CARTESIAN_POINT('Ctrl Pts',(96.1797300866637,1.76981866583316,-0.151266345408754));
#7354=CARTESIAN_POINT('Ctrl Pts',(96.1791361226274,1.7690572234074,-0.159925499836574));
#7355=CARTESIAN_POINT('Ctrl Pts',(96.178114144888,1.76762928885563,-0.174903170570591));
#7356=CARTESIAN_POINT('Ctrl Pts',(96.1776845429653,1.76699243626332,-0.181224047609109));
#7357=CARTESIAN_POINT('Ctrl Pts',(96.1766736081873,1.76540694149744,-0.196156692790316));
#7358=CARTESIAN_POINT('Ctrl Pts',(96.1760938975564,1.76442919360367,-0.204765099153601));
#7359=CARTESIAN_POINT('Ctrl Pts',(96.1743989621701,1.76136919100643,-0.230054824132373));
#7360=CARTESIAN_POINT('Ctrl Pts',(96.1732928321384,1.75911300867986,-0.246714657494879));
#7361=CARTESIAN_POINT('Ctrl Pts',(96.1648781519479,1.73997177847874,-0.374396708413501));
#7362=CARTESIAN_POINT('Ctrl Pts',(96.1580333729285,1.71282649337141,-0.483639263159261));
#7363=CARTESIAN_POINT('Ctrl Pts',(96.1492357523241,1.66525661782863,-0.618825052799923));
#7364=CARTESIAN_POINT('Ctrl Pts',(96.1473323413611,1.65420923574938,-0.647777594852745));
#7365=CARTESIAN_POINT('Ctrl Pts',(96.1418649586059,1.62049403668184,-0.72964049025782));
#7366=CARTESIAN_POINT('Ctrl Pts',(96.1382788973759,1.59600569984257,-0.781755238240675));
#7367=CARTESIAN_POINT('Ctrl Pts',(96.1321223854516,1.55062686273318,-0.867272910072371));
#7368=CARTESIAN_POINT('Ctrl Pts',(96.1295932580675,1.53107714644833,-0.901336995056063));
#7369=CARTESIAN_POINT('Ctrl Pts',(96.1259182703506,1.50152186348764,-0.949095257506187));
#7370=CARTESIAN_POINT('Ctrl Pts',(96.1248052096535,1.49242344868247,-0.963338949442147));
#7371=CARTESIAN_POINT('Ctrl Pts',(96.1228444575935,1.47615074196743,-0.988030162692928));
#7372=CARTESIAN_POINT('Ctrl Pts',(96.1220001248121,1.46906521437369,-0.998534925310201));
#7373=CARTESIAN_POINT('Ctrl Pts',(96.1202349680317,1.45409463545272,-1.02022552892517));
#7374=CARTESIAN_POINT('Ctrl Pts',(96.1193134924493,1.44619150802514,-1.03139781005262));
#7375=CARTESIAN_POINT('Ctrl Pts',(96.11688640093,1.42515167703041,-1.06042352245404));
#7376=CARTESIAN_POINT('Ctrl Pts',(96.1153728865511,1.41180885801858,-1.07812384274513));
#7377=CARTESIAN_POINT('Ctrl Pts',(96.1075088181668,1.34137448488336,-1.16801048254654));
#7378=CARTESIAN_POINT('Ctrl Pts',(96.1009522451003,1.279074957092,-1.23591929776607));
#7379=CARTESIAN_POINT('Ctrl Pts',(96.0884369810071,1.15302173583489,-1.35353945693111));
#7380=CARTESIAN_POINT('Ctrl Pts',(96.0825238555979,1.0905834334467,-1.40433456704));
#7381=CARTESIAN_POINT('Ctrl Pts',(96.0736144279593,0.990465257690351,-1.47506688072342));
#7382=CARTESIAN_POINT('Ctrl Pts',(96.0705713942124,0.955151946663038,-1.49817519867346));
#7383=CARTESIAN_POINT('Ctrl Pts',(96.065696906075,0.896328910181318,-1.53374161948242));
#7384=CARTESIAN_POINT('Ctrl Pts',(96.0638352040829,0.873303959652029,-1.54696775906898));
#7385=CARTESIAN_POINT('Ctrl Pts',(96.0612966699708,0.841018065885381,-1.56456290114178));
#7386=CARTESIAN_POINT('Ctrl Pts',(96.06059553862,0.832004126180052,-1.56937490913489));
#7387=CARTESIAN_POINT('Ctrl Pts',(96.0594091779596,0.816577961339088,-1.57743975422904));
#7388=CARTESIAN_POINT('Ctrl Pts',(96.058921577677,0.810186688795131,-1.58073188182259));
#7389=CARTESIAN_POINT('Ctrl Pts',(96.057899317769,0.796676547085477,-1.5875874495117));
#7390=CARTESIAN_POINT('Ctrl Pts',(96.0573651942251,0.789553484107672,-1.59114195861709));
#7391=CARTESIAN_POINT('Ctrl Pts',(96.0559037556126,0.769895264690334,-1.60078716882656));
#7392=CARTESIAN_POINT('Ctrl Pts',(96.0549822893982,0.757311645158543,-1.60677857231766));
#7393=CARTESIAN_POINT('Ctrl Pts',(96.0493879199421,0.679856412915963,-1.64254498428812));
#7394=CARTESIAN_POINT('Ctrl Pts',(96.0449097627957,0.613301598140134,-1.66853898768166));
#7395=CARTESIAN_POINT('Ctrl Pts',(96.0336579349796,0.440269671422942,-1.72436047511622));
#7396=CARTESIAN_POINT('Ctrl Pts',(96.026980188727,0.332254115690725,-1.74838885050254));
#7397=CARTESIAN_POINT('Ctrl Pts',(96.0176297866786,0.184213907851702,-1.76709780608814));
#7398=CARTESIAN_POINT('Ctrl Pts',(96.0151732957584,0.145574176402628,-1.77069965970032));
#7399=CARTESIAN_POINT('Ctrl Pts',(96.0107803220572,0.0773083520507664,-1.77481360072315));
#7400=CARTESIAN_POINT('Ctrl Pts',(96.0088594725822,0.0477290226381277,-1.77585519562847));
#7401=CARTESIAN_POINT('Ctrl Pts',(96.0059174789471,0.00293958411527544,
-1.77631260239359));
#7402=CARTESIAN_POINT('Ctrl Pts',(96.0049132563282,-0.0122605817015053,
-1.77627271461423));
#7403=CARTESIAN_POINT('Ctrl Pts',(96.0031527711524,-0.0387417759068703,
-1.77586330888285));
#7404=CARTESIAN_POINT('Ctrl Pts',(96.0023992932645,-0.0500234251042128,
-1.77558133124439));
#7405=CARTESIAN_POINT('Ctrl Pts',(96.0006864631264,-0.0755461067529935,
-1.77469997516593));
#7406=CARTESIAN_POINT('Ctrl Pts',(95.9997251551623,-0.0897840005021764,
-1.7740366480704));
#7407=CARTESIAN_POINT('Ctrl Pts',(95.9971146343462,-0.128205631444982,-1.77178292225054));
#7408=CARTESIAN_POINT('Ctrl Pts',(95.9954554498375,-0.152366565774769,-1.76986884709633));
#7409=CARTESIAN_POINT('Ctrl Pts',(95.9837558204365,-0.320864485336603,-1.75304444636456));
#7410=CARTESIAN_POINT('Ctrl Pts',(95.9731652489588,-0.462913996172033,-1.72099202256592));
#7411=CARTESIAN_POINT('Ctrl Pts',(95.9583642421423,-0.653576288649097,-1.6526366980808));
#7412=CARTESIAN_POINT('Ctrl Pts',(95.9541785644385,-0.706729636315566,-1.63061461010219));
#7413=CARTESIAN_POINT('Ctrl Pts',(95.9477571517117,-0.78811212986688,-1.59216825771662));
#7414=CARTESIAN_POINT('Ctrl Pts',(95.9454662527019,-0.817116154218881,-1.57747963451054));
#7415=CARTESIAN_POINT('Ctrl Pts',(95.942456226926,-0.855376199582139,-1.55676479462481));
#7416=CARTESIAN_POINT('Ctrl Pts',(95.9417000568971,-0.865001097227207,-1.55143745795666));
#7417=CARTESIAN_POINT('Ctrl Pts',(95.9404489894633,-0.880957475654667,-1.54241101544268));
#7418=CARTESIAN_POINT('Ctrl Pts',(95.9399510829823,-0.887316556175685,-1.53876156400432));
#7419=CARTESIAN_POINT('Ctrl Pts',(95.9390010148878,-0.89947043673321,-1.53168609926305));
#7420=CARTESIAN_POINT('Ctrl Pts',(95.9385484399101,-0.905268613795681,-1.52826637531556));
#7421=CARTESIAN_POINT('Ctrl Pts',(95.9373165547804,-0.921069314523666,-1.5188257556306));
#7422=CARTESIAN_POINT('Ctrl Pts',(95.9365413793302,-0.931032353349821,-1.51273895080924));
#7423=CARTESIAN_POINT('Ctrl Pts',(95.9334386523684,-0.970953549639229,-1.48780572817097));
#7424=CARTESIAN_POINT('Ctrl Pts',(95.9311570894005,-1.00040743980018,-1.46816280606409));
#7425=CARTESIAN_POINT('Ctrl Pts',(95.9224343439896,-1.11235341354032,-1.38857101751339));
#7426=CARTESIAN_POINT('Ctrl Pts',(95.9162469296047,-1.19021507280611,-1.32244126257992));
#7427=CARTESIAN_POINT('Ctrl Pts',(95.9041191872546,-1.32897063129383,-1.18235524528025));
#7428=CARTESIAN_POINT('Ctrl Pts',(95.8982083459856,-1.39041099511642,-1.10945080248137));
#7429=CARTESIAN_POINT('Ctrl Pts',(95.8904394394053,-1.46029157284766,-1.01155444584408));
#7430=CARTESIAN_POINT('Ctrl Pts',(95.8888036478111,-1.47443693559598,-0.990822635789977));
#7431=CARTESIAN_POINT('Ctrl Pts',(95.8862100196735,-1.49594418338592,-0.957820177632319));
#7432=CARTESIAN_POINT('Ctrl Pts',(95.8852633972785,-1.50360544961536,-0.945747917912847));
#7433=CARTESIAN_POINT('Ctrl Pts',(95.8834767546907,-1.51770755677366,-0.922921950612268));
#7434=CARTESIAN_POINT('Ctrl Pts',(95.882638040963,-1.5241819614242,-0.912189941496587));
#7435=CARTESIAN_POINT('Ctrl Pts',(95.8807362186176,-1.53853226994615,-0.887823420743908));
#7436=CARTESIAN_POINT('Ctrl Pts',(95.8796707723648,-1.54634145138274,-0.874151050978877));
#7437=CARTESIAN_POINT('Ctrl Pts',(95.8763862728584,-1.56970698315513,-0.831949460391712));
#7438=CARTESIAN_POINT('Ctrl Pts',(95.8741463061002,-1.58466234777351,-0.803097080071995));
#7439=CARTESIAN_POINT('Ctrl Pts',(95.8623725387151,-1.65820214162449,-0.651160231893396));
#7440=CARTESIAN_POINT('Ctrl Pts',(95.8523915150334,-1.70325821519041,-0.52205705929633));
#7441=CARTESIAN_POINT('Ctrl Pts',(95.837086880413,-1.74916676237373,-0.317574761520012));
#7442=CARTESIAN_POINT('Ctrl Pts',(95.8317673133952,-1.76078359686751,-0.24511480604364));
#7443=CARTESIAN_POINT('Ctrl Pts',(95.8253774571049,-1.76961674749343,-0.154396793821098));
#7444=CARTESIAN_POINT('Ctrl Pts',(95.8241389160994,-1.7710771374349,-0.136629560796241));
#7445=CARTESIAN_POINT('Ctrl Pts',(95.8223121579015,-1.7728556718333,-0.110106707688259));
#7446=CARTESIAN_POINT('Ctrl Pts',(95.8217137503719,-1.77337688413802,-0.101366440216693));
#7447=CARTESIAN_POINT('Ctrl Pts',(95.8206871184338,-1.7741648731016,-0.0862754849370903));
#7448=CARTESIAN_POINT('Ctrl Pts',(95.8202572560546,-1.77446221688727,-0.0799268456068247));
#7449=CARTESIAN_POINT('Ctrl Pts',(95.8192500022411,-1.77508186827587,-0.0649803284838484));
#7450=CARTESIAN_POINT('Ctrl Pts',(95.818674183327,-1.77537579439365,-0.0563815445028544));
#7451=CARTESIAN_POINT('Ctrl Pts',(95.8169670492244,-1.77606581132273,-0.0307394339663348));
#7452=CARTESIAN_POINT('Ctrl Pts',(95.8158452404988,-1.7762790520397,-0.0136916335852668));
#7453=CARTESIAN_POINT('Ctrl Pts',(95.8058569137283,-1.77598936320795,0.139571542453031));
#7454=CARTESIAN_POINT('Ctrl Pts',(95.79767224834,-1.76006424360702,0.275323520346167));
#7455=CARTESIAN_POINT('Ctrl Pts',(95.7840093761035,-1.70914764296041,0.491100796826062));
#7456=CARTESIAN_POINT('Ctrl Pts',(95.7786838601724,-1.68354994538585,0.572732785812526));
#7457=CARTESIAN_POINT('Ctrl Pts',(95.7715022726718,-1.64268433392603,0.676255153691229));
#7458=CARTESIAN_POINT('Ctrl Pts',(95.7698179094051,-1.63266496171668,0.700098468406816));
#7459=CARTESIAN_POINT('Ctrl Pts',(95.7671647622894,-1.61623931686642,0.73691484913708));
#7460=CARTESIAN_POINT('Ctrl Pts',(95.7662080897019,-1.61018879729897,0.750043359101764));
#7461=CARTESIAN_POINT('Ctrl Pts',(95.7644126597065,-1.59860136190742,0.774399397664015));
#7462=CARTESIAN_POINT('Ctrl Pts',(95.7635753395328,-1.59310465495523,0.785645139936856));
#7463=CARTESIAN_POINT('Ctrl Pts',(95.7616902449042,-1.58052611485467,0.810704766537366));
#7464=CARTESIAN_POINT('Ctrl Pts',(95.7606403044382,-1.573381201103,0.824485650277882));
#7465=CARTESIAN_POINT('Ctrl Pts',(95.7579257106127,-1.55455862039561,0.859654176813744));
#7466=CARTESIAN_POINT('Ctrl Pts',(95.7562519639852,-1.54262012868615,0.880897748940143));
#7467=CARTESIAN_POINT('Ctrl Pts',(95.7464256325662,-1.47063969579265,1.00302817252497));
#7468=CARTESIAN_POINT('Ctrl Pts',(95.7379332657299,-1.40116005939237,1.09799289654791));
#7469=CARTESIAN_POINT('Ctrl Pts',(95.7239298355492,-1.27333678860947,1.24063663272306));
#7470=CARTESIAN_POINT('Ctrl Pts',(95.7184924732507,-1.22042260659681,1.29272403303986));
#7471=CARTESIAN_POINT('Ctrl Pts',(95.711340178858,-1.14506138807853,1.35814380783864));
#7472=CARTESIAN_POINT('Ctrl Pts',(95.7095199438121,-1.12535606069443,1.37451593606286));
#7473=CARTESIAN_POINT('Ctrl Pts',(95.7064181605257,-1.09076089563072,1.4020163373249));
#7474=CARTESIAN_POINT('Ctrl Pts',(95.7051262489749,-1.07603810565433,1.41334751736624));
#7475=CARTESIAN_POINT('Ctrl Pts',(95.7032370542885,-1.05400337544441,1.42976226444971));
#7476=CARTESIAN_POINT('Ctrl Pts',(95.7026285833451,-1.04682715687904,1.43502479437198));
#7477=CARTESIAN_POINT('Ctrl Pts',(95.7015442622734,-1.03389064340781,1.44436282875775));
#7478=CARTESIAN_POINT('Ctrl Pts',(95.7010671123727,-1.02814529912166,1.44845817757642));
#7479=CARTESIAN_POINT('Ctrl Pts',(95.6999988261138,-1.01516339262973,1.4575956674066));
#7480=CARTESIAN_POINT('Ctrl Pts',(95.6994089897435,-1.00791351863893,1.46261826550269));
#7481=CARTESIAN_POINT('Ctrl Pts',(95.6976150817076,-0.985623541884869,1.47781596155627));
#7482=CARTESIAN_POINT('Ctrl Pts',(95.6964220076421,-0.97046404878879,1.4878149667598));
#7483=CARTESIAN_POINT('Ctrl Pts',(95.6897493717963,-0.883968819634331,1.54298142280817));
#7484=CARTESIAN_POINT('Ctrl Pts',(95.6845216377863,-0.809629171838312,1.5832550317039));
#7485=CARTESIAN_POINT('Ctrl Pts',(95.674701715773,-0.664181357209329,1.64911624553048));
#7486=CARTESIAN_POINT('Ctrl Pts',(95.6701121242482,-0.593763265790631,1.67575837658732));
#7487=CARTESIAN_POINT('Ctrl Pts',(95.6610608490213,-0.454649415661084,1.71851783307174));
#7488=CARTESIAN_POINT('Ctrl Pts',(95.6566184865083,-0.386267692939748,1.73516720257875));
#7489=CARTESIAN_POINT('Ctrl Pts',(95.6507140889594,-0.296914735555921,1.75137828699455));
#7490=CARTESIAN_POINT('Ctrl Pts',(95.6493710514397,-0.276684058899716,1.75468804602519));
#7491=CARTESIAN_POINT('Ctrl Pts',(95.6471358948983,-0.243203130442738,1.75957216344348));
#7492=CARTESIAN_POINT('Ctrl Pts',(95.6462502105929,-0.229984009911182,1.76134871610423));
#7493=CARTESIAN_POINT('Ctrl Pts',(95.6445127132718,-0.204152872671202,1.76452448612535));
#7494=CARTESIAN_POINT('Ctrl Pts',(95.6436614005759,-0.191543373337164,1.76593776198209));
#7495=CARTESIAN_POINT('Ctrl Pts',(95.6416056159878,-0.161212996013897,1.76900853237707));
#7496=CARTESIAN_POINT('Ctrl Pts',(95.6403971044501,-0.143480542504504,1.77053497884845));
#7497=CARTESIAN_POINT('Ctrl Pts',(95.6362851695688,-0.0834944389435133,
1.77479166539372));
#7498=CARTESIAN_POINT('Ctrl Pts',(95.6333437714287,-0.0411698961341193,
1.77627736966851));
#7499=CARTESIAN_POINT('Ctrl Pts',(95.625696656016,0.0673416476502539,1.77620623763022));
#7500=CARTESIAN_POINT('Ctrl Pts',(95.620934451418,0.133458634067817,1.77246460935006));
#7501=CARTESIAN_POINT('Ctrl Pts',(95.6088790732658,0.298121982068145,1.75388030200898));
#7502=CARTESIAN_POINT('Ctrl Pts',(95.6015348677352,0.395923435846904,1.73442151491004));
#7503=CARTESIAN_POINT('Ctrl Pts',(95.5916229010142,0.528674836413008,1.69618898666391));
#7504=CARTESIAN_POINT('Ctrl Pts',(95.5888877211877,0.565413989852701,1.68429857096844));
#7505=CARTESIAN_POINT('Ctrl Pts',(95.585375856801,0.613056594757594,1.66714437314468));
#7506=CARTESIAN_POINT('Ctrl Pts',(95.5845473109883,0.624332631081921,1.66295445971391));
#7507=CARTESIAN_POINT('Ctrl Pts',(95.583209379177,0.642613237956164,1.65594965222455));
#7508=CARTESIAN_POINT('Ctrl Pts',(95.5826961133567,0.649643743825658,1.65320417245067));
#7509=CARTESIAN_POINT('Ctrl Pts',(95.5816828576435,0.663562120940664,1.64766641273418));
#7510=CARTESIAN_POINT('Ctrl Pts',(95.5811828068971,0.670450358746701,1.64487556267026));
#7511=CARTESIAN_POINT('Ctrl Pts',(95.5799160052794,0.687943434773452,1.63765989372201));
#7512=CARTESIAN_POINT('Ctrl Pts',(95.5791527521862,0.698523442117217,1.63317516363878));
#7513=CARTESIAN_POINT('Ctrl Pts',(95.5759615185912,0.742888354547811,1.61385943417819));
#7514=CARTESIAN_POINT('Ctrl Pts',(95.5735843700897,0.77625284968718,1.59807926411387));
#7515=CARTESIAN_POINT('Ctrl Pts',(95.5667343953338,0.87237081149124,1.54889763119721));
#7516=CARTESIAN_POINT('Ctrl Pts',(95.5623638008931,0.93364212962893,1.51275525330887));
#7517=CARTESIAN_POINT('Ctrl Pts',(95.5505174098619,1.0936450894637,1.40493933661967));
#7518=CARTESIAN_POINT('Ctrl Pts',(95.5430649397026,1.18741679163067,1.32663164266866));
#7519=CARTESIAN_POINT('Ctrl Pts',(95.5336515557619,1.28933674948063,1.22199093018612));
#7520=CARTESIAN_POINT('Ctrl Pts',(95.5320765746302,1.30588424271542,1.20429121942383));
#7521=CARTESIAN_POINT('Ctrl Pts',(95.5294701966113,1.33240388976126,1.17473556481106));
#7522=CARTESIAN_POINT('Ctrl Pts',(95.5284479057122,1.34259245340436,1.1630774915711));
#7523=CARTESIAN_POINT('Ctrl Pts',(95.526587794063,1.36073848934771,1.14175804873563));
#7524=CARTESIAN_POINT('Ctrl Pts',(95.5257522245866,1.36874879658817,1.13214283387398));
#7525=CARTESIAN_POINT('Ctrl Pts',(95.5239404345869,1.38581048569498,1.1112169897048));
#7526=CARTESIAN_POINT('Ctrl Pts',(95.5229628642119,1.39482638505668,1.09987873619199));
#7527=CARTESIAN_POINT('Ctrl Pts',(95.5202144155178,1.41963978328277,1.06787799251214));
#7528=CARTESIAN_POINT('Ctrl Pts',(95.5184314249069,1.43512305180507,1.04697766091598));
#7529=CARTESIAN_POINT('Ctrl Pts',(95.5106396972869,1.5001219296749,0.955085942278702));
#7530=CARTESIAN_POINT('Ctrl Pts',(95.50445891989,1.54486432781,0.880877595526095));
#7531=CARTESIAN_POINT('Ctrl Pts',(95.4884237680268,1.64476288353193,0.683990516287231));
#7532=CARTESIAN_POINT('Ctrl Pts',(95.4784520596189,1.69174164374578,0.557764116329369));
#7533=CARTESIAN_POINT('Ctrl Pts',(95.467823869387,1.72824699052075,0.410524503161078));
#7534=CARTESIAN_POINT('Ctrl Pts',(95.4666130685231,1.73219337590142,0.393540586785368));
#7535=CARTESIAN_POINT('Ctrl Pts',(95.4648188803351,1.73772898071901,0.368018188507811));
#7536=CARTESIAN_POINT('Ctrl Pts',(95.4642258051852,1.7395065866799,0.359522239049211));
#7537=CARTESIAN_POINT('Ctrl Pts',(95.4632047610572,1.74247720472665,0.344786318748178));
#7538=CARTESIAN_POINT('Ctrl Pts',(95.4627752137472,1.74369909258552,0.338552643482281));
#7539=CARTESIAN_POINT('Ctrl Pts',(95.4617635255774,1.74651068104241,0.323789702221176));
#7540=CARTESIAN_POINT('Ctrl Pts',(95.4611830171794,1.74807136764266,0.315255185170671));
#7541=CARTESIAN_POINT('Ctrl Pts',(95.459447129513,1.75257655302122,0.28955614842903));
#7542=CARTESIAN_POINT('Ctrl Pts',(95.4583017389889,1.75533132109198,0.272358855766785));
#7543=CARTESIAN_POINT('Ctrl Pts',(95.4526382998094,1.76782129619378,0.18630121235037));
#7544=CARTESIAN_POINT('Ctrl Pts',(95.448290181176,1.7737605212833,0.116944363334072));
#7545=CARTESIAN_POINT('Ctrl Pts',(95.4420352323939,1.77646257458917,0.0157485988176179));
#7546=CARTESIAN_POINT('Ctrl Pts',(95.440091044771,1.77646049673819,-0.0159138844807851));
#7547=CARTESIAN_POINT('Ctrl Pts',(95.4381488292622,1.77561363320029,-0.0475424872432087));
#7548=CARTESIAN_POINT('',(95.4827176862982,0.000795599009507856,1.77624982182187));
#7549=CARTESIAN_POINT('Ctrl Pts',(95.2889037169497,1.77561363837295,-0.0475422940546111));
#7550=CARTESIAN_POINT('Ctrl Pts',(95.2897480647306,1.77595726937842,-0.0347083340615077));
#7551=CARTESIAN_POINT('Ctrl Pts',(95.2905966195916,1.77616174091978,-0.0218712350535019));
#7552=CARTESIAN_POINT('Ctrl Pts',(95.2922811358752,1.77629068903477,0.00348412783102648));
#7553=CARTESIAN_POINT('Ctrl Pts',(95.2931168284974,1.77622202669782,0.0160015365959801));
#7554=CARTESIAN_POINT('Ctrl Pts',(95.2949259376486,1.77578916117662,0.0429602236757479));
#7555=CARTESIAN_POINT('Ctrl Pts',(95.2959006712007,1.77538107689167,0.0573997916003285));
#7556=CARTESIAN_POINT('Ctrl Pts',(95.2986327151757,1.77375307414394,0.0976236153042587));
#7557=CARTESIAN_POINT('Ctrl Pts',(95.3004019048997,1.77214719495702,0.123387744904151));
#7558=CARTESIAN_POINT('Ctrl Pts',(95.3080774447668,1.76283725475589,0.233902057791716));
#7559=CARTESIAN_POINT('Ctrl Pts',(95.314149796804,1.74961077559695,0.318062621267385));
#7560=CARTESIAN_POINT('Ctrl Pts',(95.3299315432877,1.70053412170142,0.529870729698813));
#7561=CARTESIAN_POINT('Ctrl Pts',(95.3397599148447,1.65634522364526,0.655058599028514));
#7562=CARTESIAN_POINT('Ctrl Pts',(95.3504614292562,1.59001249145733,0.792034045329869));
#7563=CARTESIAN_POINT('Ctrl Pts',(95.3518432033154,1.58106662819951,0.809744435590271));
#7564=CARTESIAN_POINT('Ctrl Pts',(95.3538368460025,1.56757243095919,0.835382618322914));
#7565=CARTESIAN_POINT('Ctrl Pts',(95.3544616728043,1.56325703680746,0.843430430661255));
#7566=CARTESIAN_POINT('Ctrl Pts',(95.3555629191811,1.55549423342535,0.857643067696634));
#7567=CARTESIAN_POINT('Ctrl Pts',(95.3560408308539,1.5520718858252,0.863821051232642));
#7568=CARTESIAN_POINT('Ctrl Pts',(95.3570961488097,1.5443952464054,0.877485913187523));
#7569=CARTESIAN_POINT('Ctrl Pts',(95.357672430337,1.5401232699767,0.884962443250514));
#7570=CARTESIAN_POINT('Ctrl Pts',(95.3593824543972,1.52721352768129,0.907179576641817));
#7571=CARTESIAN_POINT('Ctrl Pts',(95.3605066421698,1.51841700988203,0.921827413578864));
#7572=CARTESIAN_POINT('Ctrl Pts',(95.3659622732344,1.47428508204245,0.992968987845695));
#7573=CARTESIAN_POINT('Ctrl Pts',(95.370137405077,1.43599784132198,1.04757625256597));
#7574=CARTESIAN_POINT('Ctrl Pts',(95.3837818726047,1.29944008789964,1.22073713171126));
#7575=CARTESIAN_POINT('Ctrl Pts',(95.3930287272009,1.18886389514128,1.32866254075628));
#7576=CARTESIAN_POINT('Ctrl Pts',(95.4044901795697,1.04664671799196,1.43532777786403));
#7577=CARTESIAN_POINT('Ctrl Pts',(95.4060442387585,1.02724172054587,1.44927897340892));
#7578=CARTESIAN_POINT('Ctrl Pts',(95.4086231816926,0.994890756746498,1.47156147415257));
#7579=CARTESIAN_POINT('Ctrl Pts',(95.4096392927381,0.982107110040264,1.48012377509035));
#7580=CARTESIAN_POINT('Ctrl Pts',(95.4114928873141,0.958731703293867,1.49534412498387));
#7581=CARTESIAN_POINT('Ctrl Pts',(95.4123281944281,0.948177662924896,1.50205846649818));
#7582=CARTESIAN_POINT('Ctrl Pts',(95.4141448510894,0.925187221370135,1.51634582557369));
#7583=CARTESIAN_POINT('Ctrl Pts',(95.415127611126,0.912726934048016,1.52387846600492));
#7584=CARTESIAN_POINT('Ctrl Pts',(95.4179064750809,0.877439345272682,1.54462288368058));
#7585=CARTESIAN_POINT('Ctrl Pts',(95.4197151303545,0.854409181742743,1.55748016918706));
#7586=CARTESIAN_POINT('Ctrl Pts',(95.4277273623025,0.752165852048041,1.61161039089555));
#7587=CARTESIAN_POINT('Ctrl Pts',(95.4341147851219,0.67020116420117,1.64738209155729));
#7588=CARTESIAN_POINT('Ctrl Pts',(95.4471648173014,0.500755366929287,1.70658837214136));
#7589=CARTESIAN_POINT('Ctrl Pts',(95.4538102893005,0.413463621563228,1.72981145364995));
#7590=CARTESIAN_POINT('Ctrl Pts',(95.4638215852848,0.277182520490236,1.75515764743322));
#7591=CARTESIAN_POINT('Ctrl Pts',(95.4672749072743,0.229232446356009,1.7620618286026));
#7592=CARTESIAN_POINT('Ctrl Pts',(95.471534092154,0.168252665807003,1.76831013935905));
#7593=CARTESIAN_POINT('Ctrl Pts',(95.4724219609697,0.155434993547325,1.76948288930693));
#7594=CARTESIAN_POINT('Ctrl Pts',(95.4738313781281,0.134900281988557,1.77113684621543));
#7595=CARTESIAN_POINT('Ctrl Pts',(95.4743575720501,0.127191162104832,1.7717071507879));
#7596=CARTESIAN_POINT('Ctrl Pts',(95.4753331304126,0.112814139200693,1.77267640771399));
#7597=CARTESIAN_POINT('Ctrl Pts',(95.4757831760955,0.106147377196289,1.77308810060367));
#7598=CARTESIAN_POINT('Ctrl Pts',(95.4767200729813,0.0922005598590766,1.77387041588002));
#7599=CARTESIAN_POINT('Ctrl Pts',(95.4772065323742,0.0849201555293663,1.77423385362435));
#7600=CARTESIAN_POINT('Ctrl Pts',(95.4784450815012,0.0662910261649312,1.77504888740892));
#7601=CARTESIAN_POINT('Ctrl Pts',(95.4791938865745,0.0549396407647299,1.77543648280939));
#7602=CARTESIAN_POINT('Ctrl Pts',(95.4808718906935,0.0293249217568935,1.77606519674254));
#7603=CARTESIAN_POINT('Ctrl Pts',(95.4817981529735,0.0150607598054103,1.77624343232211));
#7604=CARTESIAN_POINT('Ctrl Pts',(95.4827176862982,0.000795599009507856,
1.77624982182187));
#7605=CARTESIAN_POINT('Ctrl Pts',(95.4827175421507,0.000797835238689031,
1.77624982081883));
#7606=CARTESIAN_POINT('Ctrl Pts',(95.4904658484486,-0.119405257906508,1.77630381224638));
#7607=CARTESIAN_POINT('Ctrl Pts',(95.4977298043407,-0.239323346943683,1.76415612306193));
#7608=CARTESIAN_POINT('Ctrl Pts',(95.5091636269205,-0.421325828350258,1.72680218931832));
#7609=CARTESIAN_POINT('Ctrl Pts',(95.5132254239558,-0.484757860705407,1.71007899243386));
#7610=CARTESIAN_POINT('Ctrl Pts',(95.5192359260755,-0.574970268013196,1.68087190865953));
#7611=CARTESIAN_POINT('Ctrl Pts',(95.5211088640415,-0.602595015656902,1.67116734277415));
#7612=CARTESIAN_POINT('Ctrl Pts',(95.5245490858155,-0.652314864208148,1.65230769089842));
#7613=CARTESIAN_POINT('Ctrl Pts',(95.5261090025806,-0.67448918367119,1.64338055235981));
#7614=CARTESIAN_POINT('Ctrl Pts',(95.5286095683612,-0.709399870739571,1.62850031125412));
#7615=CARTESIAN_POINT('Ctrl Pts',(95.5295403438087,-0.722257813532284,1.62283858470574));
#7616=CARTESIAN_POINT('Ctrl Pts',(95.5313140225818,-0.746492458131851,1.61182230444266));
#7617=CARTESIAN_POINT('Ctrl Pts',(95.5321558318,-0.757882154425968,1.60649829041125));
#7618=CARTESIAN_POINT('Ctrl Pts',(95.5340885011393,-0.783769149252214,1.59406108160048));
#7619=CARTESIAN_POINT('Ctrl Pts',(95.5351820099695,-0.798227703459158,1.58687028913103));
#7620=CARTESIAN_POINT('Ctrl Pts',(95.5386505529621,-0.843485118623139,1.56358702511387));
#7621=CARTESIAN_POINT('Ctrl Pts',(95.5410500675465,-0.873909275212359,1.54678822577836));
#7622=CARTESIAN_POINT('Ctrl Pts',(95.5528356447427,-1.01902314148532,1.46101491836367));
#7623=CARTESIAN_POINT('Ctrl Pts',(95.5626410462503,-1.12614720049667,1.38012838302095));
#7624=CARTESIAN_POINT('Ctrl Pts',(95.5777033090374,-1.27573075314451,1.23807589445349));
#7625=CARTESIAN_POINT('Ctrl Pts',(95.5829623415775,-1.32520412097489,1.18497127545016));
#7626=CARTESIAN_POINT('Ctrl Pts',(95.5892889151992,-1.38257129010113,1.11529160147115));
#7627=CARTESIAN_POINT('Ctrl Pts',(95.59052131656,-1.393640873137,1.1014281207151));
#7628=CARTESIAN_POINT('Ctrl Pts',(95.5923408599228,-1.40985105737297,1.08049082394988));
#7629=CARTESIAN_POINT('Ctrl Pts',(95.5929380802453,-1.41514977619948,1.07354158916254));
#7630=CARTESIAN_POINT('Ctrl Pts',(95.593963448654,-1.42421275628829,1.0614718404399));
#7631=CARTESIAN_POINT('Ctrl Pts',(95.5943932215669,-1.42800104920147,1.05636994003308));
#7632=CARTESIAN_POINT('Ctrl Pts',(95.595401375667,-1.43686282777616,1.04430051022357));
#7633=CARTESIAN_POINT('Ctrl Pts',(95.595978171669,-1.44191308033597,1.03731625746418));
#7634=CARTESIAN_POINT('Ctrl Pts',(95.5976913401766,-1.45684541072503,1.01634579049538));
#7635=CARTESIAN_POINT('Ctrl Pts',(95.5988181056185,-1.46657659785096,1.0022526889506));
#7636=CARTESIAN_POINT('Ctrl Pts',(95.6071188494788,-1.53743412762817,0.896391513343246));
#7637=CARTESIAN_POINT('Ctrl Pts',(95.613847156059,-1.59010891703738,0.799238145194436));
#7638=CARTESIAN_POINT('Ctrl Pts',(95.6254375979447,-1.66428917893848,0.625597948211356));
#7639=CARTESIAN_POINT('Ctrl Pts',(95.6302645246951,-1.69031630186238,0.551417209256785));
#7640=CARTESIAN_POINT('Ctrl Pts',(95.6382498467306,-1.7242052599363,0.429516284835134));
#7641=CARTESIAN_POINT('Ctrl Pts',(95.6413229183178,-1.73518096171951,0.382772023256816));
#7642=CARTESIAN_POINT('Ctrl Pts',(95.6456415182285,-1.74768269828848,0.317803856105381));
#7643=CARTESIAN_POINT('Ctrl Pts',(95.6468355615283,-1.75084157994094,0.299913031651014));
#7644=CARTESIAN_POINT('Ctrl Pts',(95.6488910804261,-1.7557701744631,0.269260219130472));
#7645=CARTESIAN_POINT('Ctrl Pts',(95.6497481709408,-1.75767650890935,0.256521434276438));
#7646=CARTESIAN_POINT('Ctrl Pts',(95.6513925762957,-1.76105040700204,0.232169185724215));
#7647=CARTESIAN_POINT('Ctrl Pts',(95.6521790809028,-1.76254204876103,0.220559701103775));
#7648=CARTESIAN_POINT('Ctrl Pts',(95.6540361131477,-1.76577774886916,0.193242737959454));
#7649=CARTESIAN_POINT('Ctrl Pts',(95.6551095624317,-1.76742710328808,0.177525267253876));
#7650=CARTESIAN_POINT('Ctrl Pts',(95.6589383313237,-1.77252977756963,0.121736630974516));
#7651=CARTESIAN_POINT('Ctrl Pts',(95.6617289029506,-1.77483144840728,0.08157511874713));
#7652=CARTESIAN_POINT('Ctrl Pts',(95.6735074028595,-1.77873129869303,-0.0858111367228625));
#7653=CARTESIAN_POINT('Ctrl Pts',(95.6828433037144,-1.76802159381666,-0.212931268975042));
#7654=CARTESIAN_POINT('Ctrl Pts',(95.6959240255116,-1.73393592621098,-0.388895171229194));
#7655=CARTESIAN_POINT('Ctrl Pts',(95.6997021873171,-1.72179549789788,-0.439538585422724));
#7656=CARTESIAN_POINT('Ctrl Pts',(95.7048925824717,-1.7017050882026,-0.509605655292844));
#7657=CARTESIAN_POINT('Ctrl Pts',(95.7063642489638,-1.6956104469003,-0.529531324781816));
#7658=CARTESIAN_POINT('Ctrl Pts',(95.7089314794952,-1.68424906163052,-0.564466080873819));
#7659=CARTESIAN_POINT('Ctrl Pts',(95.7100334310342,-1.67912875316064,-0.579520087998707));
#7660=CARTESIAN_POINT('Ctrl Pts',(95.7116990281738,-1.67100460468127,-0.602393367067877));
#7661=CARTESIAN_POINT('Ctrl Pts',(95.7122704957538,-1.66814661846772,-0.610263077739285));
#7662=CARTESIAN_POINT('Ctrl Pts',(95.7133196219961,-1.66276684639011,-0.624756514314161));
#7663=CARTESIAN_POINT('Ctrl Pts',(95.7137981320778,-1.66026100605841,-0.631385525644804));
#7664=CARTESIAN_POINT('Ctrl Pts',(95.7148985779523,-1.65437821466577,-0.646670789129523));
#7665=CARTESIAN_POINT('Ctrl Pts',(95.715518837265,-1.65097293702323,-0.655315769244813));
#7666=CARTESIAN_POINT('Ctrl Pts',(95.7175495539603,-1.63953441918701,-0.683699555264158));
#7667=CARTESIAN_POINT('Ctrl Pts',(95.7189441693934,-1.63121345768394,-0.703321368262269));
#7668=CARTESIAN_POINT('Ctrl Pts',(95.7277137753823,-1.576062593838,-0.827125750951435));
#7669=CARTESIAN_POINT('Ctrl Pts',(95.7346475210422,-1.51962304985306,-0.92674831504206));
#7670=CARTESIAN_POINT('Ctrl Pts',(95.7479492671776,-1.39526052170655,-1.10397905822821));
#7671=CARTESIAN_POINT('Ctrl Pts',(95.7542768642277,-1.32940943107528,-1.18245032989773));
#7672=CARTESIAN_POINT('Ctrl Pts',(95.7625026112235,-1.23944150553618,-1.27258761341929));
#7673=CARTESIAN_POINT('Ctrl Pts',(95.7641391680124,-1.22133005931005,-1.28997955935986));
#7674=CARTESIAN_POINT('Ctrl Pts',(95.7667337122914,-1.19233466205341,-1.31666495661527));
#7675=CARTESIAN_POINT('Ctrl Pts',(95.767680471494,-1.18169625332925,-1.32622113504322));
#7676=CARTESIAN_POINT('Ctrl Pts',(95.7694671940761,-1.1615198335759,-1.34390952480264));
#7677=CARTESIAN_POINT('Ctrl Pts',(95.7703058488285,-1.15200882540806,-1.35207129505764));
#7678=CARTESIAN_POINT('Ctrl Pts',(95.7722072941982,-1.13035942582877,-1.3702552299091));
#7679=CARTESIAN_POINT('Ctrl Pts',(95.77327241917,-1.1181727166752,-1.38021794455292));
#7680=CARTESIAN_POINT('Ctrl Pts',(95.7765549810348,-1.08044547891101,-1.41023259322138));
#7681=CARTESIAN_POINT('Ctrl Pts',(95.7787932961479,-1.05448743003822,-1.42974627789123));
#7682=CARTESIAN_POINT('Ctrl Pts',(95.7905669729014,-0.916829452409413,-1.52744064427992));
#7683=CARTESIAN_POINT('Ctrl Pts',(95.800549853815,-0.796948921754993,-1.59327075624083));
#7684=CARTESIAN_POINT('Ctrl Pts',(95.8158570789823,-0.602860632897499,-1.6724229264151));
#7685=CARTESIAN_POINT('Ctrl Pts',(95.8211773104897,-0.533316541880481,-1.69588174868033));
#7686=CARTESIAN_POINT('Ctrl Pts',(95.8275678407284,-0.445304538327723,-1.71961789223093));
#7687=CARTESIAN_POINT('Ctrl Pts',(95.8288064299105,-0.428023776423409,-1.72400044507977));
#7688=CARTESIAN_POINT('Ctrl Pts',(95.8306332314175,-0.40216101172052,-1.73014659489159));
#7689=CARTESIAN_POINT('Ctrl Pts',(95.8312316351064,-0.393627781506541,-1.73210793455745));
#7690=CARTESIAN_POINT('Ctrl Pts',(95.8322582480551,-0.378875940428328,-1.73538395610821));
#7691=CARTESIAN_POINT('Ctrl Pts',(95.832688095378,-0.372664411742228,-1.73672844542116));
#7692=CARTESIAN_POINT('Ctrl Pts',(95.8336952933583,-0.358027683410053,-1.73981442961415));
#7693=CARTESIAN_POINT('Ctrl Pts',(95.8342710718519,-0.349596891582212,-1.74152809127037));
#7694=CARTESIAN_POINT('Ctrl Pts',(95.8359780244609,-0.324425785132821,-1.7464542694911));
#7695=CARTESIAN_POINT('Ctrl Pts',(95.8370996947708,-0.307650789276348,-1.74948725343086));
#7696=CARTESIAN_POINT('Ctrl Pts',(95.8470885985108,-0.156447583644824,-1.77458316863787));
#7697=CARTESIAN_POINT('Ctrl Pts',(95.8552738483938,-0.019922168732767,-1.78135766408638));
#7698=CARTESIAN_POINT('Ctrl Pts',(95.8689370723993,0.201312685185786,-1.76687237439998));
#7699=CARTESIAN_POINT('Ctrl Pts',(95.8742622882672,0.286051313500328,-1.75514587297028));
#7700=CARTESIAN_POINT('Ctrl Pts',(95.8814434860663,0.394905414453724,-1.73198802296109));
#7701=CARTESIAN_POINT('Ctrl Pts',(95.8831277808173,0.420077630275489,-1.72605546592914));
#7702=CARTESIAN_POINT('Ctrl Pts',(95.8857808221302,0.459104114651419,-1.71595350175356));
#7703=CARTESIAN_POINT('Ctrl Pts',(95.8867374584725,0.473052763193094,-1.71216064395958));
#7704=CARTESIAN_POINT('Ctrl Pts',(95.8885328206763,0.498990362079987,-1.70476665505639));
#7705=CARTESIAN_POINT('Ctrl Pts',(95.8893701094222,0.510990615446308,-1.70120819029301));
#7706=CARTESIAN_POINT('Ctrl Pts',(95.8912551325656,0.537786188428529,-1.69295334120882));
#7707=CARTESIAN_POINT('Ctrl Pts',(95.8923050328096,0.552559410563726,-1.68818928768357));
#7708=CARTESIAN_POINT('Ctrl Pts',(95.8950195178779,0.59035782903476,-1.67545080313108));
#7709=CARTESIAN_POINT('Ctrl Pts',(95.8966931952179,0.613284143432193,-1.66719531459211));
#7710=CARTESIAN_POINT('Ctrl Pts',(95.9065212778656,0.745671858290243,-1.61642392883029));
#7711=CARTESIAN_POINT('Ctrl Pts',(95.915015636956,0.850853664247691,-1.5636150925841));
#7712=CARTESIAN_POINT('Ctrl Pts',(95.9290197240891,1.0126978104176,-1.46116608767325));
#7713=CARTESIAN_POINT('Ctrl Pts',(95.9344557472441,1.07281273015068,-1.41761665117643));
#7714=CARTESIAN_POINT('Ctrl Pts',(95.9416064787261,1.14979144342763,-1.35414166147278));
#7715=CARTESIAN_POINT('Ctrl Pts',(95.9434264528082,1.16919777194216,-1.3374216647518));
#7716=CARTESIAN_POINT('Ctrl Pts',(95.9465278324851,1.20204290686763,-1.30786158116165));
#7717=CARTESIAN_POINT('Ctrl Pts',(95.947819598296,1.21565409917173,-1.29521976694221));
#7718=CARTESIAN_POINT('Ctrl Pts',(95.9497086095095,1.23548909754919,-1.27620920220812));
#7719=CARTESIAN_POINT('Ctrl Pts',(95.9503170400925,1.24186688338772,-1.27000389387438));
#7720=CARTESIAN_POINT('Ctrl Pts',(95.9514013025132,1.25321758366416,-1.25879288518818));
#7721=CARTESIAN_POINT('Ctrl Pts',(95.9518784338275,1.25820758891953,-1.25380521121105));
#7722=CARTESIAN_POINT('Ctrl Pts',(95.9529466919265,1.26936835079225,-1.24251592781981));
#7723=CARTESIAN_POINT('Ctrl Pts',(95.9535365186582,1.27552203786981,-1.23619795342259));
#7724=CARTESIAN_POINT('Ctrl Pts',(95.9553304348032,1.294201073173,-1.21673225259117));
#7725=CARTESIAN_POINT('Ctrl Pts',(95.9565235260953,1.30657252251288,-1.20343761719195));
#7726=CARTESIAN_POINT('Ctrl Pts',(95.9632017706111,1.37535814647265,-1.12720763185612));
#7727=CARTESIAN_POINT('Ctrl Pts',(95.9684345601213,1.42743415394807,-1.0604914742689));
#7728=CARTESIAN_POINT('Ctrl Pts',(95.9782650772373,1.5165495807386,-0.927799566828433));
#7729=CARTESIAN_POINT('Ctrl Pts',(95.9828601390191,1.55451526920906,-0.862679909605681));
#7730=CARTESIAN_POINT('Ctrl Pts',(95.9904587312238,1.60921892190076,-0.753442197148421));
#7731=CARTESIAN_POINT('Ctrl Pts',(95.9934041099408,1.62853689295622,-0.710723439367341));
#7732=CARTESIAN_POINT('Ctrl Pts',(95.9985728161762,1.65891227367051,-0.635790536255283));
#7733=CARTESIAN_POINT('Ctrl Pts',(96.0007710000303,1.67077467838041,-0.603929855632468));
#7734=CARTESIAN_POINT('Ctrl Pts',(96.0040490325652,1.68687006018066,-0.556587756553879));
#7735=CARTESIAN_POINT('Ctrl Pts',(96.0051053581694,1.69181950793591,-0.54135686501542));
#7736=CARTESIAN_POINT('Ctrl Pts',(96.007002159096,1.70028153635546,-0.514066602218984));
#7737=CARTESIAN_POINT('Ctrl Pts',(96.0078399699372,1.70387346810471,-0.502032832754761));
#7738=CARTESIAN_POINT('Ctrl Pts',(96.0096291565387,1.71123401666494,-0.476384040351836));
#7739=CARTESIAN_POINT('Ctrl Pts',(96.0105815824227,1.71496839714795,-0.462760186676333));
#7740=CARTESIAN_POINT('Ctrl Pts',(96.013184972328,1.72467647158157,-0.425610440871128));
#7741=CARTESIAN_POINT('Ctrl Pts',(96.0148460540379,1.73033089524674,-0.402005062453215));
#7742=CARTESIAN_POINT('Ctrl Pts',(96.0242162553543,1.75922401354049,-0.269451460646902));
#7743=CARTESIAN_POINT('Ctrl Pts',(96.0322271973074,1.77263710159839,-0.158710346315969));
#7744=CARTESIAN_POINT('Ctrl Pts',(96.0403469459233,1.77561363956144,-0.0475422496666396));
#7745=CARTESIAN_POINT('Origin',(88.3562164250559,0.,0.));
#7746=CARTESIAN_POINT('',(96.9396785508644,1.77561363580749,-0.0475423898693833));
#7747=CARTESIAN_POINT('',(96.7921246218182,1.77561363837209,-0.0475422940869062));
#7748=CARTESIAN_POINT('',(88.3562164250559,1.77561363837197,-0.0475422940912398));
#7749=CARTESIAN_POINT('',(96.3799606556061,-0.00136080493914694,1.776249478736));
#7750=CARTESIAN_POINT('Ctrl Pts',(96.9396785508644,1.77561363580749,-0.0475423898693833));
#7751=CARTESIAN_POINT('Ctrl Pts',(96.9360093059474,1.77422561861672,-0.0993820693100051));
#7752=CARTESIAN_POINT('Ctrl Pts',(96.9322809403556,1.77056776805062,-0.151147512117908));
#7753=CARTESIAN_POINT('Ctrl Pts',(96.9191246470724,1.74988061234432,-0.331252339869889));
#7754=CARTESIAN_POINT('Ctrl Pts',(96.9095195712726,1.72110911674852,-0.45781568684712));
#7755=CARTESIAN_POINT('Ctrl Pts',(96.8988544704244,1.671736746555,-0.600694276812251));
#7756=CARTESIAN_POINT('Ctrl Pts',(96.897334790537,1.66425372143838,-0.621125606865727));
#7757=CARTESIAN_POINT('Ctrl Pts',(96.895227241329,1.65321617704534,-0.649629059745425));
#7758=CARTESIAN_POINT('Ctrl Pts',(96.8946231374856,1.64997441799014,-0.657819178349955));
#7759=CARTESIAN_POINT('Ctrl Pts',(96.8935342771295,1.64398687160514,-0.672623600189202));
#7760=CARTESIAN_POINT('Ctrl Pts',(96.8930483437481,1.6412617559151,-0.67924605086048));
#7761=CARTESIAN_POINT('Ctrl Pts',(96.8920361001067,1.63547226459627,-0.693077110426369));
#7762=CARTESIAN_POINT('Ctrl Pts',(96.8915102539116,1.6324001547973,-0.700282192993025));
#7763=CARTESIAN_POINT('Ctrl Pts',(96.890096070414,1.62396631454137,-0.719705138247724));
#7764=CARTESIAN_POINT('Ctrl Pts',(96.8892129699055,1.61851429843332,-0.731883576115109));
#7765=CARTESIAN_POINT('Ctrl Pts',(96.8842364908465,1.58676778662181,-0.800707182560501));
#7766=CARTESIAN_POINT('Ctrl Pts',(96.8802924573034,1.55763475141609,-0.856002179490291));
#7767=CARTESIAN_POINT('Ctrl Pts',(96.8713938245461,1.48434481681995,-0.978922127165139));
#7768=CARTESIAN_POINT('Ctrl Pts',(96.8664872959909,1.43837325200844,-1.04529953297451));
#7769=CARTESIAN_POINT('Ctrl Pts',(96.8558670927954,1.33086218804632,-1.17994479194519));
#7770=CARTESIAN_POINT('Ctrl Pts',(96.8501474548075,1.26822487890994,-1.24702305268568));
#7771=CARTESIAN_POINT('Ctrl Pts',(96.8427676440197,1.18436965890199,-1.32394240395596));
#7772=CARTESIAN_POINT('Ctrl Pts',(96.8413188746332,1.16776369362043,-1.33861228981251));
#7773=CARTESIAN_POINT('Ctrl Pts',(96.8389545435269,1.1404658331325,-1.36183294649985));
#7774=CARTESIAN_POINT('Ctrl Pts',(96.8380470216527,1.12994156612425,-1.37057773589062));
#7775=CARTESIAN_POINT('Ctrl Pts',(96.8362894626513,1.10947850720572,-1.3871849455467));
#7776=CARTESIAN_POINT('Ctrl Pts',(96.8354401849797,1.09955451380068,-1.39506433108703));
#7777=CARTESIAN_POINT('Ctrl Pts',(96.8334478251796,1.07619578153063,-1.41320645946733));
#7778=CARTESIAN_POINT('Ctrl Pts',(96.8323015038403,1.06269733787398,-1.4233847655494));
#7779=CARTESIAN_POINT('Ctrl Pts',(96.8284654965265,1.01734732216772,-1.45657560758094));
#7780=CARTESIAN_POINT('Ctrl Pts',(96.8257433391813,0.984879592647276,-1.4787223679309));
#7781=CARTESIAN_POINT('Ctrl Pts',(96.8189383221161,0.903064194746767,-1.53063971570956));
#7782=CARTESIAN_POINT('Ctrl Pts',(96.8148159662628,0.852953441844098,-1.55911905917351));
#7783=CARTESIAN_POINT('Ctrl Pts',(96.8084876862627,0.774972299625833,-1.59855219210809));
#7784=CARTESIAN_POINT('Ctrl Pts',(96.8063189488297,0.748059638292484,-1.6113217790696));
#7785=CARTESIAN_POINT('Ctrl Pts',(96.7958527604181,0.617045506082863,-1.66949576013225));
#7786=CARTESIAN_POINT('Ctrl Pts',(96.7874807863699,0.509064051667179,-1.70552597484869));
#7787=CARTESIAN_POINT('Ctrl Pts',(96.7783594449398,0.382084610481223,-1.73474921692463));
#7788=CARTESIAN_POINT('Ctrl Pts',(96.7771991858427,0.365741355284067,-1.73826833565245));
#7789=CARTESIAN_POINT('Ctrl Pts',(96.7754570551955,0.340875220570857,-1.74325639560033));
#7790=CARTESIAN_POINT('Ctrl Pts',(96.7748664987088,0.332387784988062,-1.74489459425764));
#7791=CARTESIAN_POINT('Ctrl Pts',(96.7738478964405,0.317641325929384,-1.74762937149171));
#7792=CARTESIAN_POINT('Ctrl Pts',(96.7734183021193,0.311388056323577,-1.7487543891584));
#7793=CARTESIAN_POINT('Ctrl Pts',(96.7724041406368,0.296545448095909,-1.75134256200132));
#7794=CARTESIAN_POINT('Ctrl Pts',(96.7718212348946,0.287951219612599,-1.75277610531714));
#7795=CARTESIAN_POINT('Ctrl Pts',(96.770070542777,0.261961442575343,-1.75691495883756));
#7796=CARTESIAN_POINT('Ctrl Pts',(96.7689129980151,0.244535310882353,-1.75942505076469));
#7797=CARTESIAN_POINT('Ctrl Pts',(96.7631274137211,0.156399475672966,-1.77078545666918));
#7798=CARTESIAN_POINT('Ctrl Pts',(96.7586775786044,0.0852327611901937,-1.77563496365505));
#7799=CARTESIAN_POINT('Ctrl Pts',(96.7462469852487,-0.116088409304546,-1.77721727461864));
#7800=CARTESIAN_POINT('Ctrl Pts',(96.7383913755706,-0.245847526516281,-1.76395441980391));
#7801=CARTESIAN_POINT('Ctrl Pts',(96.7277293221064,-0.4096228602677,-1.72877895969761));
#7802=CARTESIAN_POINT('Ctrl Pts',(96.7253153357333,-0.445990778436983,-1.71975564835071));
#7803=CARTESIAN_POINT('Ctrl Pts',(96.7218596093438,-0.496839121342897,-1.70541820048172));
#7804=CARTESIAN_POINT('Ctrl Pts',(96.7208482201852,-0.511578749778558,-1.70105482254783));
#7805=CARTESIAN_POINT('Ctrl Pts',(96.7189855107789,-0.538451957928767,-1.6927186746764));
#7806=CARTESIAN_POINT('Ctrl Pts',(96.7181361734394,-0.550602990733809,-1.68880530395462));
#7807=CARTESIAN_POINT('Ctrl Pts',(96.7163985709306,-0.575247283188849,-1.68057410707942));
#7808=CARTESIAN_POINT('Ctrl Pts',(96.7155100486443,-0.587736611889357,-1.67624712522501));
#7809=CARTESIAN_POINT('Ctrl Pts',(96.7132714615485,-0.618914248722107,-1.66505422815375));
#7810=CARTESIAN_POINT('Ctrl Pts',(96.7119156399892,-0.637537175345806,-1.65801288404216));
#7811=CARTESIAN_POINT('Ctrl Pts',(96.706188050881,-0.715095985380527,-1.62718796874745));
#7812=CARTESIAN_POINT('Ctrl Pts',(96.7017227651265,-0.772845611352546,-1.60056581526375));
#7813=CARTESIAN_POINT('Ctrl Pts',(96.6871908439572,-0.952443114142012,-1.50578419193227));
#7814=CARTESIAN_POINT('Ctrl Pts',(96.6768203460474,-1.06772991755214,-1.42635256114721));
#7815=CARTESIAN_POINT('Ctrl Pts',(96.6640216999793,-1.20169913623521,-1.30862187833408));
#7816=CARTESIAN_POINT('Ctrl Pts',(96.6612697156964,-1.23002287475852,-1.28203598420486));
#7817=CARTESIAN_POINT('Ctrl Pts',(96.657740092985,-1.26596594136532,-1.24600944134234));
#7818=CARTESIAN_POINT('Ctrl Pts',(96.6569099579442,-1.27439075388407,-1.23739141712105));
#7819=CARTESIAN_POINT('Ctrl Pts',(96.6555701103028,-1.28795157610974,-1.22323417041578));
#7820=CARTESIAN_POINT('Ctrl Pts',(96.6550564979998,-1.2931409524755,-1.21774692794425));
#7821=CARTESIAN_POINT('Ctrl Pts',(96.6540431740179,-1.30336441136377,-1.20679759859031));
#7822=CARTESIAN_POINT('Ctrl Pts',(96.653543395813,-1.30839951827122,-1.20133672943951));
#7823=CARTESIAN_POINT('Ctrl Pts',(96.6522781974598,-1.32112264184425,-1.18736287508338));
#7824=CARTESIAN_POINT('Ctrl Pts',(96.6515162572625,-1.32876288357837,-1.17880653561924));
#7825=CARTESIAN_POINT('Ctrl Pts',(96.6483389712748,-1.360499064883,-1.14256440286425));
#7826=CARTESIAN_POINT('Ctrl Pts',(96.6459739047634,-1.38381854093846,-1.11420725192121));
#7827=CARTESIAN_POINT('Ctrl Pts',(96.6391760797448,-1.44926410057058,-1.02939610599516));
#7828=CARTESIAN_POINT('Ctrl Pts',(96.634843734833,-1.48893365165142,-0.971133725175154));
#7829=CARTESIAN_POINT('Ctrl Pts',(96.6229771282697,-1.58801245031204,-0.805212074532495));
#7830=CARTESIAN_POINT('Ctrl Pts',(96.615469193436,-1.63986946771954,-0.693523012538193));
#7831=CARTESIAN_POINT('Ctrl Pts',(96.605995753295,-1.68765191166171,-0.554508930939387));
#7832=CARTESIAN_POINT('Ctrl Pts',(96.604423331374,-1.6950460714177,-0.53147705045719));
#7833=CARTESIAN_POINT('Ctrl Pts',(96.6018203058615,-1.70639458514099,-0.493478397115742));
#7834=CARTESIAN_POINT('Ctrl Pts',(96.6007987671682,-1.71062782577722,-0.478597769536734));
#7835=CARTESIAN_POINT('Ctrl Pts',(96.5989394484765,-1.71793261651852,-0.451584084712511));
#7836=CARTESIAN_POINT('Ctrl Pts',(96.5981039106108,-1.7210713667691,-0.439470132275238));
#7837=CARTESIAN_POINT('Ctrl Pts',(96.5962915322782,-1.72756889017515,-0.413255236254104));
#7838=CARTESIAN_POINT('Ctrl Pts',(96.5953133346457,-1.73088355559718,-0.399144404723195));
#7839=CARTESIAN_POINT('Ctrl Pts',(96.5925612298575,-1.73967188643625,-0.359561583582922));
#7840=CARTESIAN_POINT('Ctrl Pts',(96.5907751580764,-1.7447581849659,-0.334008316247691));
#7841=CARTESIAN_POINT('Ctrl Pts',(96.5829572510782,-1.76436231667799,-0.222794672062727));
#7842=CARTESIAN_POINT('Ctrl Pts',(96.5767519974262,-1.77314468288618,-0.136256793711199));
#7843=CARTESIAN_POINT('Ctrl Pts',(96.5607332307596,-1.77928215523848,0.0841847312820075));
#7844=CARTESIAN_POINT('Ctrl Pts',(96.5508064275624,-1.76790784823396,0.217799325124803));
#7845=CARTESIAN_POINT('Ctrl Pts',(96.5402093336297,-1.73820508027656,0.3660806167852));
#7846=CARTESIAN_POINT('Ctrl Pts',(96.5389906357336,-1.7345039792407,0.383233509929725));
#7847=CARTESIAN_POINT('Ctrl Pts',(96.5371871673338,-1.72858805696209,0.408806927476766));
#7848=CARTESIAN_POINT('Ctrl Pts',(96.5365925670625,-1.72656465479547,0.417270027035853));
#7849=CARTESIAN_POINT('Ctrl Pts',(96.5355220313824,-1.72278740173632,0.432570746793511));
#7850=CARTESIAN_POINT('Ctrl Pts',(96.5350449616162,-1.72105491804803,0.439413080720304));
#7851=CARTESIAN_POINT('Ctrl Pts',(96.5339631634434,-1.71701400318364,0.454981806028477));
#7852=CARTESIAN_POINT('Ctrl Pts',(96.5333599055038,-1.71467979450505,0.46370113443145));
#7853=CARTESIAN_POINT('Ctrl Pts',(96.5314804346736,-1.70715686030677,0.490968904495373));
#7854=CARTESIAN_POINT('Ctrl Pts',(96.5302167953181,-1.70173266897346,0.509451674044301));
#7855=CARTESIAN_POINT('Ctrl Pts',(96.527220429214,-1.68801680869621,0.553521969975682));
#7856=CARTESIAN_POINT('Ctrl Pts',(96.5255006036531,-1.67944238715746,0.579017045551026));
#7857=CARTESIAN_POINT('Ctrl Pts',(96.5186598692157,-1.64265427280525,0.680698307274408));
#7858=CARTESIAN_POINT('Ctrl Pts',(96.5136926065033,-1.60980699752699,0.755106888657162));
#7859=CARTESIAN_POINT('Ctrl Pts',(96.5021245887605,-1.52206767422841,0.921881756632036));
#7860=CARTESIAN_POINT('Ctrl Pts',(96.4955233611927,-1.46367586985561,1.01203037165438));
#7861=CARTESIAN_POINT('Ctrl Pts',(96.4870251661317,-1.38221816353613,1.11586354820601));
#7862=CARTESIAN_POINT('Ctrl Pts',(96.4854147864763,-1.3665122211505,1.13504306647039));
#7863=CARTESIAN_POINT('Ctrl Pts',(96.4827620665564,-1.34024760626116,1.1657809278241));
#7864=CARTESIAN_POINT('Ctrl Pts',(96.4817294090236,-1.32992811767511,1.17753980546898));
#7865=CARTESIAN_POINT('Ctrl Pts',(96.4798582806115,-1.31106925349879,1.19846500476759));
#7866=CARTESIAN_POINT('Ctrl Pts',(96.4790221868509,-1.30258559149896,1.20768030460096));
#7867=CARTESIAN_POINT('Ctrl Pts',(96.477272054403,-1.28471453510014,1.22668519402338));
#7868=CARTESIAN_POINT('Ctrl Pts',(96.476357353371,-1.27531108684119,1.23645849744996));
#7869=CARTESIAN_POINT('Ctrl Pts',(96.4738375456233,-1.24924077303768,1.26294041246723));
#7870=CARTESIAN_POINT('Ctrl Pts',(96.4722227460352,-1.23235190194515,1.27942553152099));
#7871=CARTESIAN_POINT('Ctrl Pts',(96.468565205041,-1.19371107125203,1.31566755683684));
#7872=CARTESIAN_POINT('Ctrl Pts',(96.4665150914687,-1.17178759817331,1.33523065235273));
#7873=CARTESIAN_POINT('Ctrl Pts',(96.4597987557615,-1.09911985597801,1.39690626094531));
#7874=CARTESIAN_POINT('Ctrl Pts',(96.455054658504,-1.04651757266186,1.43673624852704));
#7875=CARTESIAN_POINT('Ctrl Pts',(96.4430618778972,-0.90974733349233,1.52879473713312));
#7876=CARTESIAN_POINT('Ctrl Pts',(96.4357625293724,-0.823194267332992,1.57708757596209));
#7877=CARTESIAN_POINT('Ctrl Pts',(96.4258284794161,-0.697158952443633,1.63419330722842));
#7878=CARTESIAN_POINT('Ctrl Pts',(96.4230333717317,-0.660713497353632,1.64926546311315));
#7879=CARTESIAN_POINT('Ctrl Pts',(96.4194582617891,-0.61245683148005,1.66736537620701));
#7880=CARTESIAN_POINT('Ctrl Pts',(96.4186241161812,-0.601076381048696,1.67150168194804));
#7881=CARTESIAN_POINT('Ctrl Pts',(96.4172794336662,-0.582518580807284,1.67803259431247));
#7882=CARTESIAN_POINT('Ctrl Pts',(96.4167649467335,-0.575366888624275,1.68049820989801));
#7883=CARTESIAN_POINT('Ctrl Pts',(96.415751437447,-0.561172097585905,1.68529076219419));
#7884=CARTESIAN_POINT('Ctrl Pts',(96.4152523343324,-0.554129784599802,1.68761940674598));
#7885=CARTESIAN_POINT('Ctrl Pts',(96.4139911208785,-0.536208107210804,1.69342119527823));
#7886=CARTESIAN_POINT('Ctrl Pts',(96.4132324462594,-0.525309228327221,1.69683373096838));
#7887=CARTESIAN_POINT('Ctrl Pts',(96.4100895298802,-0.479704720221569,1.71063137956607));
#7888=CARTESIAN_POINT('Ctrl Pts',(96.407754219235,-0.444715976703036,1.7200594334633));
#7889=CARTESIAN_POINT('Ctrl Pts',(96.3967293572918,-0.275739721330435,1.76008990915589));
#7890=CARTESIAN_POINT('Ctrl Pts',(96.3885157802462,-0.138792400966149,1.77614419082633));
#7891=CARTESIAN_POINT('Ctrl Pts',(96.3799606556061,-0.00136080493914694,
1.776249478736));
#7892=CARTESIAN_POINT('Ctrl Pts',(96.3799605315711,-0.00135881241127846,
1.77624948026138));
#7893=CARTESIAN_POINT('Ctrl Pts',(96.3771359461598,0.0440159983497685,1.77628419152053));
#7894=CARTESIAN_POINT('Ctrl Pts',(96.3742821016252,0.0893735997216053,1.77458023586255));
#7895=CARTESIAN_POINT('Ctrl Pts',(96.3695680710927,0.162886034414931,1.76899295676369));
#7896=CARTESIAN_POINT('Ctrl Pts',(96.3677375691263,0.19110043961938,1.7661677226491));
#7897=CARTESIAN_POINT('Ctrl Pts',(96.3649791296725,0.233026948812799,1.76095306372232));
#7898=CARTESIAN_POINT('Ctrl Pts',(96.3640668564934,0.246798975789945,1.75907575138726));
#7899=CARTESIAN_POINT('Ctrl Pts',(96.3623740786795,0.272169704351601,1.75531358069128));
#7900=CARTESIAN_POINT('Ctrl Pts',(96.3615950548584,0.283774538716189,1.75347486850474));
#7901=CARTESIAN_POINT('Ctrl Pts',(96.3599756773798,0.307745227130418,1.74943267727441));
#7902=CARTESIAN_POINT('Ctrl Pts',(96.3591348485344,0.320107624437626,1.74721289827679));
#7903=CARTESIAN_POINT('Ctrl Pts',(96.3572114666753,0.348189162795337,1.74186257801504));
#7904=CARTESIAN_POINT('Ctrl Pts',(96.3561263583703,0.363891364543811,1.73865004505273));
#7905=CARTESIAN_POINT('Ctrl Pts',(96.3532543711735,0.4050708538016,1.72964281694881));
#7906=CARTESIAN_POINT('Ctrl Pts',(96.3514565297596,0.430466670761104,1.72349789391396));
#7907=CARTESIAN_POINT('Ctrl Pts',(96.3426606879059,0.552829861422637,1.6910170651083));
#7908=CARTESIAN_POINT('Ctrl Pts',(96.3354262629305,0.647566284091938,1.65704915401004));
#7909=CARTESIAN_POINT('Ctrl Pts',(96.319717491925,0.843306568021876,1.56750668510802));
#7910=CARTESIAN_POINT('Ctrl Pts',(96.3112477206887,0.942832950861685,1.50973931636731));
#7911=CARTESIAN_POINT('Ctrl Pts',(96.3019566656879,1.05049702935109,1.43242261165794));
#7912=CARTESIAN_POINT('Ctrl Pts',(96.3007246276125,1.06474629232017,1.42186284143817));
#7913=CARTESIAN_POINT('Ctrl Pts',(96.2989054973366,1.08577712208158,1.40578392785827));
#7914=CARTESIAN_POINT('Ctrl Pts',(96.2983083335792,1.09267950405553,1.40042562108768));
#7915=CARTESIAN_POINT('Ctrl Pts',(96.2972830095491,1.10453310351432,1.39108269663284));
#7916=CARTESIAN_POINT('Ctrl Pts',(96.2968532252188,1.10950276963026,1.38712222003486));
#7917=CARTESIAN_POINT('Ctrl Pts',(96.2958449657166,1.12116354053304,1.37772663523553));
#7918=CARTESIAN_POINT('Ctrl Pts',(96.2952680767584,1.12783646352564,1.37226939241132));
#7919=CARTESIAN_POINT('Ctrl Pts',(96.2935544052096,1.14765122798923,1.35582232979771));
#7920=CARTESIAN_POINT('Ctrl Pts',(96.2924272377111,1.16067451617624,1.34469039258165));
#7921=CARTESIAN_POINT('Ctrl Pts',(96.2841349700639,1.25620290138329,1.26061333673786));
#7922=CARTESIAN_POINT('Ctrl Pts',(96.2774143820565,1.33193652298923,1.18031492904804));
#7923=CARTESIAN_POINT('Ctrl Pts',(96.2658271491983,1.44814871144439,1.03155692990616));
#7924=CARTESIAN_POINT('Ctrl Pts',(96.2609953233858,1.49237785151521,0.966463456511067));
#7925=CARTESIAN_POINT('Ctrl Pts',(96.2530029689848,1.55644807866837,0.85722831253604));
#7926=CARTESIAN_POINT('Ctrl Pts',(96.2499279712534,1.57905592553948,0.814832963680922));
#7927=CARTESIAN_POINT('Ctrl Pts',(96.2456070837453,1.60781031903938,0.75520874340931));
#7928=CARTESIAN_POINT('Ctrl Pts',(96.2444127525875,1.61545188814941,0.738721479942792));
#7929=CARTESIAN_POINT('Ctrl Pts',(96.2423568678873,1.62807590441677,0.710351216477564));
#7930=CARTESIAN_POINT('Ctrl Pts',(96.2414997029326,1.63318456213679,0.698525713458277));
#7931=CARTESIAN_POINT('Ctrl Pts',(96.239855242837,1.64268869402638,0.675851252212387));
#7932=CARTESIAN_POINT('Ctrl Pts',(96.2390687588947,1.64710645001301,0.665012324340922));
#7933=CARTESIAN_POINT('Ctrl Pts',(96.2372119112794,1.65723568916024,0.639440075317252));
#7934=CARTESIAN_POINT('Ctrl Pts',(96.2361386277546,1.66285824846726,0.624672839685363));
#7935=CARTESIAN_POINT('Ctrl Pts',(96.2323114358717,1.6820840759176,0.572077914748872));
#7936=CARTESIAN_POINT('Ctrl Pts',(96.2295223155883,1.69459858847406,0.533868105591887));
#7937=CARTESIAN_POINT('Ctrl Pts',(96.217744075585,1.74128313488529,0.373077265965746));
#7938=CARTESIAN_POINT('Ctrl Pts',(96.2084067670488,1.76352441031514,0.247440391240251));
#7939=CARTESIAN_POINT('Ctrl Pts',(96.1950311507562,1.7759607034936,0.0645875547311537));
#7940=CARTESIAN_POINT('Ctrl Pts',(96.1909633780533,1.77711420189509,0.00850086325508087));
#7941=CARTESIAN_POINT('Ctrl Pts',(96.1869838792616,1.77561363799551,-0.0475423081512957));
#7942=CARTESIAN_POINT('Ctrl Pts',(96.0403469459233,1.77561363956144,-0.0475422496666412));
#7943=CARTESIAN_POINT('Ctrl Pts',(96.0429305947739,1.7765607537211,-0.0121693164989692));
#7944=CARTESIAN_POINT('Ctrl Pts',(96.0455230953014,1.77645125620421,0.0232470040897777));
#7945=CARTESIAN_POINT('Ctrl Pts',(96.0536670536774,1.77277018539353,0.134651230012726));
#7946=CARTESIAN_POINT('Ctrl Pts',(96.0591920699511,1.76538228751994,0.210410668352316));
#7947=CARTESIAN_POINT('Ctrl Pts',(96.0657959955279,1.75024958838739,0.303345449978323));
#7948=CARTESIAN_POINT('Ctrl Pts',(96.0670548596476,1.74706544865344,0.321176688500235));
#7949=CARTESIAN_POINT('Ctrl Pts',(96.0689054150075,1.74192774667112,0.347605246776164));
#7950=CARTESIAN_POINT('Ctrl Pts',(96.0695076718102,1.74018215381035,0.356241157197292));
#7951=CARTESIAN_POINT('Ctrl Pts',(96.0705857245962,1.73692306169425,0.371768905423816));
#7952=CARTESIAN_POINT('Ctrl Pts',(96.0710627467569,1.73543268868601,0.378665061297894));
#7953=CARTESIAN_POINT('Ctrl Pts',(96.072136694263,1.73196774586346,0.394247550244933));
#7954=CARTESIAN_POINT('Ctrl Pts',(96.0727322465169,1.72996888680125,0.402928111176793));
#7955=CARTESIAN_POINT('Ctrl Pts',(96.0745623518416,1.72358927002873,0.429710288731958));
#7956=CARTESIAN_POINT('Ctrl Pts',(96.0757852531339,1.718988910735,0.447758971005908));
#7957=CARTESIAN_POINT('Ctrl Pts',(96.0856944615445,1.67901004470484,0.594899098207155));
#7958=CARTESIAN_POINT('Ctrl Pts',(96.0937415366243,1.62942271619631,0.719702123240553));
#7959=CARTESIAN_POINT('Ctrl Pts',(96.1072532047551,1.52601761048561,0.913028002144553));
#7960=CARTESIAN_POINT('Ctrl Pts',(96.112573263114,1.48039082549657,0.985287010657162));
#7961=CARTESIAN_POINT('Ctrl Pts',(96.1197481772966,1.41441283712687,1.07478765958966));
#7962=CARTESIAN_POINT('Ctrl Pts',(96.1214317220378,1.39862358250974,1.09525529010562));
#7963=CARTESIAN_POINT('Ctrl Pts',(96.124083844661,1.37331873206725,1.12661821322305));
#7964=CARTESIAN_POINT('Ctrl Pts',(96.1250403264075,1.3641067679079,1.13775464982094));
#7965=CARTESIAN_POINT('Ctrl Pts',(96.1268355504355,1.34666495163778,1.15832389379713));
#7966=CARTESIAN_POINT('Ctrl Pts',(96.1276728575929,1.33846924430396,1.16778457050768));
#7967=CARTESIAN_POINT('Ctrl Pts',(96.1295581232069,1.3198854016086,1.18878409624206));
#7968=CARTESIAN_POINT('Ctrl Pts',(96.1306082500195,1.30944469720809,1.20027482647593));
#7969=CARTESIAN_POINT('Ctrl Pts',(96.133323738823,1.28222672909368,1.22945228491238));
#7970=CARTESIAN_POINT('Ctrl Pts',(96.134998204742,1.26523403643993,1.24693265100488));
#7971=CARTESIAN_POINT('Ctrl Pts',(96.1447955454228,1.16464765006783,1.34623237311867));
#7972=CARTESIAN_POINT('Ctrl Pts',(96.1532554314745,1.07350776921719,1.41997119366398));
#7973=CARTESIAN_POINT('Ctrl Pts',(96.1672492962213,0.913567196571819,1.52512499028642));
#7974=CARTESIAN_POINT('Ctrl Pts',(96.1727096330583,0.848818828398172,1.5620879575303));
#7975=CARTESIAN_POINT('Ctrl Pts',(96.1798884341912,0.758887891755748,1.60617940948923));
#7976=CARTESIAN_POINT('Ctrl Pts',(96.181712866031,0.735593470474882,1.61698036824198));
#7977=CARTESIAN_POINT('Ctrl Pts',(96.1848209852281,0.695025401393963,1.63473238772244));
#7978=CARTESIAN_POINT('Ctrl Pts',(96.1861150890555,0.677861859100586,1.64192376694141));
#7979=CARTESIAN_POINT('Ctrl Pts',(96.1880068286817,0.652322081780324,1.65215593991399));
#7980=CARTESIAN_POINT('Ctrl Pts',(96.1886156942732,0.644031500587317,1.65540532287018));
#7981=CARTESIAN_POINT('Ctrl Pts',(96.1897003983767,0.629128596796746,1.66111740984336));
#7982=CARTESIAN_POINT('Ctrl Pts',(96.1901775415121,0.622525668807706,1.66360320898977));
#7983=CARTESIAN_POINT('Ctrl Pts',(96.1912454169857,0.607641290655673,1.6691056877951));
#7984=CARTESIAN_POINT('Ctrl Pts',(96.1918348542588,0.599352013488451,1.67210014870824));
#7985=CARTESIAN_POINT('Ctrl Pts',(96.1936263250468,0.573946447942976,1.68106458177001));
#7986=CARTESIAN_POINT('Ctrl Pts',(96.1948174039312,0.556760175894033,1.68683455684777));
#7987=CARTESIAN_POINT('Ctrl Pts',(96.2020621255761,0.450641824788726,1.72066317898613));
#7988=CARTESIAN_POINT('Ctrl Pts',(96.2078058695158,0.359692029100929,1.74194883450128));
#7989=CARTESIAN_POINT('Ctrl Pts',(96.2190111548587,0.179330225747883,1.76942242407391));
#7990=CARTESIAN_POINT('Ctrl Pts',(96.2244597500703,0.0902975448931025,1.77619263733928));
#7991=CARTESIAN_POINT('Ctrl Pts',(96.2332640174644,-0.0496013302610995,
1.77628207226836));
#7992=CARTESIAN_POINT('Ctrl Pts',(96.2365037790513,-0.100312206868422,1.77414064584529));
#7993=CARTESIAN_POINT('Ctrl Pts',(96.2410517104331,-0.169842546179014,1.76821395150884));
#7994=CARTESIAN_POINT('Ctrl Pts',(96.2423023789833,-0.188798532341161,1.76629050181665));
#7995=CARTESIAN_POINT('Ctrl Pts',(96.2443394016273,-0.219382454270107,1.7626892283897));
#7996=CARTESIAN_POINT('Ctrl Pts',(96.245119784636,-0.231031430532863,1.76120028501954));
#7997=CARTESIAN_POINT('Ctrl Pts',(96.2467614032788,-0.255388744886605,1.75784118617991));
#7998=CARTESIAN_POINT('Ctrl Pts',(96.2476233082744,-0.268093229966685,1.75594847642369));
#7999=CARTESIAN_POINT('Ctrl Pts',(96.249701407859,-0.298516383411224,1.75107818949044));
#8000=CARTESIAN_POINT('Ctrl Pts',(96.2509216936409,-0.316212274917905,1.74796928251198));
#8001=CARTESIAN_POINT('Ctrl Pts',(96.2553311850609,-0.379531801574689,1.73585201604046));
#8002=CARTESIAN_POINT('Ctrl Pts',(96.2585677481278,-0.42484132560191,1.72532193241922));
#8003=CARTESIAN_POINT('Ctrl Pts',(96.2671243581273,-0.541597006854946,1.69330956313051));
#8004=CARTESIAN_POINT('Ctrl Pts',(96.272516992436,-0.612191989460444,1.66908465702206));
#8005=CARTESIAN_POINT('Ctrl Pts',(96.2865036993469,-0.789212022949411,1.59559513393595));
#8006=CARTESIAN_POINT('Ctrl Pts',(96.2951473848639,-0.892675143316029,1.5401020788303));
#8007=CARTESIAN_POINT('Ctrl Pts',(96.3044877645388,-1.00352385081625,1.46569849458347));
#8008=CARTESIAN_POINT('Ctrl Pts',(96.3056238031913,-1.0169936440536,1.45638462358153));
#8009=CARTESIAN_POINT('Ctrl Pts',(96.3073370571403,-1.03731557726136,1.44191328793803));
#8010=CARTESIAN_POINT('Ctrl Pts',(96.3079225502138,-1.0442619650909,1.43689056393344));
#8011=CARTESIAN_POINT('Ctrl Pts',(96.3089797874547,-1.05681272686145,1.42767639593554));
#8012=CARTESIAN_POINT('Ctrl Pts',(96.3094526024021,-1.06242890223962,1.42350197125741));
#8013=CARTESIAN_POINT('Ctrl Pts',(96.3105377059455,-1.07532401676266,1.41379838235499));
#8014=CARTESIAN_POINT('Ctrl Pts',(96.3111483870352,-1.08258512229333,1.40824609677859));
#8015=CARTESIAN_POINT('Ctrl Pts',(96.3130763915856,-1.10550813790064,1.39043567151691));
#8016=CARTESIAN_POINT('Ctrl Pts',(96.3143801998682,-1.12100779813375,1.37796995504197));
#8017=CARTESIAN_POINT('Ctrl Pts',(96.3174917772527,-1.15788567820576,1.34727645706107));
#8018=CARTESIAN_POINT('Ctrl Pts',(96.3192852768906,-1.17904766352649,1.32879640039378));
#8019=CARTESIAN_POINT('Ctrl Pts',(96.3266447849985,-1.26497907830156,1.25008537108752));
#8020=CARTESIAN_POINT('Ctrl Pts',(96.3320328771673,-1.32564632861231,1.18555864382153));
#8021=CARTESIAN_POINT('Ctrl Pts',(96.3440149301448,-1.44826292070771,1.03390349240651));
#8022=CARTESIAN_POINT('Ctrl Pts',(96.3506131582488,-1.50766587335273,0.945178043956437));
#8023=CARTESIAN_POINT('Ctrl Pts',(96.3589860392484,-1.5696110079357,0.831803977510228));
#8024=CARTESIAN_POINT('Ctrl Pts',(96.3604655216718,-1.58008451500923,0.811732359071696));
#8025=CARTESIAN_POINT('Ctrl Pts',(96.3628674593071,-1.59631312264466,0.779126739895723));
#8026=CARTESIAN_POINT('Ctrl Pts',(96.3637813830707,-1.60231105673727,0.766715932849892));
#8027=CARTESIAN_POINT('Ctrl Pts',(96.3655429361139,-1.61353013802961,0.742794905873446));
#8028=CARTESIAN_POINT('Ctrl Pts',(96.3663897100565,-1.61877408507284,0.731296263990779));
#8029=CARTESIAN_POINT('Ctrl Pts',(96.3683634329026,-1.6306500609846,0.704501508135821));
#8030=CARTESIAN_POINT('Ctrl Pts',(96.3694934375602,-1.63719023074581,0.68916624379013));
#8031=CARTESIAN_POINT('Ctrl Pts',(96.3732127549297,-1.65786798179438,0.638725305186988));
#8032=CARTESIAN_POINT('Ctrl Pts',(96.3758318742429,-1.67109881218692,0.603261670587379));
#8033=CARTESIAN_POINT('Ctrl Pts',(96.3823112229407,-1.70061124914197,0.515714072397891));
#8034=CARTESIAN_POINT('Ctrl Pts',(96.3862060737616,-1.71564442895074,0.463252513849962));
#8035=CARTESIAN_POINT('Ctrl Pts',(96.3920633671962,-1.73435957616409,0.384399954820618));
#8036=CARTESIAN_POINT('Ctrl Pts',(96.3939889571552,-1.73990180156531,0.358480295225153));
#8037=CARTESIAN_POINT('Ctrl Pts',(96.4041006893171,-1.76586579546782,0.222207165366694));
#8038=CARTESIAN_POINT('Ctrl Pts',(96.4123882134443,-1.77637602342196,0.110220894126013));
#8039=CARTESIAN_POINT('Ctrl Pts',(96.4219356337484,-1.77622292108002,-0.0249058862137763));
#8040=CARTESIAN_POINT('Ctrl Pts',(96.4235367073418,-1.77575438786865,-0.0477979414076611));
#8041=CARTESIAN_POINT('Ctrl Pts',(96.4257369128305,-1.77448549307923,-0.0796630104551556));
#8042=CARTESIAN_POINT('Ctrl Pts',(96.4263541214217,-1.77405934820833,-0.0886476058793519));
#8043=CARTESIAN_POINT('Ctrl Pts',(96.4274592574622,-1.77316887393021,-0.104824326006481));
#8044=CARTESIAN_POINT('Ctrl Pts',(96.4279484807638,-1.77272898713365,-0.11201758910826));
#8045=CARTESIAN_POINT('Ctrl Pts',(96.4289580706819,-1.77172574007857,-0.126932662859727));
#8046=CARTESIAN_POINT('Ctrl Pts',(96.4294780672173,-1.77115565795979,-0.134653778236111));
#8047=CARTESIAN_POINT('Ctrl Pts',(96.430859039143,-1.76949909525797,-0.15525488560299));
#8048=CARTESIAN_POINT('Ctrl Pts',(96.4317151909711,-1.76832245787829,-0.168127442025727));
#8049=CARTESIAN_POINT('Ctrl Pts',(96.4361606407028,-1.76143035413475,-0.235416363585029));
#8050=CARTESIAN_POINT('Ctrl Pts',(96.4396357816746,-1.75334276350391,-0.289565461497547));
#8051=CARTESIAN_POINT('Ctrl Pts',(96.4518478839361,-1.7155738740101,-0.48132212391297));
#8052=CARTESIAN_POINT('Ctrl Pts',(96.4602674316417,-1.67207244681705,-0.615662730493593));
#8053=CARTESIAN_POINT('Ctrl Pts',(96.4721491277466,-1.59324143018987,-0.786710336662938));
#8054=CARTESIAN_POINT('Ctrl Pts',(96.4751958222187,-1.57158171838095,-0.829133103648108));
#8055=CARTESIAN_POINT('Ctrl Pts',(96.4795158378172,-1.53911593211159,-0.886867033379799));
#8056=CARTESIAN_POINT('Ctrl Pts',(96.4807392228008,-1.52973190582593,-0.902956942727873));
#8057=CARTESIAN_POINT('Ctrl Pts',(96.4827440000593,-1.51405971622055,-0.928882892035104));
#8058=CARTESIAN_POINT('Ctrl Pts',(96.4835197970066,-1.50792440146361,-0.93881001261809));
#8059=CARTESIAN_POINT('Ctrl Pts',(96.485161869898,-1.49479355162338,-0.959595291276738));
#8060=CARTESIAN_POINT('Ctrl Pts',(96.4860289095425,-1.48777653469146,-0.97043899990679));
#8061=CARTESIAN_POINT('Ctrl Pts',(96.4881393193162,-1.47049946272533,-0.996510167248802));
#8062=CARTESIAN_POINT('Ctrl Pts',(96.4893871067741,-1.46012052952907,-1.01165665040451));
#8063=CARTESIAN_POINT('Ctrl Pts',(96.4940313797154,-1.42090299781262,-1.06702778179582));
#8064=CARTESIAN_POINT('Ctrl Pts',(96.49748219682,-1.39062410456743,-1.10619952662017));
#8065=CARTESIAN_POINT('Ctrl Pts',(96.5068460732315,-1.30549852244011,-1.20730020674722));
#8066=CARTESIAN_POINT('Ctrl Pts',(96.5128512574472,-1.24789914464058,-1.26674600555088));
#8067=CARTESIAN_POINT('Ctrl Pts',(96.5264416373767,-1.10953018681088,-1.3909234703311));
#8068=CARTESIAN_POINT('Ctrl Pts',(96.5340262472109,-1.02681155116719,-1.45306120981445));
#8069=CARTESIAN_POINT('Ctrl Pts',(96.5425050795468,-0.924134324972083,-1.51702111036533));
#8070=CARTESIAN_POINT('Ctrl Pts',(96.5437346179634,-0.908972255393016,-1.52615425114478));
#8071=CARTESIAN_POINT('Ctrl Pts',(96.5455508018133,-0.886130283236608,-1.53945230824795));
#8072=CARTESIAN_POINT('Ctrl Pts',(96.5461474734486,-0.878552575863178,-1.54378938582509));
#8073=CARTESIAN_POINT('Ctrl Pts',(96.5472200098624,-0.864792511976391,-1.55153078461017));
#8074=CARTESIAN_POINT('Ctrl Pts',(96.5476970340651,-0.858621571191204,-1.55495429702979));
#8075=CARTESIAN_POINT('Ctrl Pts',(96.5487765738756,-0.844540855101335,-1.5626566062066));
#8076=CARTESIAN_POINT('Ctrl Pts',(96.5493776464294,-0.836618809330666,-1.56691221880814));
#8077=CARTESIAN_POINT('Ctrl Pts',(96.551243080958,-0.811789057644641,-1.58000841642962));
#8078=CARTESIAN_POINT('Ctrl Pts',(96.5524951347937,-0.794770389611333,-1.58863720526073));
#8079=CARTESIAN_POINT('Ctrl Pts',(96.5554585327273,-0.753742116818432,-1.60861491124368));
#8080=CARTESIAN_POINT('Ctrl Pts',(96.5571573528449,-0.729610139254469,-1.61970315313515));
#8081=CARTESIAN_POINT('Ctrl Pts',(96.5638571617283,-0.632460043549448,-1.66172984783569));
#8082=CARTESIAN_POINT('Ctrl Pts',(96.5687108282092,-0.557651250579835,-1.68830641348407));
#8083=CARTESIAN_POINT('Ctrl Pts',(96.5803478917882,-0.375155249633172,-1.73967956813267));
#8084=CARTESIAN_POINT('Ctrl Pts',(96.5871305227646,-0.266457729055983,-1.7596087985455));
#8085=CARTESIAN_POINT('Ctrl Pts',(96.5958125007933,-0.132207570211483,-1.77149255555919));
#8086=CARTESIAN_POINT('Ctrl Pts',(96.5974051789182,-0.107753695154972,-1.77314798134366));
#8087=CARTESIAN_POINT('Ctrl Pts',(96.600034712005,-0.0677279813718079,-1.77502653611153));
#8088=CARTESIAN_POINT('Ctrl Pts',(96.6010621743621,-0.0521731590333654,
-1.77555180693419));
#8089=CARTESIAN_POINT('Ctrl Pts',(96.6029277325171,-0.024097086011011,-1.77613066209162));
#8090=CARTESIAN_POINT('Ctrl Pts',(96.6037635139506,-0.0115782317456789,
-1.77625638045931));
#8091=CARTESIAN_POINT('Ctrl Pts',(96.6055712791055,0.0153650730629895,-1.77624211229682));
#8092=CARTESIAN_POINT('Ctrl Pts',(96.606544562844,0.0297884983151368,-1.77605876899343));
#8093=CARTESIAN_POINT('Ctrl Pts',(96.6092681825941,0.0699110680632635,-1.77505987962055));
#8094=CARTESIAN_POINT('Ctrl Pts',(96.6110302787581,0.0955962382527541,-1.77386199356287));
#8095=CARTESIAN_POINT('Ctrl Pts',(96.6186465448605,0.205403068147676,-1.76634915506463));
#8096=CARTESIAN_POINT('Ctrl Pts',(96.6246636818704,0.289032029862484,-1.75460441867524));
#8097=CARTESIAN_POINT('Ctrl Pts',(96.640089302414,0.496909221935101,-1.71014389116129));
#8098=CARTESIAN_POINT('Ctrl Pts',(96.6496061101153,0.619044508931569,-1.66981919887867));
#8099=CARTESIAN_POINT('Ctrl Pts',(96.6602723154879,0.756472068764938,-1.607274458543));
#8100=CARTESIAN_POINT('Ctrl Pts',(96.6618624219181,0.776987924297431,-1.59745768641492));
#8101=CARTESIAN_POINT('Ctrl Pts',(96.6640501907187,0.805326124750116,-1.58322277429939));
#8102=CARTESIAN_POINT('Ctrl Pts',(96.6646656761367,0.813311121542918,-1.57913569663409));
#8103=CARTESIAN_POINT('Ctrl Pts',(96.6657686595379,0.827649421922248,-1.57165910435213));
#8104=CARTESIAN_POINT('Ctrl Pts',(96.6662574377991,0.83401371977274,-1.56829111725617));
#8105=CARTESIAN_POINT('Ctrl Pts',(96.6672673201938,0.847188129075107,-1.56121633576739));
#8106=CARTESIAN_POINT('Ctrl Pts',(96.6677880423197,0.853994723795976,-1.55750351223451));
#8107=CARTESIAN_POINT('Ctrl Pts',(96.6691731381417,0.8721284908976,-1.54745738675956));
#8108=CARTESIAN_POINT('Ctrl Pts',(96.6700326376638,0.883411183373555,-1.54104418301764));
#8109=CARTESIAN_POINT('Ctrl Pts',(96.6745377654946,0.942637930946875,-1.50651479581373));
#8110=CARTESIAN_POINT('Ctrl Pts',(96.6780655359865,0.989317791106444,-1.47628069982322));
#8111=CARTESIAN_POINT('Ctrl Pts',(96.689945931623,1.14396695557424,-1.36547992972549));
#8112=CARTESIAN_POINT('Ctrl Pts',(96.6980172235576,1.24415374654073,-1.27486438901223));
#8113=CARTESIAN_POINT('Ctrl Pts',(96.7097268330864,1.36718145418235,-1.13513535636418));
#8114=CARTESIAN_POINT('Ctrl Pts',(96.7130144029842,1.39952055358183,-1.09501546842448));
#8115=CARTESIAN_POINT('Ctrl Pts',(96.7176183032336,1.44142704974603,-1.0381323763672));
#8116=CARTESIAN_POINT('Ctrl Pts',(96.7188751648333,1.45253485041673,-1.02253275354074));
#8117=CARTESIAN_POINT('Ctrl Pts',(96.7209195284333,1.47005376763467,-0.997067849906867));
#8118=CARTESIAN_POINT('Ctrl Pts',(96.7217009729549,1.47662306765102,-0.987312859135083));
#8119=CARTESIAN_POINT('Ctrl Pts',(96.7233426119769,1.49015535386034,-0.966781097631948));
#8120=CARTESIAN_POINT('Ctrl Pts',(96.7242034552566,1.49709938928443,-0.955992715975454));
#8121=CARTESIAN_POINT('Ctrl Pts',(96.7262747434513,1.51344123132743,-0.929988981057599));
#8122=CARTESIAN_POINT('Ctrl Pts',(96.7274892112717,1.52272715137805,-0.914705333504172));
#8123=CARTESIAN_POINT('Ctrl Pts',(96.7318506890216,1.55501601619991,-0.859706667257943));
#8124=CARTESIAN_POINT('Ctrl Pts',(96.735043694123,1.5767069529734,-0.819246536161576));
#8125=CARTESIAN_POINT('Ctrl Pts',(96.7434425754164,1.62878217932912,-0.712364092350434));
#8126=CARTESIAN_POINT('Ctrl Pts',(96.7487175546672,1.65667916698548,-0.644830401763326));
#8127=CARTESIAN_POINT('Ctrl Pts',(96.7627968283574,1.71924971914142,-0.46222569635848));
#8128=CARTESIAN_POINT('Ctrl Pts',(96.7716645787291,1.7465511271665,-0.345014884656039));
#8129=CARTESIAN_POINT('Ctrl Pts',(96.7811810998427,1.76386280466687,-0.210022825954433));
#8130=CARTESIAN_POINT('Ctrl Pts',(96.7822939260873,1.76568833496166,-0.194078154182664));
#8131=CARTESIAN_POINT('Ctrl Pts',(96.7839794602016,1.76815013766352,-0.169650935814082));
#8132=CARTESIAN_POINT('Ctrl Pts',(96.7845600632623,1.76894195155957,-0.161185386670087));
#8133=CARTESIAN_POINT('Ctrl Pts',(96.7856173569261,1.77028092814129,-0.145669149656872));
#8134=CARTESIAN_POINT('Ctrl Pts',(96.786095012061,1.77084679814569,-0.138620656056731));
#8135=CARTESIAN_POINT('Ctrl Pts',(96.7871934042979,1.77205718347817,-0.122324659259793));
#8136=CARTESIAN_POINT('Ctrl Pts',(96.7878124725179,1.77267142432164,-0.113075261067244));
#8137=CARTESIAN_POINT('Ctrl Pts',(96.7896744186737,1.7743107609307,-0.0850762327700656));
#8138=CARTESIAN_POINT('Ctrl Pts',(96.7909057720709,1.77511101730436,-0.0663142284229205));
#8139=CARTESIAN_POINT('Ctrl Pts',(96.7921246218182,1.77561363837209,-0.0475422940869062));
#8140=CARTESIAN_POINT('Origin',(88.3562164250559,0.,0.));
#8141=CARTESIAN_POINT('',(97.6892780485025,1.77561363630377,-0.0475423713344133));
#8142=CARTESIAN_POINT('',(97.5395353031289,1.77561364475627,-0.0475420556493824));
#8143=CARTESIAN_POINT('',(88.3562164250559,1.77561363837197,-0.0475422940912398));
#8144=CARTESIAN_POINT('Ctrl Pts',(97.6892780485025,1.77561363630377,-0.0475423713344133));
#8145=CARTESIAN_POINT('Ctrl Pts',(97.6860851367942,1.7742455753338,-0.098636745581963));
#8146=CARTESIAN_POINT('Ctrl Pts',(97.6828502987857,1.77067243241096,-0.149661107924927));
#8147=CARTESIAN_POINT('Ctrl Pts',(97.6778872795951,1.76199269377043,-0.226074449728626));
#8148=CARTESIAN_POINT('Ctrl Pts',(97.6762089950545,1.75852819260191,-0.251607622260889));
#8149=CARTESIAN_POINT('Ctrl Pts',(97.6735632941531,1.75225805166211,-0.291314566887335));
#8150=CARTESIAN_POINT('Ctrl Pts',(97.6726078751094,1.74983269179659,-0.30554539190279));
#8151=CARTESIAN_POINT('Ctrl Pts',(97.6708135629497,1.74498066720861,-0.332059115408676));
#8152=CARTESIAN_POINT('Ctrl Pts',(97.6699760909007,1.74259705634423,-0.344349053175954));
#8153=CARTESIAN_POINT('Ctrl Pts',(97.668089017505,1.73696201122558,-0.371845146531463));
#8154=CARTESIAN_POINT('Ctrl Pts',(97.6670372296867,1.73364044114145,-0.38703570302432));
#8155=CARTESIAN_POINT('Ctrl Pts',(97.6643144480537,1.72458210704467,-0.426003313583445));
#8156=CARTESIAN_POINT('Ctrl Pts',(97.6626342676826,1.71855304858058,-0.449708330764711));
#8157=CARTESIAN_POINT('Ctrl Pts',(97.6530897555053,1.68186805120106,-0.58241205918583));
#8158=CARTESIAN_POINT('Ctrl Pts',(97.6449119597441,1.64133880184685,-0.688391596023122));
#8159=CARTESIAN_POINT('Ctrl Pts',(97.6310005188252,1.55670350694662,-0.858889850223094));
#8160=CARTESIAN_POINT('Ctrl Pts',(97.6253386875275,1.51792806652487,-0.925695892344974));
#8161=CARTESIAN_POINT('Ctrl Pts',(97.6179279154381,1.46034812331345,-1.01149997829049));
#8162=CARTESIAN_POINT('Ctrl Pts',(97.6160671760906,1.44528724671633,-1.03290549710349));
#8163=CARTESIAN_POINT('Ctrl Pts',(97.6129042420688,1.41855892678731,-1.06916362510806));
#8164=CARTESIAN_POINT('Ctrl Pts',(97.6115911680215,1.40711775137802,-1.08417710314031));
#8165=CARTESIAN_POINT('Ctrl Pts',(97.6096772980609,1.3898985829476,-1.10604076472857));
#8166=CARTESIAN_POINT('Ctrl Pts',(97.609064907682,1.38430501417714,-1.11303363855099));
#8167=CARTESIAN_POINT('Ctrl Pts',(97.6079765881981,1.37420938251813,-1.12546098455746));
#8168=CARTESIAN_POINT('Ctrl Pts',(97.6074993130242,1.36972755906712,-1.13091125804803));
#8169=CARTESIAN_POINT('Ctrl Pts',(97.6064343912579,1.35960498133772,-1.14307270331917));
#8170=CARTESIAN_POINT('Ctrl Pts',(97.6058480004248,1.35394690022151,-1.14976898107994));
#8171=CARTESIAN_POINT('Ctrl Pts',(97.6040756557549,1.33659758303948,-1.16999603141518));
#8172=CARTESIAN_POINT('Ctrl Pts',(97.6029003189752,1.32475099769636,-1.18339286237959));
#8173=CARTESIAN_POINT('Ctrl Pts',(97.5954625188914,1.24775107531066,-1.26786328036346));
#8174=CARTESIAN_POINT('Ctrl Pts',(97.5895337426477,1.17709629497725,-1.33371998978517));
#8175=CARTESIAN_POINT('Ctrl Pts',(97.5806755662456,1.06391453497321,-1.42317861191845));
#8176=CARTESIAN_POINT('Ctrl Pts',(97.5777455429909,1.02521054317239,-1.4513079431965));
#8177=CARTESIAN_POINT('Ctrl Pts',(97.5713205616504,0.938716378206845,-1.50898195869091));
#8178=CARTESIAN_POINT('Ctrl Pts',(97.5678191601895,0.890566680024818,-1.5378898829842));
#8179=CARTESIAN_POINT('Ctrl Pts',(97.5617913582137,0.807132920930405,-1.58274778755483));
#8180=CARTESIAN_POINT('Ctrl Pts',(97.5593039128058,0.772549516970274,-1.59991281346182));
#8181=CARTESIAN_POINT('Ctrl Pts',(97.555678680275,0.722157435175025,-1.6229093512226));
#8182=CARTESIAN_POINT('Ctrl Pts',(97.554572438951,0.706780878128642,-1.6296646531436));
#8183=CARTESIAN_POINT('Ctrl Pts',(97.5526195067215,0.679653569629399,-1.64112621400613));
#8184=CARTESIAN_POINT('Ctrl Pts',(97.5517760901293,0.66794382794548,-1.64592686760696));
#8185=CARTESIAN_POINT('Ctrl Pts',(97.5500087152771,0.643425160313609,-1.65567407475106));
#8186=CARTESIAN_POINT('Ctrl Pts',(97.5490840624209,0.630608219265672,-1.66059803507056));
#8187=CARTESIAN_POINT('Ctrl Pts',(97.546638934068,0.596752388612501,-1.67315615919371));
#8188=CARTESIAN_POINT('Ctrl Pts',(97.5451103431152,0.575624640443485,-1.68054191847934));
#8189=CARTESIAN_POINT('Ctrl Pts',(97.5367581266179,0.46043481555503,-1.71838255638424));
#8190=CARTESIAN_POINT('Ctrl Pts',(97.5296940642403,0.364109062153793,-1.74133788960204));
#8191=CARTESIAN_POINT('Ctrl Pts',(97.5166888289907,0.18737235502855,-1.76814674305959));
#8192=CARTESIAN_POINT('Ctrl Pts',(97.5108099048211,0.107638023393683,-1.77478598852511));
#8193=CARTESIAN_POINT('Ctrl Pts',(97.5009453103086,-0.0284251646162766,
-1.77691024142284));
#8194=CARTESIAN_POINT('Ctrl Pts',(97.4969232324965,-0.0845942238383299,
-1.77512340432486));
#8195=CARTESIAN_POINT('Ctrl Pts',(97.4921148464802,-0.153559953124779,-1.76964762039276));
#8196=CARTESIAN_POINT('Ctrl Pts',(97.4912170293429,-0.166519331224918,-1.76847524633837));
#8197=CARTESIAN_POINT('Ctrl Pts',(97.4897956201097,-0.187186139931326,-1.76637641526618));
#8198=CARTESIAN_POINT('Ctrl Pts',(97.4892672493625,-0.194902120250317,-1.76554169045786));
#8199=CARTESIAN_POINT('Ctrl Pts',(97.488254441058,-0.209762345949854,-1.76383548381618));
#8200=CARTESIAN_POINT('Ctrl Pts',(97.4877696507699,-0.216907112276236,-1.76297111788326));
#8201=CARTESIAN_POINT('Ctrl Pts',(97.4866869910549,-0.232929453070199,-1.76093387564777));
#8202=CARTESIAN_POINT('Ctrl Pts',(97.4860904219326,-0.24180394109597,-1.75973722668616));
#8203=CARTESIAN_POINT('Ctrl Pts',(97.4839972776029,-0.273085972637487,-1.75527799379606));
#8204=CARTESIAN_POINT('Ctrl Pts',(97.4825191052179,-0.295440827975233,-1.75165396585247));
#8205=CARTESIAN_POINT('Ctrl Pts',(97.4727772573635,-0.443995740595216,-1.72464606865087));
#8206=CARTESIAN_POINT('Ctrl Pts',(97.46505321923,-0.567424474727915,-1.68806801141452));
#8207=CARTESIAN_POINT('Ctrl Pts',(97.451937575724,-0.763672693581614,-1.60592239649487));
#8208=CARTESIAN_POINT('Ctrl Pts',(97.4466757615812,-0.839073408649331,-1.56784444489353));
#8209=CARTESIAN_POINT('Ctrl Pts',(97.4395717900887,-0.933548914404199,-1.51136088335045));
#8210=CARTESIAN_POINT('Ctrl Pts',(97.437896729353,-0.955329522485675,-1.49768844871949));
#8211=CARTESIAN_POINT('Ctrl Pts',(97.4352549778074,-0.988853125566246,-1.47561568557153));
#8212=CARTESIAN_POINT('Ctrl Pts',(97.434300224079,-1.00080404708521,-1.46753650521054));
#8213=CARTESIAN_POINT('Ctrl Pts',(97.4325065027749,-1.02294087606994,-1.45217518680701));
#8214=CARTESIAN_POINT('Ctrl Pts',(97.4316689476699,-1.03315081579598,-1.44492912873749));
#8215=CARTESIAN_POINT('Ctrl Pts',(97.4297808120678,-1.05587907306941,-1.42843469094478));
#8216=CARTESIAN_POINT('Ctrl Pts',(97.4287280341355,-1.06835401452044,-1.41912859035445));
#8217=CARTESIAN_POINT('Ctrl Pts',(97.4260008607048,-1.10015403665477,-1.3947493545123));
#8218=CARTESIAN_POINT('Ctrl Pts',(97.4243172284351,-1.11929178981383,-1.37943845507715));
#8219=CARTESIAN_POINT('Ctrl Pts',(97.414966201394,-1.22284828997991,-1.29301545342972));
#8220=CARTESIAN_POINT('Ctrl Pts',(97.4070025974125,-1.30080083094552,-1.21456030540418));
#8221=CARTESIAN_POINT('Ctrl Pts',(97.3931521974554,-1.42133975248412,-1.06823942455043));
#8222=CARTESIAN_POINT('Ctrl Pts',(97.387334266965,-1.46757267273331,-1.00377960977377));
#8223=CARTESIAN_POINT('Ctrl Pts',(97.3797445969987,-1.52334126397546,-0.91389272769813));
#8224=CARTESIAN_POINT('Ctrl Pts',(97.3778565238841,-1.53682765047578,-0.891027186070993));
#8225=CARTESIAN_POINT('Ctrl Pts',(97.3746524303853,-1.55911624108677,-0.851225232666872));
#8226=CARTESIAN_POINT('Ctrl Pts',(97.3733251762329,-1.56816714668493,-0.834433774077758));
#8227=CARTESIAN_POINT('Ctrl Pts',(97.371394798285,-1.58108448748137,-0.809516369581118));
#8228=CARTESIAN_POINT('Ctrl Pts',(97.3707798040096,-1.58516215472815,-0.801502252769358));
#8229=CARTESIAN_POINT('Ctrl Pts',(97.3696888056598,-1.59233138940458,-0.787143324507735));
#8230=CARTESIAN_POINT('Ctrl Pts',(97.3692114248528,-1.59544619965415,-0.780810665933484));
#8231=CARTESIAN_POINT('Ctrl Pts',(97.3681486391894,-1.60233067676083,-0.766600754156208));
#8232=CARTESIAN_POINT('Ctrl Pts',(97.3675644615615,-1.60608008853077,-0.758714090563911));
#8233=CARTESIAN_POINT('Ctrl Pts',(97.3658058854859,-1.61725503490599,-0.734754167266526));
#8234=CARTESIAN_POINT('Ctrl Pts',(97.3646418645835,-1.62449880927977,-0.718596695903648));
#8235=CARTESIAN_POINT('Ctrl Pts',(97.3548441005699,-1.68401395711633,-0.580344630162377));
#8236=CARTESIAN_POINT('Ctrl Pts',(97.3468508091913,-1.72268794946102,-0.452834486244263));
#8237=CARTESIAN_POINT('Ctrl Pts',(97.3338630160027,-1.76093808214626,-0.245457280220734));
#8238=CARTESIAN_POINT('Ctrl Pts',(97.3290119156321,-1.7700185981609,-0.167882842248317));
#8239=CARTESIAN_POINT('Ctrl Pts',(97.3219751714822,-1.77558103311633,-0.0582032388153459));
#8240=CARTESIAN_POINT('Ctrl Pts',(97.3199147583734,-1.77633845114438,-0.026403202290071));
#8241=CARTESIAN_POINT('Ctrl Pts',(97.3168032564605,-1.77619432741937,0.0210168398053602));
#8242=CARTESIAN_POINT('Ctrl Pts',(97.3157722796422,-1.77594086713687,0.0366334103178855));
#8243=CARTESIAN_POINT('Ctrl Pts',(97.3139029481796,-1.77511315781711,0.0647625144756611));
#8244=CARTESIAN_POINT('Ctrl Pts',(97.3130669502636,-1.77461242710866,0.0772762969659785));
#8245=CARTESIAN_POINT('Ctrl Pts',(97.3112616440601,-1.77325227257266,0.104150800846863));
#8246=CARTESIAN_POINT('Ctrl Pts',(97.3102910679666,-1.77235062903052,0.118508388028271));
#8247=CARTESIAN_POINT('Ctrl Pts',(97.3076293381081,-1.76941664928055,0.157625916758776));
#8248=CARTESIAN_POINT('Ctrl Pts',(97.3059275397609,-1.76703917022971,0.18235588917505));
#8249=CARTESIAN_POINT('Ctrl Pts',(97.2944875463846,-1.74775628799199,0.346671704171294));
#8250=CARTESIAN_POINT('Ctrl Pts',(97.2842387785549,-1.71484836886303,0.483853147740892));
#8251=CARTESIAN_POINT('Ctrl Pts',(97.2695889457956,-1.64538395672542,0.671831720883208));
#8252=CARTESIAN_POINT('Ctrl Pts',(97.2652269375064,-1.62181263006219,0.726891206554976));
#8253=CARTESIAN_POINT('Ctrl Pts',(97.258574357595,-1.58086144958288,0.810587017625067));
#8254=CARTESIAN_POINT('Ctrl Pts',(97.2562243807072,-1.56537732742084,0.840100230408765));
#8255=CARTESIAN_POINT('Ctrl Pts',(97.2531504459254,-1.54364110389789,0.87883976818607));
#8256=CARTESIAN_POINT('Ctrl Pts',(97.2523875043142,-1.53812055206124,0.888466307219416));
#8257=CARTESIAN_POINT('Ctrl Pts',(97.2511283718436,-1.52879356342425,0.904382848350329));
#8258=CARTESIAN_POINT('Ctrl Pts',(97.2506290923629,-1.52503770716857,0.910701979105579));
#8259=CARTESIAN_POINT('Ctrl Pts',(97.2496155028211,-1.51729300760363,0.923549956016718));
#8260=CARTESIAN_POINT('Ctrl Pts',(97.2491014010215,-1.51330103134567,0.930076656133694));
#8261=CARTESIAN_POINT('Ctrl Pts',(97.2477539924649,-1.50267385867069,0.947202030026113));
#8262=CARTESIAN_POINT('Ctrl Pts',(97.2469251046745,-1.4959685661537,0.957757005886478));
#8263=CARTESIAN_POINT('Ctrl Pts',(97.2432177592273,-1.46524950761932,1.00500285444358));
#8264=CARTESIAN_POINT('Ctrl Pts',(97.2404110674975,-1.43999156109458,1.04087071867133));
#8265=CARTESIAN_POINT('Ctrl Pts',(97.2316173425303,-1.35543808043715,1.15196361958598));
#8266=CARTESIAN_POINT('Ctrl Pts',(97.2258050666096,-1.29137734948703,1.22334755089961));
#8267=CARTESIAN_POINT('Ctrl Pts',(97.2144259797327,-1.15721222554527,1.35050363808496));
#8268=CARTESIAN_POINT('Ctrl Pts',(97.2088860335297,-1.08804190118155,1.40682708479119));
#8269=CARTESIAN_POINT('Ctrl Pts',(97.2014432529643,-0.993323652236097,1.47277500882813));
#8270=CARTESIAN_POINT('Ctrl Pts',(97.1997281982726,-0.971372019795175,1.48734474373017));
#8271=CARTESIAN_POINT('Ctrl Pts',(97.197037468463,-0.936802927122869,1.50919719333448));
#8272=CARTESIAN_POINT('Ctrl Pts',(97.1960744872528,-0.924405663805522,1.51682234957224));
#8273=CARTESIAN_POINT('Ctrl Pts',(97.1942733451361,-0.901181239050674,1.53071647515727));
#8274=CARTESIAN_POINT('Ctrl Pts',(97.1934367022838,-0.890378775346953,1.53702510569225));
#8275=CARTESIAN_POINT('Ctrl Pts',(97.1915611397493,-0.866136092175699,1.55084148712438));
#8276=CARTESIAN_POINT('Ctrl Pts',(97.1905201533219,-0.852663226102643,1.5582895896279));
#8277=CARTESIAN_POINT('Ctrl Pts',(97.1878451286312,-0.818007712317258,1.57686394194831));
#8278=CARTESIAN_POINT('Ctrl Pts',(97.1862024419064,-0.796694542136727,1.58773871223062));
#8279=CARTESIAN_POINT('Ctrl Pts',(97.175715937046,-0.660490524407602,1.6538021068581));
#8280=CARTESIAN_POINT('Ctrl Pts',(97.166463225868,-0.540177302808986,1.69691092413055));
#8281=CARTESIAN_POINT('Ctrl Pts',(97.1522132162331,-0.350766428870102,1.74257655893968));
#8282=CARTESIAN_POINT('Ctrl Pts',(97.1472830034468,-0.284369881230242,1.75463524134333));
#8283=CARTESIAN_POINT('Ctrl Pts',(97.1398974533419,-0.181926266547648,1.76727126281748));
#8284=CARTESIAN_POINT('Ctrl Pts',(97.1373685041337,-0.14627965715846,1.77057831064361));
#8285=CARTESIAN_POINT('Ctrl Pts',(97.134102278792,-0.0992036183010982,1.77351404131004));
#8286=CARTESIAN_POINT('Ctrl Pts',(97.1333198709273,-0.0878455342175128,
1.77411290278429));
#8287=CARTESIAN_POINT('Ctrl Pts',(97.1320374642849,-0.0690816861468553,
1.77492159014721));
#8288=CARTESIAN_POINT('Ctrl Pts',(97.131534146549,-0.0616791231231223,1.77519424929974));
#8289=CARTESIAN_POINT('Ctrl Pts',(97.1305834792549,-0.0476203873594082,
1.77562402678054));
#8290=CARTESIAN_POINT('Ctrl Pts',(97.1301356227535,-0.0409646935344745,
1.77579004484116));
#8291=CARTESIAN_POINT('Ctrl Pts',(97.1289339825993,-0.0230240468821298,
1.77613663123154));
#8292=CARTESIAN_POINT('Ctrl Pts',(97.1281839866272,-0.011737821428815,1.77624707729253));
#8293=CARTESIAN_POINT('Ctrl Pts',(97.125130256148,0.0345399038578194,1.77625882609085));
#8294=CARTESIAN_POINT('Ctrl Pts',(97.1228720460036,0.069526154371763,1.77523376429706));
#8295=CARTESIAN_POINT('Ctrl Pts',(97.1165216538083,0.169246905730238,1.76935898348863));
#8296=CARTESIAN_POINT('Ctrl Pts',(97.1125149670027,0.233778716580485,1.7619944382235));
#8297=CARTESIAN_POINT('Ctrl Pts',(97.1004369633245,0.427498358375281,1.72905356259309));
#8298=CARTESIAN_POINT('Ctrl Pts',(97.0924259376233,0.554362751486858,1.69264849389071));
#8299=CARTESIAN_POINT('Ctrl Pts',(97.0822700322195,0.699969124711183,1.63272072156878));
#8300=CARTESIAN_POINT('Ctrl Pts',(97.0805852934568,0.723680343428494,1.62235026416194));
#8301=CARTESIAN_POINT('Ctrl Pts',(97.0779220324908,0.76041003395233,1.6053205562427));
#8302=CARTESIAN_POINT('Ctrl Pts',(97.0769555161355,0.773587780499568,1.59901201761015));
#8303=CARTESIAN_POINT('Ctrl Pts',(97.0751511134287,0.797898684095875,1.58700288557339));
#8304=CARTESIAN_POINT('Ctrl Pts',(97.0743147900584,0.809052416864327,1.58134583246737));
#8305=CARTESIAN_POINT('Ctrl Pts',(97.0724442750668,0.833739543536161,1.56849523935448));
#8306=CARTESIAN_POINT('Ctrl Pts',(97.0714080697921,0.847241306201684,1.56124344215834));
#8307=CARTESIAN_POINT('Ctrl Pts',(97.0683079974663,0.887108737226521,1.53916119616685));
#8308=CARTESIAN_POINT('Ctrl Pts',(97.0662265065759,0.913190054955769,1.5238316270869));
#8309=CARTESIAN_POINT('Ctrl Pts',(97.0562044215072,1.03546571249375,1.44769615303172));
#8310=CARTESIAN_POINT('Ctrl Pts',(97.0479601301718,1.12604724226921,1.37841333940808));
#8311=CARTESIAN_POINT('Ctrl Pts',(97.0323782557359,1.28212577806341,1.23332304985503));
#8312=CARTESIAN_POINT('Ctrl Pts',(97.0250919416703,1.34908743251226,1.15969768673858));
#8313=CARTESIAN_POINT('Ctrl Pts',(97.0168788342668,1.42037881719271,1.06672630988367));
#8314=CARTESIAN_POINT('Ctrl Pts',(97.0156418849221,1.43099943706171,1.05243606747396));
#8315=CARTESIAN_POINT('Ctrl Pts',(97.0138169933292,1.44651778841764,1.03088647885204));
#8316=CARTESIAN_POINT('Ctrl Pts',(97.0132188898722,1.45157926711454,1.02374717773884));
#8317=CARTESIAN_POINT('Ctrl Pts',(97.0121449304965,1.46062657865936,1.01078378399968));
#8318=CARTESIAN_POINT('Ctrl Pts',(97.0116678981872,1.46463066042491,1.00497308068935));
#8319=CARTESIAN_POINT('Ctrl Pts',(97.0105897675122,1.47364630178632,0.991721288962956));
#8320=CARTESIAN_POINT('Ctrl Pts',(97.0099900943235,1.47863623981172,0.984265927850673));
#8321=CARTESIAN_POINT('Ctrl Pts',(97.0081337285318,1.49399686650572,0.960935469534442));
#8322=CARTESIAN_POINT('Ctrl Pts',(97.0068891734624,1.50417036529532,0.944931318520012));
#8323=CARTESIAN_POINT('Ctrl Pts',(97.0039470835018,1.52785504372839,0.906320277871069));
#8324=CARTESIAN_POINT('Ctrl Pts',(97.0022618315973,1.54112385274543,0.883569406638891));
#8325=CARTESIAN_POINT('Ctrl Pts',(96.9956516835887,1.59170198507842,0.792239171381185));
#8326=CARTESIAN_POINT('Ctrl Pts',(96.9908701435527,1.62498086707824,0.721524026948818));
#8327=CARTESIAN_POINT('Ctrl Pts',(96.9792057480504,1.69440022418173,0.544617334105543));
#8328=CARTESIAN_POINT('Ctrl Pts',(96.9723253309013,1.72534918452841,0.436768439586762));
#8329=CARTESIAN_POINT('Ctrl Pts',(96.9635364352556,1.7504446312907,0.302666490877937));
#8330=CARTESIAN_POINT('Ctrl Pts',(96.9619454414689,1.75444970953147,0.278513079530205));
#8331=CARTESIAN_POINT('Ctrl Pts',(96.9593180936436,1.76018117208739,0.238889711297656));
#8332=CARTESIAN_POINT('Ctrl Pts',(96.9582911045482,1.76220574555847,0.223465740910955));
#8333=CARTESIAN_POINT('Ctrl Pts',(96.9564260201053,1.76549357143071,0.195584369913954));
#8334=CARTESIAN_POINT('Ctrl Pts',(96.9555902330909,1.76682819712699,0.183136300473857));
#8335=CARTESIAN_POINT('Ctrl Pts',(96.9537820195819,1.76941772206497,0.156311346428569));
#8336=CARTESIAN_POINT('Ctrl Pts',(96.9528082881519,1.77062921095662,0.141931279292703));
#8337=CARTESIAN_POINT('Ctrl Pts',(96.9500821747846,1.77351357510641,0.101863914718327));
#8338=CARTESIAN_POINT('Ctrl Pts',(96.9483179980546,1.77480341953332,0.0761535232723153));
#8339=CARTESIAN_POINT('Ctrl Pts',(96.9442757851557,1.77646166416109,0.0177647976588811));
#8340=CARTESIAN_POINT('Ctrl Pts',(96.9419887518329,1.77648754821479,-0.0149035008449363));
#8341=CARTESIAN_POINT('Ctrl Pts',(96.9396785508644,1.77561363580749,-0.0475423898693833));
#8342=CARTESIAN_POINT('',(96.9801888256167,-0.00138251417933347,1.77624916100617));
#8343=CARTESIAN_POINT('Ctrl Pts',(96.7921246218182,1.77561363837209,-0.0475422940869062));
#8344=CARTESIAN_POINT('Ctrl Pts',(96.7922437685583,1.77566277130408,-0.0457072731687558));
#8345=CARTESIAN_POINT('Ctrl Pts',(96.7923627957961,1.7757090601137,-0.0438721573609598));
#8346=CARTESIAN_POINT('Ctrl Pts',(96.7943923145719,1.7764505530197,-0.0125495285269162));
#8347=CARTESIAN_POINT('Ctrl Pts',(96.7962722099045,1.77641404750837,0.0169523811319034));
#8348=CARTESIAN_POINT('Ctrl Pts',(96.8042962371452,1.77308574138958,0.144207381436421));
#8349=CARTESIAN_POINT('Ctrl Pts',(96.8102291969789,1.76245856168471,0.241600729689548));
#8350=CARTESIAN_POINT('Ctrl Pts',(96.8221323450874,1.72571382706155,0.431388848441539));
#8351=CARTESIAN_POINT('Ctrl Pts',(96.8280805935747,1.70003152890578,0.523520821034303));
#8352=CARTESIAN_POINT('Ctrl Pts',(96.8357144305895,1.65939582986076,0.634006342816208));
#8353=CARTESIAN_POINT('Ctrl Pts',(96.8371683455194,1.65132886099307,0.654730084574135));
#8354=CARTESIAN_POINT('Ctrl Pts',(96.8395389566912,1.63766687352809,0.687967264574194));
#8355=CARTESIAN_POINT('Ctrl Pts',(96.8404475313342,1.63231219870343,0.700577343294984));
#8356=CARTESIAN_POINT('Ctrl Pts',(96.8422056839233,1.62172756777363,0.72472350822251));
#8357=CARTESIAN_POINT('Ctrl Pts',(96.8430544860503,1.6165190168332,0.736268104208643));
#8358=CARTESIAN_POINT('Ctrl Pts',(96.8450435034146,1.60408831789244,0.76305250186109));
#8359=CARTESIAN_POINT('Ctrl Pts',(96.8461869253768,1.59677180622489,0.778246886761163));
#8360=CARTESIAN_POINT('Ctrl Pts',(96.8500020979588,1.5718059326399,0.828259560446652));
#8361=CARTESIAN_POINT('Ctrl Pts',(96.852705836114,1.55322634147074,0.862597999351462));
#8362=CARTESIAN_POINT('Ctrl Pts',(96.8594521292481,1.5047419045311,0.945553372479553));
#8363=CARTESIAN_POINT('Ctrl Pts',(96.8635332741876,1.47359766824722,0.993392295439538));
#8364=CARTESIAN_POINT('Ctrl Pts',(96.8705574053086,1.41680746957138,1.07206301221505));
#8365=CARTESIAN_POINT('Ctrl Pts',(96.8734732699792,1.39231952950349,1.10367960218034));
#8366=CARTESIAN_POINT('Ctrl Pts',(96.8839312565245,1.30094814819622,1.21376468954196));
#8367=CARTESIAN_POINT('Ctrl Pts',(96.8915029359685,1.22832426597517,1.28721164200949));
#8368=CARTESIAN_POINT('Ctrl Pts',(96.8999669219529,1.13627161330593,1.36538009295072));
#8369=CARTESIAN_POINT('Ctrl Pts',(96.9011938045346,1.12263901421325,1.3766109400705));
#8370=CARTESIAN_POINT('Ctrl Pts',(96.9030068711349,1.10202560449784,1.39308281473312));
#8371=CARTESIAN_POINT('Ctrl Pts',(96.9036030331115,1.09517046134036,1.39847839824765));
#8372=CARTESIAN_POINT('Ctrl Pts',(96.9046750712617,1.08269809366977,1.40814725988875));
#8373=CARTESIAN_POINT('Ctrl Pts',(96.9051521007454,1.07709490636209,1.41243776295829));
#8374=CARTESIAN_POINT('Ctrl Pts',(96.9062321733752,1.06428748731943,1.42212419060212));
#8375=CARTESIAN_POINT('Ctrl Pts',(96.9068337668854,1.05706764996443,1.4274988831171));
#8376=CARTESIAN_POINT('Ctrl Pts',(96.9087025582789,1.03438200029868,1.44412035593852));
#8377=CARTESIAN_POINT('Ctrl Pts',(96.9099573847161,1.01877465662034,1.4551728407666));
#8378=CARTESIAN_POINT('Ctrl Pts',(96.91292866658,0.981009434937713,1.48101111751221));
#8379=CARTESIAN_POINT('Ctrl Pts',(96.9146325083126,0.958691101456287,1.49555506853468));
#8380=CARTESIAN_POINT('Ctrl Pts',(96.9229139142508,0.847481151165387,1.56451302829528));
#8381=CARTESIAN_POINT('Ctrl Pts',(96.9292263006332,0.754241933742447,1.61153574269311));
#8382=CARTESIAN_POINT('Ctrl Pts',(96.9410682152184,0.575638153710478,1.68269222118986));
#8383=CARTESIAN_POINT('Ctrl Pts',(96.9465494071981,0.491564871815255,1.70914417241013));
#8384=CARTESIAN_POINT('Ctrl Pts',(96.9538614853282,0.381286077192493,1.73502834236508));
#8385=CARTESIAN_POINT('Ctrl Pts',(96.9555073811031,0.35656946099771,1.74027599454798));
#8386=CARTESIAN_POINT('Ctrl Pts',(96.9581226318639,0.317527721943207,1.74769842969621));
#8387=CARTESIAN_POINT('Ctrl Pts',(96.9590806950033,0.303272988465862,1.75022830766665));
#8388=CARTESIAN_POINT('Ctrl Pts',(96.9608773366331,0.276641223220803,1.75461970698126));
#8389=CARTESIAN_POINT('Ctrl Pts',(96.961714459652,0.26427228374705,1.75652521436954));
#8390=CARTESIAN_POINT('Ctrl Pts',(96.9633643921041,0.239977636233082,1.76000553399761));
#8391=CARTESIAN_POINT('Ctrl Pts',(96.964176839764,0.228054007247566,1.76159021992694));
#8392=CARTESIAN_POINT('Ctrl Pts',(96.9660239477529,0.201039240146856,1.76490169526194));
#8393=CARTESIAN_POINT('Ctrl Pts',(96.9670608165743,0.185940365010559,1.76655623337296));
#8394=CARTESIAN_POINT('Ctrl Pts',(96.9720524385833,0.113580530829335,1.77354750697522));
#8395=CARTESIAN_POINT('Ctrl Pts',(96.9760859240408,0.0561108169463007,1.77629428175891));
#8396=CARTESIAN_POINT('Ctrl Pts',(96.9801884594846,-0.00138470182539974,
1.77624946026758));
#8397=CARTESIAN_POINT('Ctrl Pts',(96.9801883060489,-0.00138255147987768,
1.77624946194261));
#8398=CARTESIAN_POINT('Ctrl Pts',(96.9888781118596,-0.123167018364227,1.77615467047411));
#8399=CARTESIAN_POINT('Ctrl Pts',(96.9978703122374,-0.244618001788385,1.76353484642063));
#8400=CARTESIAN_POINT('Ctrl Pts',(97.0096401642456,-0.403294066310954,1.73033093233982));
#8401=CARTESIAN_POINT('Ctrl Pts',(97.0125459753947,-0.442486778458538,1.72072574469952));
#8402=CARTESIAN_POINT('Ctrl Pts',(97.0172282731229,-0.506103334100098,1.70281717563903));
#8403=CARTESIAN_POINT('Ctrl Pts',(97.0190323767654,-0.530733068229441,1.6953021845568));
#8404=CARTESIAN_POINT('Ctrl Pts',(97.021506568238,-0.564785934503054,1.68409706251978));
#8405=CARTESIAN_POINT('Ctrl Pts',(97.0221994295379,-0.574352860200603,1.68085837357009));
#8406=CARTESIAN_POINT('Ctrl Pts',(97.0233762264753,-0.590663598176203,1.67518118042147));
#8407=CARTESIAN_POINT('Ctrl Pts',(97.0238624382114,-0.597421114109849,1.67278315795344));
#8408=CARTESIAN_POINT('Ctrl Pts',(97.0248867384612,-0.611699108923349,1.66761880065494));
#8409=CARTESIAN_POINT('Ctrl Pts',(97.0254242396394,-0.619215623776566,1.66484241949637));
#8410=CARTESIAN_POINT('Ctrl Pts',(97.026905113785,-0.639982151907685,1.65701176974645));
#8411=CARTESIAN_POINT('Ctrl Pts',(97.0278423776131,-0.653191150663329,1.65184942168224));
#8412=CARTESIAN_POINT('Ctrl Pts',(97.0345283700719,-0.747756006590991,1.61357976904493));
#8413=CARTESIAN_POINT('Ctrl Pts',(97.0399796584938,-0.826629830325608,1.57463199548102));
#8414=CARTESIAN_POINT('Ctrl Pts',(97.0496472008356,-0.961930678130402,1.49483943245545));
#8415=CARTESIAN_POINT('Ctrl Pts',(97.0538715129715,-1.0194478007896,1.4562216898493));
#8416=CARTESIAN_POINT('Ctrl Pts',(97.0613941257715,-1.11613280631746,1.38276425876093));
#8417=CARTESIAN_POINT('Ctrl Pts',(97.0646604321251,-1.15628620920349,1.34936690664802));
#8418=CARTESIAN_POINT('Ctrl Pts',(97.0696072688698,-1.21370096103492,1.2971657998148));
#8419=CARTESIAN_POINT('Ctrl Pts',(97.071240153233,-1.23212383489966,1.27967960588984));
#8420=CARTESIAN_POINT('Ctrl Pts',(97.0742507054329,-1.26506335087017,1.24704395982025));
#8421=CARTESIAN_POINT('Ctrl Pts',(97.0756230273378,-1.27969875370991,1.23202068102459));
#8422=CARTESIAN_POINT('Ctrl Pts',(97.0770514721577,-1.29452735232963,1.21624974970036));
#8423=CARTESIAN_POINT('Ctrl Pts',(97.0770960959958,-1.2949901852817,1.2157569410033));
#8424=CARTESIAN_POINT('Ctrl Pts',(97.0771851926868,-1.29591347729013,1.21477272581397));
#8425=CARTESIAN_POINT('Ctrl Pts',(97.0772296654398,-1.2963739384717,1.21428132146262));
#8426=CARTESIAN_POINT('Ctrl Pts',(97.0773189916011,-1.29729799520658,1.21329404306859));
#8427=CARTESIAN_POINT('Ctrl Pts',(97.0773638451912,-1.29776158616472,1.21279816490042));
#8428=CARTESIAN_POINT('Ctrl Pts',(97.0774545117024,-1.29869785782136,1.21179553424503));
#8429=CARTESIAN_POINT('Ctrl Pts',(97.0775003251194,-1.29917052643283,1.21128877067853));
#8430=CARTESIAN_POINT('Ctrl Pts',(97.0783710958697,-1.3081463941225,1.2016541500088));
#8431=CARTESIAN_POINT('Ctrl Pts',(97.0792000631972,-1.31655330769046,1.19243744455801));
#8432=CARTESIAN_POINT('Ctrl Pts',(97.080884849684,-1.33335661767487,1.17362124341324));
#8433=CARTESIAN_POINT('Ctrl Pts',(97.0817408050526,-1.34174809092055,1.16401835839392));
#8434=CARTESIAN_POINT('Ctrl Pts',(97.0836346313891,-1.35999131981821,1.14268209929668));
#8435=CARTESIAN_POINT('Ctrl Pts',(97.0846743446301,-1.36979604571571,1.13091004835098));
#8436=CARTESIAN_POINT('Ctrl Pts',(97.0882567343631,-1.40285218236564,1.09016057494093));
#8437=CARTESIAN_POINT('Ctrl Pts',(97.0908289821726,-1.42534474758043,1.06058300888247));
#8438=CARTESIAN_POINT('Ctrl Pts',(97.1025801316417,-1.52252384841471,0.92411361179058));
#8439=CARTESIAN_POINT('Ctrl Pts',(97.1121417022289,-1.58622164205634,0.809911189767498));
#8440=CARTESIAN_POINT('Ctrl Pts',(97.1268676280928,-1.66456113263312,0.624015341245022));
#8441=CARTESIAN_POINT('Ctrl Pts',(97.1320419515988,-1.688293013959,0.556621562040473));
#8442=CARTESIAN_POINT('Ctrl Pts',(97.1382798557681,-1.71274574132034,0.471037620343215));
#8443=CARTESIAN_POINT('Ctrl Pts',(97.1395035918621,-1.71733344477497,0.454026774933829));
#8444=CARTESIAN_POINT('Ctrl Pts',(97.1413129643585,-1.72381133309032,0.428502624925536));
#8445=CARTESIAN_POINT('Ctrl Pts',(97.1419085216915,-1.72589301759252,0.420039654730272));
#8446=CARTESIAN_POINT('Ctrl Pts',(97.1429321472193,-1.72938451851909,0.405380829924952));
#8447=CARTESIAN_POINT('Ctrl Pts',(97.1433618216244,-1.73082346667513,0.399192385694116));
#8448=CARTESIAN_POINT('Ctrl Pts',(97.1443713483996,-1.73414105584454,0.384569273484682));
#8449=CARTESIAN_POINT('Ctrl Pts',(97.1449495970272,-1.73599139291627,0.376128461029571));
#8450=CARTESIAN_POINT('Ctrl Pts',(97.1466360808566,-1.74123765446337,0.351332466613573));
#8451=CARTESIAN_POINT('Ctrl Pts',(97.1477353559214,-1.74446467080607,0.334941984876958));
#8452=CARTESIAN_POINT('Ctrl Pts',(97.1562366591382,-1.7678494486457,0.206643778443689));
#8453=CARTESIAN_POINT('Ctrl Pts',(97.1631620696565,-1.77745305689395,0.0930646441787165));
#8454=CARTESIAN_POINT('Ctrl Pts',(97.1719650990916,-1.77578481163069,-0.0503142245878193));
#8455=CARTESIAN_POINT('Ctrl Pts',(97.1737870088823,-1.77469752648212,-0.0799491757074712));
#8456=CARTESIAN_POINT('Ctrl Pts',(97.1791756440195,-1.76931604337451,-0.167044589364597));
#8457=CARTESIAN_POINT('Ctrl Pts',(97.182765326705,-1.76296786597526,-0.224336213576346));
#8458=CARTESIAN_POINT('Ctrl Pts',(97.1889273187664,-1.74762663853319,-0.320014534657242));
#8459=CARTESIAN_POINT('Ctrl Pts',(97.1914582004671,-1.74012006453733,-0.358594435874066));
#8460=CARTESIAN_POINT('Ctrl Pts',(97.1951352568546,-1.72756346416243,-0.413369483262266));
#8461=CARTESIAN_POINT('Ctrl Pts',(97.1962485782657,-1.72355114409207,-0.42979212814451));
#8462=CARTESIAN_POINT('Ctrl Pts',(97.19820960432,-1.71612243011675,-0.458419486717947));
#8463=CARTESIAN_POINT('Ctrl Pts',(97.1990539469004,-1.71280863784795,-0.47064973898909));
#8464=CARTESIAN_POINT('Ctrl Pts',(97.200818942107,-1.70564502230207,-0.496010411814038));
#8465=CARTESIAN_POINT('Ctrl Pts',(97.2017402443821,-1.70177377224475,-0.509133853307769));
#8466=CARTESIAN_POINT('Ctrl Pts',(97.204166455181,-1.69123798005035,-0.543386593288768));
#8467=CARTESIAN_POINT('Ctrl Pts',(97.2056792521123,-1.6843292329152,-0.564437642741746));
#8468=CARTESIAN_POINT('Ctrl Pts',(97.2135102461873,-1.64685447371526,-0.671802316721369));
#8469=CARTESIAN_POINT('Ctrl Pts',(97.2200321965358,-1.61004561045119,-0.755775409602791));
#8470=CARTESIAN_POINT('Ctrl Pts',(97.2325340341959,-1.52892464780371,-0.907726680286481));
#8471=CARTESIAN_POINT('Ctrl Pts',(97.2384701622505,-1.48610618988684,-0.976251142072641));
#8472=CARTESIAN_POINT('Ctrl Pts',(97.2474109210745,-1.41397264494414,-1.07588781732506));
#8473=CARTESIAN_POINT('Ctrl Pts',(97.2504623162311,-1.38795042163254,-1.10925529229559));
#8474=CARTESIAN_POINT('Ctrl Pts',(97.2553484521581,-1.34366570940094,-1.16203867603485));
#8475=CARTESIAN_POINT('Ctrl Pts',(97.2572136041881,-1.32611467559119,-1.18202854208054));
#8476=CARTESIAN_POINT('Ctrl Pts',(97.2597559673009,-1.301203641617,-1.2091475009338));
#8477=CARTESIAN_POINT('Ctrl Pts',(97.2604575706657,-1.29422199103556,-1.2166174610547));
#8478=CARTESIAN_POINT('Ctrl Pts',(97.2616444642072,-1.28222137046485,-1.22923720861687));
#8479=CARTESIAN_POINT('Ctrl Pts',(97.2621321309166,-1.27723499451919,-1.23441748790563));
#8480=CARTESIAN_POINT('Ctrl Pts',(97.2631542330905,-1.26666422153393,-1.24526668877775));
#8481=CARTESIAN_POINT('Ctrl Pts',(97.2636881355722,-1.26107301145638,-1.25092855202763));
#8482=CARTESIAN_POINT('Ctrl Pts',(97.2651483664758,-1.24559575493238,-1.26639214894037));
#8483=CARTESIAN_POINT('Ctrl Pts',(97.2660688617533,-1.23563199304419,-1.27611577341478));
#8484=CARTESIAN_POINT('Ctrl Pts',(97.2716269416035,-1.17428053351596,-1.33459620959885));
#8485=CARTESIAN_POINT('Ctrl Pts',(97.2760727785378,-1.12012235394852,-1.38036593561045));
#8486=CARTESIAN_POINT('Ctrl Pts',(97.2873208262136,-0.974572906350596,-1.48914765574475));
#8487=CARTESIAN_POINT('Ctrl Pts',(97.2940236613079,-0.879761440665309,-1.54705296543348));
#8488=CARTESIAN_POINT('Ctrl Pts',(97.3034050939055,-0.745253040993197,-1.61281514062893));
#8489=CARTESIAN_POINT('Ctrl Pts',(97.3058657814968,-0.709785986780823,-1.62873519338897));
#8490=CARTESIAN_POINT('Ctrl Pts',(97.3102654868022,-0.646408509465607,-1.65471999003766));
#8491=CARTESIAN_POINT('Ctrl Pts',(97.3121887995141,-0.618714421747461,-1.66527310285286));
#8492=CARTESIAN_POINT('Ctrl Pts',(97.3151337692743,-0.576429123368358,-1.68018593816973));
#8493=CARTESIAN_POINT('Ctrl Pts',(97.3161384504943,-0.56202370540974,-1.68505924275226));
#8494=CARTESIAN_POINT('Ctrl Pts',(97.3178994086071,-0.536822030139404,-1.69322577682258));
#8495=CARTESIAN_POINT('Ctrl Pts',(97.3186528952439,-0.526053510895679,-1.69660222707012));
#8496=CARTESIAN_POINT('Ctrl Pts',(97.320365299605,-0.501619438624628,-1.70400850216787));
#8497=CARTESIAN_POINT('Ctrl Pts',(97.321326168154,-0.487936249435783,-1.70797694144979));
#8498=CARTESIAN_POINT('Ctrl Pts',(97.3239343656804,-0.45087785510985,-1.71824306951903));
#8499=CARTESIAN_POINT('Ctrl Pts',(97.3255916367632,-0.427419947876987,-1.7242279934651));
#8500=CARTESIAN_POINT('Ctrl Pts',(97.3373022631047,-0.262357853849691,-1.76276576962774));
#8501=CARTESIAN_POINT('Ctrl Pts',(97.3479074822279,-0.117373005340089,-1.77830885307717));
#8502=CARTESIAN_POINT('Ctrl Pts',(97.3627151341032,0.0852418244054738,-1.77513171131178));
#8503=CARTESIAN_POINT('Ctrl Pts',(97.3668934723986,0.142560325561041,-1.77145027518955));
#8504=CARTESIAN_POINT('Ctrl Pts',(97.3733052064261,0.231865169953898,-1.76135083838498));
#8505=CARTESIAN_POINT('Ctrl Pts',(97.3755935924289,0.264023904640286,-1.75681812560288));
#8506=CARTESIAN_POINT('Ctrl Pts',(97.3786008775865,0.306884651916257,-1.74957331436839));
#8507=CARTESIAN_POINT('Ctrl Pts',(97.3793567387839,0.317709837809064,-1.74763996476218));
#8508=CARTESIAN_POINT('Ctrl Pts',(97.3806074259483,0.335720762319991,-1.74425037442664));
#8509=CARTESIAN_POINT('Ctrl Pts',(97.3811052574871,0.342916576746842,-1.74284997277102));
#8510=CARTESIAN_POINT('Ctrl Pts',(97.3821192954709,0.357632504092766,-1.73989138378944));
#8511=CARTESIAN_POINT('Ctrl Pts',(97.3826352604509,0.365151520437643,-1.73832891252584));
#8512=CARTESIAN_POINT('Ctrl Pts',(97.3839933204874,0.385016872022323,-1.73406625726528));
#8513=CARTESIAN_POINT('Ctrl Pts',(97.3848308694473,0.397345189167589,-1.73128293460842));
#8514=CARTESIAN_POINT('Ctrl Pts',(97.3885834959496,0.452867912009762,-1.71812340914117));
#8515=CARTESIAN_POINT('Ctrl Pts',(97.391425062721,0.495697129025543,-1.70625978845645));
#8516=CARTESIAN_POINT('Ctrl Pts',(97.4026489644181,0.665622795597073,-1.65225061430707));
#8517=CARTESIAN_POINT('Ctrl Pts',(97.4106630685918,0.788216230640514,-1.59740565909893));
#8518=CARTESIAN_POINT('Ctrl Pts',(97.4229383930489,0.957407710078322,-1.49744998751428));
#8519=CARTESIAN_POINT('Ctrl Pts',(97.4269119345481,1.00959894993034,-1.4627695270249));
#8520=CARTESIAN_POINT('Ctrl Pts',(97.4322776110068,1.07575223229045,-1.41358199429229));
#8521=CARTESIAN_POINT('Ctrl Pts',(97.4335773439042,1.09145831242276,-1.40149049955702));
#8522=CARTESIAN_POINT('Ctrl Pts',(97.4357598612371,1.11728101885328,-1.38091325260486));
#8523=CARTESIAN_POINT('Ctrl Pts',(97.4366368308502,1.12751151318121,-1.37257278785242));
#8524=CARTESIAN_POINT('Ctrl Pts',(97.4383719095569,1.14746096314669,-1.35593535014906));
#8525=CARTESIAN_POINT('Ctrl Pts',(97.4392296757877,1.15718522786088,-1.34764597329514));
#8526=CARTESIAN_POINT('Ctrl Pts',(97.441132413044,1.17844747446322,-1.32912131747619));
#8527=CARTESIAN_POINT('Ctrl Pts',(97.4421792919348,1.18994317513302,-1.31883931559493));
#8528=CARTESIAN_POINT('Ctrl Pts',(97.4452915682999,1.22351445935931,-1.28801616653578));
#8529=CARTESIAN_POINT('Ctrl Pts',(97.447374251714,1.24520156455222,-1.26706201476719));
#8530=CARTESIAN_POINT('Ctrl Pts',(97.4589226506963,1.36118556753658,-1.14914334412415));
#8531=CARTESIAN_POINT('Ctrl Pts',(97.4688289373423,1.44469092034567,-1.04221556110278));
#8532=CARTESIAN_POINT('Ctrl Pts',(97.4840305025927,1.55331995211775,-0.864630232680956));
#8533=CARTESIAN_POINT('Ctrl Pts',(97.4893244391102,1.58752763775887,-0.800091461380455));
#8534=CARTESIAN_POINT('Ctrl Pts',(97.4956875000583,1.62501741712128,-0.717425181961458));
#8535=CARTESIAN_POINT('Ctrl Pts',(97.4969234379416,1.63212104036389,-0.70111444685532));
#8536=CARTESIAN_POINT('Ctrl Pts',(97.4987471300399,1.64235095052128,-0.676626890032803));
#8537=CARTESIAN_POINT('Ctrl Pts',(97.4993450271165,1.64566355765598,-0.668529772071085));
#8538=CARTESIAN_POINT('Ctrl Pts',(97.5003711068295,1.65127908927038,-0.654508837426563));
#8539=CARTESIAN_POINT('Ctrl Pts',(97.5008009218634,1.65361018774981,-0.648596792651734));
#8540=CARTESIAN_POINT('Ctrl Pts',(97.5018085270933,1.6590246788308,-0.634645808050767));
#8541=CARTESIAN_POINT('Ctrl Pts',(97.5023847395692,1.6620814147094,-0.626596812349615));
#8542=CARTESIAN_POINT('Ctrl Pts',(97.5040594036382,1.67084406726151,-0.603007632693148));
#8543=CARTESIAN_POINT('Ctrl Pts',(97.5051490821601,1.67639158786321,-0.58740905220074));
#8544=CARTESIAN_POINT('Ctrl Pts',(97.5137502702867,1.71884952684422,-0.462521744043253));
#8545=CARTESIAN_POINT('Ctrl Pts',(97.5207697033183,1.74525699913278,-0.349936298998502));
#8546=CARTESIAN_POINT('Ctrl Pts',(97.5317197955851,1.76890942707055,-0.173168709070312));
#8547=CARTESIAN_POINT('Ctrl Pts',(97.5355920537966,1.77393052506702,-0.110403668282001));
#8548=CARTESIAN_POINT('Ctrl Pts',(97.5395353031289,1.77561364475627,-0.0475420556493824));
#8549=CARTESIAN_POINT('Origin',(88.3562164250559,0.,0.));
#8550=CARTESIAN_POINT('',(98.436744300164,1.7756136383717,-0.047542294101169));
#8551=CARTESIAN_POINT('',(98.2893138640945,1.77561363880419,-0.0475422779488097));
#8552=CARTESIAN_POINT('',(88.3562164250559,1.77561363837197,-0.0475422940912398));
#8553=CARTESIAN_POINT('',(97.8793796642132,0.00163535216639757,1.77624916181758));
#8554=CARTESIAN_POINT('Ctrl Pts',(98.436744300164,1.7756136383717,-0.047542294101169));
#8555=CARTESIAN_POINT('Ctrl Pts',(98.4364498240271,1.77549319424063,-0.0520406517400838));
#8556=CARTESIAN_POINT('Ctrl Pts',(98.4361561234276,1.77535565357106,-0.0565386361140695));
#8557=CARTESIAN_POINT('Ctrl Pts',(98.4311977724099,1.77273844685076,-0.132658575839666));
#8558=CARTESIAN_POINT('Ctrl Pts',(98.4267239300063,1.76594329645432,-0.20407454630018));
#8559=CARTESIAN_POINT('Ctrl Pts',(98.4141953155081,1.73453508085451,-0.404578135937726));
#8560=CARTESIAN_POINT('Ctrl Pts',(98.4062659760535,1.69990889600267,-0.531604606724482));
#8561=CARTESIAN_POINT('Ctrl Pts',(98.3955350445561,1.63793764026522,-0.688188708671686));
#8562=CARTESIAN_POINT('Ctrl Pts',(98.3931391781615,1.62319149197298,-0.722282827827224));
#8563=CARTESIAN_POINT('Ctrl Pts',(98.3896351500677,1.60041890180874,-0.770708521507362));
#8564=CARTESIAN_POINT('Ctrl Pts',(98.3885560132639,1.59324495485693,-0.785431582274868));
#8565=CARTESIAN_POINT('Ctrl Pts',(98.3866316427076,1.58017679376829,-0.811335351670994));
#8566=CARTESIAN_POINT('Ctrl Pts',(98.3857893296536,1.57436483616474,-0.822556442399754));
#8567=CARTESIAN_POINT('Ctrl Pts',(98.3840189450417,1.56196142527674,-0.845890488638317));
#8568=CARTESIAN_POINT('Ctrl Pts',(98.3830901233183,1.55534767344118,-0.857990564550234));
#8569=CARTESIAN_POINT('Ctrl Pts',(98.3806213227468,1.53749338176221,-0.889770635239372));
#8570=CARTESIAN_POINT('Ctrl Pts',(98.379072940221,1.52601623550939,-0.909314053726346));
#8571=CARTESIAN_POINT('Ctrl Pts',(98.3756282868196,1.49988411870613,-0.951923445489135));
#8572=CARTESIAN_POINT('Ctrl Pts',(98.3737264128007,1.48506464933855,-0.974881256111815));
#8573=CARTESIAN_POINT('Ctrl Pts',(98.3676896827283,1.43681408146994,-1.04597483981874));
#8574=CARTESIAN_POINT('Ctrl Pts',(98.363493518691,1.4015295071744,-1.09280007310644));
#8575=CARTESIAN_POINT('Ctrl Pts',(98.3510962686073,1.29193994017567,-1.22417728151325));
#8576=CARTESIAN_POINT('Ctrl Pts',(98.3427739988167,1.21183999426396,-1.30351922822059));
#8577=CARTESIAN_POINT('Ctrl Pts',(98.3319802823211,1.09535447533574,-1.39882365770442));
#8578=CARTESIAN_POINT('Ctrl Pts',(98.329287957368,1.0651661475218,-1.42194606282038));
#8579=CARTESIAN_POINT('Ctrl Pts',(98.3258215630699,1.02452613141695,-1.45105255546659));
#8580=CARTESIAN_POINT('Ctrl Pts',(98.3249972334819,1.01472508825768,-1.45792329280199));
#8581=CARTESIAN_POINT('Ctrl Pts',(98.3236643845982,0.998642196679764,-1.46895697412623));
#8582=CARTESIAN_POINT('Ctrl Pts',(98.3231520380507,0.992402177815162,-1.47317980968612));
#8583=CARTESIAN_POINT('Ctrl Pts',(98.3221389492554,0.979944398176783,-1.48149534039439));
#8584=CARTESIAN_POINT('Ctrl Pts',(98.3216381612921,0.973727428107289,-1.48558889579128));
#8585=CARTESIAN_POINT('Ctrl Pts',(98.3203670385265,0.957802482630964,-1.49593173566324));
#8586=CARTESIAN_POINT('Ctrl Pts',(98.319600249639,0.948058781504405,-1.50212579962672));
#8587=CARTESIAN_POINT('Ctrl Pts',(98.3163710769934,0.906478407406836,-1.52799263392985));
#8588=CARTESIAN_POINT('Ctrl Pts',(98.313961045111,0.874082307631577,-1.54675310553334));
#8589=CARTESIAN_POINT('Ctrl Pts',(98.3069674180164,0.776938001593733,-1.59898111633273));
#8590=CARTESIAN_POINT('Ctrl Pts',(98.3024911482823,0.7106941327705,-1.62950561828538));
#8591=CARTESIAN_POINT('Ctrl Pts',(98.2906967785278,0.53158988904329,-1.69902819980099));
#8592=CARTESIAN_POINT('Ctrl Pts',(98.2833946947551,0.416371093931519,-1.73087140908704));
#8593=CARTESIAN_POINT('Ctrl Pts',(98.2741449514429,0.274865870806526,-1.75502255525102));
#8594=CARTESIAN_POINT('Ctrl Pts',(98.2725643259572,0.250814224237256,-1.75862092273437));
#8595=CARTESIAN_POINT('Ctrl Pts',(98.2699505545576,0.211315506337741,-1.76370358420352));
#8596=CARTESIAN_POINT('Ctrl Pts',(98.2689266055335,0.195908989197235,-1.76548129942933));
#8597=CARTESIAN_POINT('Ctrl Pts',(98.267064742168,0.168030104502262,-1.76832875981146));
#8598=CARTESIAN_POINT('Ctrl Pts',(98.2662290992367,0.155565829647346,-1.76946884054118));
#8599=CARTESIAN_POINT('Ctrl Pts',(98.2644185886328,0.128671633307802,-1.77164244253615));
#8600=CARTESIAN_POINT('Ctrl Pts',(98.2634423871007,0.114239137391958,-1.77263158363403));
#8601=CARTESIAN_POINT('Ctrl Pts',(98.2607019125536,0.073924309156453,-1.77490020865661));
#8602=CARTESIAN_POINT('Ctrl Pts',(98.2589256410564,0.0480245868690461,-1.77578970311681));
#8603=CARTESIAN_POINT('Ctrl Pts',(98.2511907568331,-0.0637156155086965,
-1.7771810714908));
#8604=CARTESIAN_POINT('Ctrl Pts',(98.2450630746089,-0.149499456208484,-1.77202663779861));
#8605=CARTESIAN_POINT('Ctrl Pts',(98.2289914100532,-0.368907542626103,-1.74279653295528));
#8606=CARTESIAN_POINT('Ctrl Pts',(98.2189210969748,-0.500763045706761,-1.70958225491674));
#8607=CARTESIAN_POINT('Ctrl Pts',(98.2082251164003,-0.643639316351112,-1.65562310180338));
#8608=CARTESIAN_POINT('Ctrl Pts',(98.2070319525122,-0.65962883413529,-1.64931782283778));
#8609=CARTESIAN_POINT('Ctrl Pts',(98.2052585137159,-0.68350734298818,-1.63949878495326));
#8610=CARTESIAN_POINT('Ctrl Pts',(98.2046688648038,-0.691465830415999,-1.63615817297545));
#8611=CARTESIAN_POINT('Ctrl Pts',(98.2036511370002,-0.705240822678005,-1.6302575935744));
#8612=CARTESIAN_POINT('Ctrl Pts',(98.2032215203264,-0.711068238444655,-1.62772430183764));
#8613=CARTESIAN_POINT('Ctrl Pts',(98.2022064439018,-0.724866180770959,-1.6216378230353));
#8614=CARTESIAN_POINT('Ctrl Pts',(98.2016226562061,-0.73282426998406,-1.61805710853004));
#8615=CARTESIAN_POINT('Ctrl Pts',(98.199866499607,-0.756819732126975,-1.60704708427951));
#8616=CARTESIAN_POINT('Ctrl Pts',(98.1987044664364,-0.772773454218721,-1.59943667729234));
#8617=CARTESIAN_POINT('Ctrl Pts',(98.1928732159986,-0.853038453770335,-1.55966641513358));
#8618=CARTESIAN_POINT('Ctrl Pts',(98.1883853476541,-0.915474885686514,-1.52385758172097));
#8619=CARTESIAN_POINT('Ctrl Pts',(98.1757991777122,-1.08586835669961,-1.41186879055));
#8620=CARTESIAN_POINT('Ctrl Pts',(98.1678264465526,-1.18773237498556,-1.32731819330471));
#8621=CARTESIAN_POINT('Ctrl Pts',(98.1570861781658,-1.30458340611965,-1.20600805754049));
#8622=CARTESIAN_POINT('Ctrl Pts',(98.154733024162,-1.32906049843106,-1.17897887864473));
#8623=CARTESIAN_POINT('Ctrl Pts',(98.1512801076867,-1.3632290539861,-1.13883061183677));
#8624=CARTESIAN_POINT('Ctrl Pts',(98.1502081643678,-1.37359980289895,-1.12630021236477));
#8625=CARTESIAN_POINT('Ctrl Pts',(98.1482919914552,-1.39170965169996,-1.103796902547));
#8626=CARTESIAN_POINT('Ctrl Pts',(98.1474505962984,-1.39951736511529,-1.09388047214783));
#8627=CARTESIAN_POINT('Ctrl Pts',(98.1456773516888,-1.41566632264314,-1.07291406148234));
#8628=CARTESIAN_POINT('Ctrl Pts',(98.1447447018772,-1.42398534729773,-1.06184812104333));
#8629=CARTESIAN_POINT('Ctrl Pts',(98.1422541599318,-1.44573328471294,-1.03220385063352));
#8630=CARTESIAN_POINT('Ctrl Pts',(98.140687596042,-1.45893296429981,-1.01346141497995));
#8631=CARTESIAN_POINT('Ctrl Pts',(98.1309863637115,-1.53771799886348,-0.896863459877092));
#8632=CARTESIAN_POINT('Ctrl Pts',(98.122500698521,-1.59378544509857,-0.792956095033334));
#8633=CARTESIAN_POINT('Ctrl Pts',(98.1059342027565,-1.6811430969999,-0.583697823282789));
#8634=CARTESIAN_POINT('Ctrl Pts',(98.0979117060398,-1.71378990472506,-0.479450878684006));
#8635=CARTESIAN_POINT('Ctrl Pts',(98.0890734513185,-1.74028131645104,-0.356062133078072));
#8636=CARTESIAN_POINT('Ctrl Pts',(98.0878805388098,-1.74364440909747,-0.339210159587333));
#8637=CARTESIAN_POINT('Ctrl Pts',(98.0861073964421,-1.74832856695896,-0.313824415211005));
#8638=CARTESIAN_POINT('Ctrl Pts',(98.0855177970025,-1.74983272494863,-0.305326029302561));
#8639=CARTESIAN_POINT('Ctrl Pts',(98.0845001171586,-1.75233674593911,-0.290551834537751));
#8640=CARTESIAN_POINT('Ctrl Pts',(98.0840704995541,-1.7533649310515,-0.284281306837281));
#8641=CARTESIAN_POINT('Ctrl Pts',(98.0830553743316,-1.75572536987176,-0.269385685262963));
#8642=CARTESIAN_POINT('Ctrl Pts',(98.0824715393429,-1.7570277377871,-0.260756128408594));
#8643=CARTESIAN_POINT('Ctrl Pts',(98.0807150889001,-1.76077564968997,-0.234618163303082));
#8644=CARTESIAN_POINT('Ctrl Pts',(98.0795528142587,-1.76302355799085,-0.217081927580092));
#8645=CARTESIAN_POINT('Ctrl Pts',(98.0737190971453,-1.7730895312314,-0.128032963612148));
#8646=CARTESIAN_POINT('Ctrl Pts',(98.0692291743233,-1.77682072677008,-0.0561186120152204));
#8647=CARTESIAN_POINT('Ctrl Pts',(98.0566345562477,-1.77500221966316,0.147913529084895));
#8648=CARTESIAN_POINT('Ctrl Pts',(98.0486554499844,-1.75909658494166,0.279443545136796));
#8649=CARTESIAN_POINT('Ctrl Pts',(98.0379432557986,-1.72051310657633,0.442930355753527));
#8650=CARTESIAN_POINT('Ctrl Pts',(98.035626539613,-1.7112111265038,0.477607422824908));
#8651=CARTESIAN_POINT('Ctrl Pts',(98.0322015786947,-1.69613361538493,0.527697198407684));
#8652=CARTESIAN_POINT('Ctrl Pts',(98.0311199289867,-1.69118414416974,0.543350471583162));
#8653=CARTESIAN_POINT('Ctrl Pts',(98.0291926836041,-1.6820403441575,0.57093272406222));
#8654=CARTESIAN_POINT('Ctrl Pts',(98.0283500388017,-1.67793422260694,0.582889891159723));
#8655=CARTESIAN_POINT('Ctrl Pts',(98.0265805996596,-1.66908947021142,0.60777795701333));
#8656=CARTESIAN_POINT('Ctrl Pts',(98.0256530723141,-1.66432741053121,0.62069957028101));
#8657=CARTESIAN_POINT('Ctrl Pts',(98.0231916245013,-1.65136338049467,0.654654637687382));
#8658=CARTESIAN_POINT('Ctrl Pts',(98.0216493903083,-1.6429100585522,0.675588755524796));
#8659=CARTESIAN_POINT('Ctrl Pts',(98.0118529852273,-1.58717381741344,0.806378868563877));
#8660=CARTESIAN_POINT('Ctrl Pts',(98.0032349843248,-1.52930368236859,0.911366073932465));
#8661=CARTESIAN_POINT('Ctrl Pts',(97.9866284126233,-1.40010641559389,1.09834854595397));
#8662=CARTESIAN_POINT('Ctrl Pts',(97.9787037845345,-1.3309331086271,1.18122319923876));
#8663=CARTESIAN_POINT('Ctrl Pts',(97.9699474030927,-1.24244254822381,1.26952709552912));
#8664=CARTESIAN_POINT('Ctrl Pts',(97.968747840813,-1.23003552466186,1.28155187002866));
#8665=CARTESIAN_POINT('Ctrl Pts',(97.9669668709888,-1.21115693202138,1.29932203324005));
#8666=CARTESIAN_POINT('Ctrl Pts',(97.9663759760926,-1.20481602133872,1.30520390079967));
#8667=CARTESIAN_POINT('Ctrl Pts',(97.9653570469639,-1.19374275718619,1.31532606570448));
#8668=CARTESIAN_POINT('Ctrl Pts',(97.9649274601845,-1.18903037412981,1.31958751208561));
#8669=CARTESIAN_POINT('Ctrl Pts',(97.9639136364093,-1.17780528126715,1.32962949883111));
#8670=CARTESIAN_POINT('Ctrl Pts',(97.9633310568957,-1.17127281032193,1.33538754543905));
#8671=CARTESIAN_POINT('Ctrl Pts',(97.9617106378978,-1.15288177893972,1.35135953820233));
#8672=CARTESIAN_POINT('Ctrl Pts',(97.960680202148,-1.14092986342967,1.36146541832615));
#8673=CARTESIAN_POINT('Ctrl Pts',(97.9568232330882,-1.09529295588967,1.39903035090943));
#8674=CARTESIAN_POINT('Ctrl Pts',(97.9540592012098,-1.06073540648793,1.42540997514884));
#8675=CARTESIAN_POINT('Ctrl Pts',(97.9430159046634,-0.916900363792435,1.52707563437461));
#8676=CARTESIAN_POINT('Ctrl Pts',(97.9350664257595,-0.800318623036185,1.59127598507827));
#8677=CARTESIAN_POINT('Ctrl Pts',(97.9231224735167,-0.623983897376875,1.66405570736381));
#8678=CARTESIAN_POINT('Ctrl Pts',(97.9194302741321,-0.569247678466713,1.68356566639224));
#8679=CARTESIAN_POINT('Ctrl Pts',(97.9143575918865,-0.494637045618368,1.70610464833716));
#8680=CARTESIAN_POINT('Ctrl Pts',(97.913054707576,-0.475521620471654,1.71153089785536));
#8681=CARTESIAN_POINT('Ctrl Pts',(97.9109555654397,-0.444828751366333,1.71968974503466));
#8682=CARTESIAN_POINT('Ctrl Pts',(97.9101660200869,-0.433307562692562,1.72262879972795));
#8683=CARTESIAN_POINT('Ctrl Pts',(97.9085229511075,-0.409386056290628,1.72847601339143));
#8684=CARTESIAN_POINT('Ctrl Pts',(97.9076689232356,-0.39698226407884,1.73136689910523));
#8685=CARTESIAN_POINT('Ctrl Pts',(97.9059646715361,-0.372295530630285,1.73684127784819));
#8686=CARTESIAN_POINT('Ctrl Pts',(97.905114621494,-0.360014158679006,1.7394284630239));
#8687=CARTESIAN_POINT('Ctrl Pts',(97.9031159236725,-0.331217087005892,1.74517679465249));
#8688=CARTESIAN_POINT('Ctrl Pts',(97.9019640602107,-0.314682107919662,1.74823394900781));
#8689=CARTESIAN_POINT('Ctrl Pts',(97.8938788046602,-0.199066246213916,1.76791685285348));
#8690=CARTESIAN_POINT('Ctrl Pts',(97.8866915543347,-0.0987931240126965,
1.77634175479645));
#8691=CARTESIAN_POINT('Ctrl Pts',(97.8793797538287,0.00163615522257698,
1.7762492464449));
#8692=CARTESIAN_POINT('Ctrl Pts',(97.8793798115091,0.00163536296821643,
1.7762492471745));
#8693=CARTESIAN_POINT('Ctrl Pts',(97.8701489465145,0.12842344781845,1.77613251550573));
#8694=CARTESIAN_POINT('Ctrl Pts',(97.8607566791393,0.254844257215121,1.76244136402429));
#8695=CARTESIAN_POINT('Ctrl Pts',(97.8510352112,0.390526460359617,1.73282968049199));
#8696=CARTESIAN_POINT('Ctrl Pts',(97.8501958426688,0.402287510813218,1.73013710295976));
#8697=CARTESIAN_POINT('Ctrl Pts',(97.8486422596125,0.424157922583311,1.72489500807164));
#8698=CARTESIAN_POINT('Ctrl Pts',(97.8479265771266,0.434273992030345,1.72237593032756));
#8699=CARTESIAN_POINT('Ctrl Pts',(97.8467232858721,0.45136187029056,1.717960625396));
#8700=CARTESIAN_POINT('Ctrl Pts',(97.8462331385813,0.458345256861603,1.7161106845584));
#8701=CARTESIAN_POINT('Ctrl Pts',(97.8452139353772,0.472917549871457,1.71215509540286));
#8702=CARTESIAN_POINT('Ctrl Pts',(97.8446853299995,0.480504008581517,1.71004151512806));
#8703=CARTESIAN_POINT('Ctrl Pts',(97.8432554246691,0.501094868121651,1.70415706999478));
#8704=CARTESIAN_POINT('Ctrl Pts',(97.842359562017,0.514070918531787,1.70028777103803));
#8705=CARTESIAN_POINT('Ctrl Pts',(97.8375287995418,0.58436235787695,1.67844943302586));
#8706=CARTESIAN_POINT('Ctrl Pts',(97.8337307943092,0.640788414818756,1.65772845892284));
#8707=CARTESIAN_POINT('Ctrl Pts',(97.8239836348431,0.784851380338988,1.59636659444337));
#8708=CARTESIAN_POINT('Ctrl Pts',(97.8181365185447,0.870412805256262,1.55137374007192));
#8709=CARTESIAN_POINT('Ctrl Pts',(97.8072521675063,1.01883580541849,1.45716290885644));
#8710=CARTESIAN_POINT('Ctrl Pts',(97.802270518153,1.08284705075691,1.41024472440532));
#8711=CARTESIAN_POINT('Ctrl Pts',(97.7957629469704,1.15954461491003,1.34571900645595));
#8712=CARTESIAN_POINT('Ctrl Pts',(97.7943914964367,1.1753423755258,1.33194354159338));
#8713=CARTESIAN_POINT('Ctrl Pts',(97.7929663866391,1.19136624139158,1.31746383238738));
#8714=CARTESIAN_POINT('Ctrl Pts',(97.7929242128531,1.19184009107077,1.31703518103769));
#8715=CARTESIAN_POINT('Ctrl Pts',(97.7928395981406,1.19279008854765,1.31617486688233));
#8716=CARTESIAN_POINT('Ctrl Pts',(97.7927971570968,1.19326623356079,1.31574320115745));
#8717=CARTESIAN_POINT('Ctrl Pts',(97.7927115203567,1.1942262738616,1.31487189366832));
#8718=CARTESIAN_POINT('Ctrl Pts',(97.7926683242941,1.19471016088888,1.31443224298828));
#8719=CARTESIAN_POINT('Ctrl Pts',(97.7925806329629,1.19569174266412,1.31353940637621));
#8720=CARTESIAN_POINT('Ctrl Pts',(97.7925361370363,1.19618942272962,1.31308620452962));
#8721=CARTESIAN_POINT('Ctrl Pts',(97.7924452117151,1.19720561175954,1.31215977627235));
#8722=CARTESIAN_POINT('Ctrl Pts',(97.792398781297,1.19772409798665,1.31168652520156));
#8723=CARTESIAN_POINT('Ctrl Pts',(97.7923032176292,1.1987903794802,1.31071211172024));
#8724=CARTESIAN_POINT('Ctrl Pts',(97.7922540828689,1.19933814127114,1.31021091303418));
#8725=CARTESIAN_POINT('Ctrl Pts',(97.7921521396999,1.20047363373767,1.30917063564497));
#8726=CARTESIAN_POINT('Ctrl Pts',(97.7920993290948,1.2010613158117,1.30863150435542));
#8727=CARTESIAN_POINT('Ctrl Pts',(97.7919887602823,1.20229058906726,1.30750226072982));
#8728=CARTESIAN_POINT('Ctrl Pts',(97.7919309988614,1.20293210918085,1.30691207166756));
#8729=CARTESIAN_POINT('Ctrl Pts',(97.79180878787,1.20428804298039,1.30566278832957));
#8730=CARTESIAN_POINT('Ctrl Pts',(97.7917443334925,1.20500235040018,1.30500357961876));
#8731=CARTESIAN_POINT('Ctrl Pts',(97.7916062525742,1.20653086621023,1.30359064219827));
#8732=CARTESIAN_POINT('Ctrl Pts',(97.7915326185799,1.20734490983612,1.30283673659758));
#8733=CARTESIAN_POINT('Ctrl Pts',(97.7914017433997,1.20878987833227,1.30149599883434));
#8734=CARTESIAN_POINT('Ctrl Pts',(97.7913445150267,1.20942108419775,1.30090946880782));
#8735=CARTESIAN_POINT('Ctrl Pts',(97.7911442978448,1.21162715143311,1.29885655054649));
#8736=CARTESIAN_POINT('Ctrl Pts',(97.7910012072874,1.21319976965839,1.29738776463275));
#8737=CARTESIAN_POINT('Ctrl Pts',(97.7900254248622,1.22389661059604,1.28736072812023));
#8738=CARTESIAN_POINT('Ctrl Pts',(97.7891887641735,1.23293266851325,1.27870934102654));
#8739=CARTESIAN_POINT('Ctrl Pts',(97.7873129321521,1.25288548084041,1.2591978131394));
#8740=CARTESIAN_POINT('Ctrl Pts',(97.78627169125,1.26375379960836,1.24828981755339));
#8741=CARTESIAN_POINT('Ctrl Pts',(97.7835955445836,1.29115283437915,1.22006617252224));
#8742=CARTESIAN_POINT('Ctrl Pts',(97.7819519778819,1.3074773577559,1.20255559905682));
#8743=CARTESIAN_POINT('Ctrl Pts',(97.7696475394835,1.42594619136729,1.07021503337505));
#8744=CARTESIAN_POINT('Ctrl Pts',(97.758366896901,1.51313959683016,0.942906875832111));
#8745=CARTESIAN_POINT('Ctrl Pts',(97.7435743829219,1.60519890862316,0.762119559965586));
#8746=CARTESIAN_POINT('Ctrl Pts',(97.7400051867513,1.62571403238309,0.717317390210057));
#8747=CARTESIAN_POINT('Ctrl Pts',(97.7350692557899,1.65195559844421,0.653078976351917));
#8748=CARTESIAN_POINT('Ctrl Pts',(97.7336484304696,1.65925256249553,0.634311008894522));
#8749=CARTESIAN_POINT('Ctrl Pts',(97.7311604808452,1.67159626534977,0.600890964381311));
#8750=CARTESIAN_POINT('Ctrl Pts',(97.7300874769289,1.67677329432323,0.586289506784017));
#8751=CARTESIAN_POINT('Ctrl Pts',(97.7284562666619,1.6844261484165,0.563774165282989));
#8752=CARTESIAN_POINT('Ctrl Pts',(97.727890706222,1.68703855584239,0.555907975311019));
#8753=CARTESIAN_POINT('Ctrl Pts',(97.7268466064179,1.69178672199528,0.541269039885092));
#8754=CARTESIAN_POINT('Ctrl Pts',(97.7263672900859,1.69393698150973,0.534501628853972));
#8755=CARTESIAN_POINT('Ctrl Pts',(97.7252576935113,1.6988447916866,0.518728382762341));
#8756=CARTESIAN_POINT('Ctrl Pts',(97.7246291899807,1.70157137852542,0.509713267442633));
#8757=CARTESIAN_POINT('Ctrl Pts',(97.7225988897404,1.71019917986507,0.480345559955327));
#8758=CARTESIAN_POINT('Ctrl Pts',(97.7212125679938,1.71580817779871,0.45990812653986));
#8759=CARTESIAN_POINT('Ctrl Pts',(97.7114075839688,1.75330038296824,0.313049291815026));
#8760=CARTESIAN_POINT('Ctrl Pts',(97.7035642303021,1.77154816250142,0.183542283052406));
#8761=CARTESIAN_POINT('Ctrl Pts',(97.6934547137312,1.77645946109298,0.0196101616983407));
#8762=CARTESIAN_POINT('Ctrl Pts',(97.6913753020059,1.77651224263065,-0.0139812004696996));
#8763=CARTESIAN_POINT('Ctrl Pts',(97.6892780485025,1.77561363630377,-0.0475423713344133));
#8764=CARTESIAN_POINT('Ctrl Pts',(97.5395353031289,1.77561364475627,-0.0475420556493824));
#8765=CARTESIAN_POINT('Ctrl Pts',(97.5425586847016,1.77690413202303,0.000655414316051098));
#8766=CARTESIAN_POINT('Ctrl Pts',(97.5456233416066,1.77623234914152,0.0489096839338776));
#8767=CARTESIAN_POINT('Ctrl Pts',(97.5502625108346,1.77231499271284,0.120461303337754));
#8768=CARTESIAN_POINT('Ctrl Pts',(97.5517901044051,1.77057478767216,0.14379220025042));
#8769=CARTESIAN_POINT('Ctrl Pts',(97.5542510280419,1.76706288314405,0.18096195333014));
#8770=CARTESIAN_POINT('Ctrl Pts',(97.555175033585,1.76558801832578,0.194826569943365));
#8771=CARTESIAN_POINT('Ctrl Pts',(97.5569436102543,1.76247042131107,0.221180292731501));
#8772=CARTESIAN_POINT('Ctrl Pts',(97.5577871813323,1.76085775191497,0.233672144835478));
#8773=CARTESIAN_POINT('Ctrl Pts',(97.55971687325,1.7568851281505,0.262063040706086));
#8774=CARTESIAN_POINT('Ctrl Pts',(97.5608055638305,1.75444197532685,0.277949125473025));
#8775=CARTESIAN_POINT('Ctrl Pts',(97.5643084824895,1.74594203684482,0.328630141396153));
#8776=CARTESIAN_POINT('Ctrl Pts',(97.5667482812997,1.73906331039275,0.363276561632091));
#8777=CARTESIAN_POINT('Ctrl Pts',(97.5785376134707,1.70133176282299,0.527521962657322));
#8778=CARTESIAN_POINT('Ctrl Pts',(97.5882996383161,1.65699991275731,0.653567004216802));
#8779=CARTESIAN_POINT('Ctrl Pts',(97.6033019644879,1.56752829277696,0.838538541028123));
#8780=CARTESIAN_POINT('Ctrl Pts',(97.6085459003841,1.53209652977743,0.901650740422808));
#8781=CARTESIAN_POINT('Ctrl Pts',(97.6148566838,1.48331286868377,0.977323332058229));
#8782=CARTESIAN_POINT('Ctrl Pts',(97.6160875494375,1.4734903662234,0.992070643697838));
#8783=CARTESIAN_POINT('Ctrl Pts',(97.6179052908165,1.45849829640912,1.01386541061438));
#8784=CARTESIAN_POINT('Ctrl Pts',(97.6185022169071,1.4534950569604,1.02102520976362));
#8785=CARTESIAN_POINT('Ctrl Pts',(97.6195272764258,1.44476095753207,1.03332967459584));
#8786=CARTESIAN_POINT('Ctrl Pts',(97.6199570313881,1.44105509690339,1.03849152716279));
#8787=CARTESIAN_POINT('Ctrl Pts',(97.6209654258572,1.43225530557543,1.0506108455963));
#8788=CARTESIAN_POINT('Ctrl Pts',(97.6215424769177,1.42713832285308,1.0575512396253));
#8789=CARTESIAN_POINT('Ctrl Pts',(97.6232220039917,1.41201362826333,1.077755841736));
#8790=CARTESIAN_POINT('Ctrl Pts',(97.6243156301994,1.40186979439358,1.09091762711231));
#8791=CARTESIAN_POINT('Ctrl Pts',(97.6328776694483,1.32025343362954,1.19379736865903));
#8792=CARTESIAN_POINT('Ctrl Pts',(97.6398601416418,1.24041753488387,1.27655507653146));
#8793=CARTESIAN_POINT('Ctrl Pts',(97.6538722981848,1.06682691655794,1.42471885462746));
#8794=CARTESIAN_POINT('Ctrl Pts',(97.6608748569019,0.973655896634358,1.48994404688947));
#8795=CARTESIAN_POINT('Ctrl Pts',(97.669688355139,0.855329321199499,1.55691421621624));
#8796=CARTESIAN_POINT('Ctrl Pts',(97.6711587363999,0.83554370618768,1.5676213716582));
#8797=CARTESIAN_POINT('Ctrl Pts',(97.6735495207309,0.803342261584215,1.58426463906003));
#8798=CARTESIAN_POINT('Ctrl Pts',(97.6744615391623,0.791051094788556,1.59043748171712));
#8799=CARTESIAN_POINT('Ctrl Pts',(97.6762218527198,0.76732268184386,1.60201120949056));
#8800=CARTESIAN_POINT('Ctrl Pts',(97.6770693205909,0.755896966967381,1.60743390981106));
#8801=CARTESIAN_POINT('Ctrl Pts',(97.679029059649,0.729477219176431,1.61962888119423));
#8802=CARTESIAN_POINT('Ctrl Pts',(97.6801441894382,0.714445254834644,1.62631567418661));
#8803=CARTESIAN_POINT('Ctrl Pts',(97.6838313674153,0.664762223535504,1.64759485489488));
#8804=CARTESIAN_POINT('Ctrl Pts',(97.686432936118,0.629742638082642,1.66129511508623));
#8805=CARTESIAN_POINT('Ctrl Pts',(97.6982401041299,0.47105139360017,1.71763922613347));
#8806=CARTESIAN_POINT('Ctrl Pts',(97.7078314111602,0.343343451211992,1.74764969268258));
#8807=CARTESIAN_POINT('Ctrl Pts',(97.7225976416918,0.142535472152848,1.77196529599101));
#8808=CARTESIAN_POINT('Ctrl Pts',(97.7277816840557,0.0710851755450795,1.77626749882615));
#8809=CARTESIAN_POINT('Ctrl Pts',(97.7340297739119,-0.0180668696401158,
1.77624561983836));
#8810=CARTESIAN_POINT('Ctrl Pts',(97.7352545122925,-0.0356975912649656,
1.77597878719614));
#8811=CARTESIAN_POINT('Ctrl Pts',(97.7370650612153,-0.0620359187743667,
1.77518776588008));
#8812=CARTESIAN_POINT('Ctrl Pts',(97.7376608108302,-0.0707477952616069,
1.77486191487761));
#8813=CARTESIAN_POINT('Ctrl Pts',(97.7387324464921,-0.0865075477073852,
1.77415622606674));
#8814=CARTESIAN_POINT('Ctrl Pts',(97.7392094808993,-0.0935558722339675,
1.77379851533988));
#8815=CARTESIAN_POINT('Ctrl Pts',(97.7402899875013,-0.10959472234161,1.77288865511995));
#8816=CARTESIAN_POINT('Ctrl Pts',(97.7408920047095,-0.118583389984603,1.77231012382063));
#8817=CARTESIAN_POINT('Ctrl Pts',(97.7427635291836,-0.146675619950463,1.7702873602638));
#8818=CARTESIAN_POINT('Ctrl Pts',(97.7440206133399,-0.165761174770733,1.76860238075398));
#8819=CARTESIAN_POINT('Ctrl Pts',(97.7469983195556,-0.211372283655386,1.7638307003064));
#8820=CARTESIAN_POINT('Ctrl Pts',(97.7487062545554,-0.237863310459977,1.76045396915936));
#8821=CARTESIAN_POINT('Ctrl Pts',(97.755466897655,-0.343509538651874,1.74455907919223));
#8822=CARTESIAN_POINT('Ctrl Pts',(97.7603695669039,-0.421857354911061,1.72728783200836));
#8823=CARTESIAN_POINT('Ctrl Pts',(97.7719887950462,-0.603533472988367,1.67413412309499));
#8824=CARTESIAN_POINT('Ctrl Pts',(97.7787054078985,-0.705231803194474,1.63389787011403));
#8825=CARTESIAN_POINT('Ctrl Pts',(97.7873151561424,-0.824466380498535,1.57350584355566));
#8826=CARTESIAN_POINT('Ctrl Pts',(97.788908784359,-0.846110762977519,1.56197373070925));
#8827=CARTESIAN_POINT('Ctrl Pts',(97.791539561245,-0.881093490031954,1.54239446335952));
#8828=CARTESIAN_POINT('Ctrl Pts',(97.7925673018254,-0.894577397893878,1.53461319954098));
#8829=CARTESIAN_POINT('Ctrl Pts',(97.7944331557519,-0.91871741597027,1.52025626636946));
#8830=CARTESIAN_POINT('Ctrl Pts',(97.7952689513567,-0.929409689604636,1.51374318195242));
#8831=CARTESIAN_POINT('Ctrl Pts',(97.7970765109963,-0.95226818095429,1.49948569408843));
#8832=CARTESIAN_POINT('Ctrl Pts',(97.7980495724369,-0.96441064730009,1.49170510396853));
#8833=CARTESIAN_POINT('Ctrl Pts',(97.8007719013291,-0.997921549224405,1.46965197228837));
#8834=CARTESIAN_POINT('Ctrl Pts',(97.8025329107228,-1.01907628718828,1.45506279536731));
#8835=CARTESIAN_POINT('Ctrl Pts',(97.8101401281606,-1.10820146556018,1.39070133401691));
#8836=CARTESIAN_POINT('Ctrl Pts',(97.8161488427617,-1.17289214131673,1.33659311260837));
#8837=CARTESIAN_POINT('Ctrl Pts',(97.8315215010746,-1.32533595371766,1.18947057894043));
#8838=CARTESIAN_POINT('Ctrl Pts',(97.8409922241215,-1.4073574069972,1.09119294837478));
#8839=CARTESIAN_POINT('Ctrl Pts',(97.8516596605576,-1.49103969379446,0.96561169987598));
#8840=CARTESIAN_POINT('Ctrl Pts',(97.853287338811,-1.50355984265597,0.945998546056781));
#8841=CARTESIAN_POINT('Ctrl Pts',(97.8555176095748,-1.52041168021235,0.918419474345613));
#8842=CARTESIAN_POINT('Ctrl Pts',(97.8561389019386,-1.52507263900095,0.910658806975379));
#8843=CARTESIAN_POINT('Ctrl Pts',(97.8572491516214,-1.53334470898269,0.896643860124756));
#8844=CARTESIAN_POINT('Ctrl Pts',(97.8577394416453,-1.53697739073637,0.89040255841188));
#8845=CARTESIAN_POINT('Ctrl Pts',(97.8587483952373,-1.54441268115744,0.877446903239372));
#8846=CARTESIAN_POINT('Ctrl Pts',(97.8592667165369,-1.5482097659704,0.870729650341733));
#8847=CARTESIAN_POINT('Ctrl Pts',(97.8606381682904,-1.55819196748425,0.852798830530928));
#8848=CARTESIAN_POINT('Ctrl Pts',(97.8614865912363,-1.56429992888596,0.841542517599367));
#8849=CARTESIAN_POINT('Ctrl Pts',(97.865799759499,-1.59496612214828,0.783540245267494));
#8850=CARTESIAN_POINT('Ctrl Pts',(97.8691583242864,-1.61755519354283,0.735777533661978));
#8851=CARTESIAN_POINT('Ctrl Pts',(97.8826352233069,-1.70087074363245,0.53715345997276));
#8852=CARTESIAN_POINT('Ctrl Pts',(97.8923040251559,-1.74287675597427,0.379313492927175));
#8853=CARTESIAN_POINT('Ctrl Pts',(97.9048635937319,-1.76699544275429,0.184242241589279));
#8854=CARTESIAN_POINT('Ctrl Pts',(97.9070593723809,-1.77019562383987,0.150417125199075));
#8855=CARTESIAN_POINT('Ctrl Pts',(97.9103378428348,-1.77347793073927,0.100490046205927));
#8856=CARTESIAN_POINT('Ctrl Pts',(97.9113971299915,-1.77431433485467,0.0844442606645976));
#8857=CARTESIAN_POINT('Ctrl Pts',(97.9132989634496,-1.77541785751231,0.0558043210656278));
#8858=CARTESIAN_POINT('Ctrl Pts',(97.914138826311,-1.77576890269678,0.0432143635474879));
#8859=CARTESIAN_POINT('Ctrl Pts',(97.9159175655818,-1.77622644058033,0.0166785196096828));
#8860=CARTESIAN_POINT('Ctrl Pts',(97.9168573342802,-1.7763026353616,0.00273303967374188));
#8861=CARTESIAN_POINT('Ctrl Pts',(97.9193884676931,-1.77606686676729,-0.0346191132123111));
#8862=CARTESIAN_POINT('Ctrl Pts',(97.9209890141123,-1.77545643032106,-0.0580204354177988));
#8863=CARTESIAN_POINT('Ctrl Pts',(97.9303005656727,-1.76927075674116,-0.192854587791792));
#8864=CARTESIAN_POINT('Ctrl Pts',(97.9383219233224,-1.75366936091735,-0.303558416506494));
#8865=CARTESIAN_POINT('Ctrl Pts',(97.9548536607572,-1.70113338126843,-0.523850692904557));
#8866=CARTESIAN_POINT('Ctrl Pts',(97.9633305628131,-1.66368074194744,-0.632806885667819));
#8867=CARTESIAN_POINT('Ctrl Pts',(97.9725374940179,-1.6090704094395,-0.752483809863521));
#8868=CARTESIAN_POINT('Ctrl Pts',(97.973689173362,-1.6019695329526,-0.767484939020849));
#8869=CARTESIAN_POINT('Ctrl Pts',(97.9754210735959,-1.59086308487221,-0.79012213038731));
#8870=CARTESIAN_POINT('Ctrl Pts',(97.9760098343347,-1.58701066898874,-0.797831736687428));
#8871=CARTESIAN_POINT('Ctrl Pts',(97.9770266913584,-1.58022042939027,-0.811176823038558));
#8872=CARTESIAN_POINT('Ctrl Pts',(97.9774563150506,-1.57730833768481,-0.816824861683276));
#8873=CARTESIAN_POINT('Ctrl Pts',(97.9784722324572,-1.57031946963772,-0.830203104135587));
#8874=CARTESIAN_POINT('Ctrl Pts',(97.9790568440424,-1.56621588280704,-0.837918998073964));
#8875=CARTESIAN_POINT('Ctrl Pts',(97.9808181821864,-1.55360975473148,-0.861205854619897));
#8876=CARTESIAN_POINT('Ctrl Pts',(97.9819844830017,-1.54493044487041,-0.876680542353074));
#8877=CARTESIAN_POINT('Ctrl Pts',(97.9878595995566,-1.49960128193414,-0.954735135648458));
#8878=CARTESIAN_POINT('Ctrl Pts',(97.9923840174514,-1.45937163277881,-1.01516497826087));
#8879=CARTESIAN_POINT('Ctrl Pts',(98.0051211547573,-1.33469436489176,-1.17964988082152));
#8880=CARTESIAN_POINT('Ctrl Pts',(98.0132080430048,-1.2420402602709,-1.2768386178051));
#8881=CARTESIAN_POINT('Ctrl Pts',(98.0239750277157,-1.11272924210098,-1.38495553804921));
#8882=CARTESIAN_POINT('Ctrl Pts',(98.0262177713969,-1.08546260600003,-1.4064277030494));
#8883=CARTESIAN_POINT('Ctrl Pts',(98.0295495057299,-1.04461920518179,-1.43669595192929));
#8884=CARTESIAN_POINT('Ctrl Pts',(98.0306138139149,-1.03152239950535,-1.44612795175987));
#8885=CARTESIAN_POINT('Ctrl Pts',(98.0325194317244,-1.0079986170815,-1.46258705585762));
#8886=CARTESIAN_POINT('Ctrl Pts',(98.0333579798927,-0.997622008173373,-1.46968446370513));
#8887=CARTESIAN_POINT('Ctrl Pts',(98.035142894318,-0.975487628671854,-1.48448154543761));
#8888=CARTESIAN_POINT('Ctrl Pts',(98.036090248123,-0.963712115236208,-1.4921529786152));
#8889=CARTESIAN_POINT('Ctrl Pts',(98.0386646325251,-0.93164735285255,-1.51250443763817));
#8890=CARTESIAN_POINT('Ctrl Pts',(98.0403014005506,-0.911191547132932,-1.5249151881083));
#8891=CARTESIAN_POINT('Ctrl Pts',(98.0496210260315,-0.794384693386821,-1.5925936399937));
#8892=CARTESIAN_POINT('Ctrl Pts',(98.0576098467225,-0.693282340216207,-1.6391318813214));
#8893=CARTESIAN_POINT('Ctrl Pts',(98.0740667416858,-0.480588425955996,-1.71382127789952));
#8894=CARTESIAN_POINT('Ctrl Pts',(98.0825016559088,-0.369245924892541,-1.74120931554221));
#8895=CARTESIAN_POINT('Ctrl Pts',(98.0916745135745,-0.239564446111824,-1.76009943371607));
#8896=CARTESIAN_POINT('Ctrl Pts',(98.0928297650041,-0.223058957020188,-1.76226725896373));
#8897=CARTESIAN_POINT('Ctrl Pts',(98.0945659201883,-0.197954466757662,-1.76520609197967));
#8898=CARTESIAN_POINT('Ctrl Pts',(98.0951554241278,-0.189376801999137,-1.76614692276035));
#8899=CARTESIAN_POINT('Ctrl Pts',(98.096172995095,-0.174471283318033,-1.76767197425584));
#8900=CARTESIAN_POINT('Ctrl Pts',(98.0966025983444,-0.168146831454844,-1.76828478573917));
#8901=CARTESIAN_POINT('Ctrl Pts',(98.0976177569636,-0.153127524129337,-1.76965877952667));
#8902=CARTESIAN_POINT('Ctrl Pts',(98.0982016389986,-0.144430183136867,-1.77038983413899));
#8903=CARTESIAN_POINT('Ctrl Pts',(98.0999584478457,-0.118096614105517,-1.77240794650525));
#8904=CARTESIAN_POINT('Ctrl Pts',(98.101121027297,-0.100445630535094,-1.7734958338457));
#8905=CARTESIAN_POINT('Ctrl Pts',(98.1069580150417,-0.0108759779991224,
-1.77767468756287));
#8906=CARTESIAN_POINT('Ctrl Pts',(98.1114506752503,0.0611742825880121,-1.77665572367131));
#8907=CARTESIAN_POINT('Ctrl Pts',(98.1240564817259,0.264826494166932,-1.76136733671736));
#8908=CARTESIAN_POINT('Ctrl Pts',(98.1320440159963,0.395155384570257,-1.73677815796907));
#8909=CARTESIAN_POINT('Ctrl Pts',(98.1427875808873,0.556178398088762,-1.68731802837179));
#8910=CARTESIAN_POINT('Ctrl Pts',(98.1451262653825,0.590474006407298,-1.67562427133545));
#8911=CARTESIAN_POINT('Ctrl Pts',(98.1485618274086,0.639577099906993,-1.65718692031408));
#8912=CARTESIAN_POINT('Ctrl Pts',(98.1496312881101,0.654688548133184,-1.65127533486647));
#8913=CARTESIAN_POINT('Ctrl Pts',(98.1515446157408,0.681400949134859,-1.64040115843671));
#8914=CARTESIAN_POINT('Ctrl Pts',(98.1523856776915,0.693034144509014,-1.63552036812227));
#8915=CARTESIAN_POINT('Ctrl Pts',(98.1541598759638,0.717339372620875,-1.62501706439367));
#8916=CARTESIAN_POINT('Ctrl Pts',(98.1550938299829,0.729999497315904,-1.61936930624657));
#8917=CARTESIAN_POINT('Ctrl Pts',(98.1575918864274,0.76349718098708,-1.60395315069062));
#8918=CARTESIAN_POINT('Ctrl Pts',(98.1591647545552,0.784212598631661,-1.59392727823774));
#8919=CARTESIAN_POINT('Ctrl Pts',(98.1687504837128,0.908153302718764,-1.53094133552961));
#8920=CARTESIAN_POINT('Ctrl Pts',(98.177102559885,1.0061635644245,-1.46838338638781));
#8921=CARTESIAN_POINT('Ctrl Pts',(98.193662273175,1.1844411984287,-1.32831724905043));
#8922=CARTESIAN_POINT('Ctrl Pts',(98.2018179603839,1.26493859002854,-1.25190326577961));
#8923=CARTESIAN_POINT('Ctrl Pts',(98.2107712597663,1.34904972000503,-1.15560433882296));
#8924=CARTESIAN_POINT('Ctrl Pts',(98.211958443334,1.36011387238599,-1.1425615270612));
#8925=CARTESIAN_POINT('Ctrl Pts',(98.2137248255919,1.37646531003053,-1.12271167898388));
#8926=CARTESIAN_POINT('Ctrl Pts',(98.2143132930364,1.38189391183424,-1.11602306789876));
#8927=CARTESIAN_POINT('Ctrl Pts',(98.2153298688578,1.39124246731377,-1.10433185387431));
#8928=CARTESIAN_POINT('Ctrl Pts',(98.2157595011614,1.39518443365512,-1.09934746350167));
#8929=CARTESIAN_POINT('Ctrl Pts',(98.2167757204004,1.40448652677752,-1.08745487489939));
#8930=CARTESIAN_POINT('Ctrl Pts',(98.2173606217157,1.40982250082346,-1.08052812692499));
#8931=CARTESIAN_POINT('Ctrl Pts',(98.2191237605207,1.42584362089369,-1.05941001590188));
#8932=CARTESIAN_POINT('Ctrl Pts',(98.2202915410238,1.43636759683231,-1.04509702842376));
#8933=CARTESIAN_POINT('Ctrl Pts',(98.2261818779144,1.48887793920055,-0.971389118555967));
#8934=CARTESIAN_POINT('Ctrl Pts',(98.2307189733209,1.527406738542,-0.909607234055698));
#8935=CARTESIAN_POINT('Ctrl Pts',(98.2435088905345,1.62608287019497,-0.727333496393834));
#8936=CARTESIAN_POINT('Ctrl Pts',(98.251635824275,1.67647483199959,-0.602154085750077));
#8937=CARTESIAN_POINT('Ctrl Pts',(98.2624129259529,1.72132495878054,-0.439621394110926));
#8938=CARTESIAN_POINT('Ctrl Pts',(98.2646176201938,1.72944580936269,-0.406501578108011));
#8939=CARTESIAN_POINT('Ctrl Pts',(98.2679035038079,1.73997654347827,-0.357495099775459));
#8940=CARTESIAN_POINT('Ctrl Pts',(98.2689610024306,1.74313240598006,-0.341775519017846));
#8941=CARTESIAN_POINT('Ctrl Pts',(98.2708590945617,1.74838028470816,-0.313668936708854));
#8942=CARTESIAN_POINT('Ctrl Pts',(98.2716970093455,1.7505545312382,-0.301298259295974));
#8943=CARTESIAN_POINT('Ctrl Pts',(98.2734855465802,1.75489320772866,-0.274978427330228));
#8944=CARTESIAN_POINT('Ctrl Pts',(98.2744372097997,1.75702290508012,-0.261024514166255));
#8945=CARTESIAN_POINT('Ctrl Pts',(98.2770362337843,1.76235455455678,-0.223062931168784));
#8946=CARTESIAN_POINT('Ctrl Pts',(98.2786936546126,1.76523204234351,-0.199013524262738));
#8947=CARTESIAN_POINT('Ctrl Pts',(98.2824231014625,1.77054965998076,-0.145275567998812));
#8948=CARTESIAN_POINT('Ctrl Pts',(98.2845023180137,1.77273645006418,-0.115569846465187));
#8949=CARTESIAN_POINT('Ctrl Pts',(98.2875024743817,1.77479247071467,-0.0730675819004155));
#8950=CARTESIAN_POINT('Ctrl Pts',(98.2884065155601,1.77527188706779,-0.060306055167887));
#8951=CARTESIAN_POINT('Ctrl Pts',(98.2893138640945,1.77561363880419,-0.0475422779488097));
#8952=CARTESIAN_POINT('Origin',(88.3562164250559,0.,0.));
#8953=CARTESIAN_POINT('',(99.1886897654568,1.7756136354609,-0.0475424028141329));
#8954=CARTESIAN_POINT('',(99.0404834457757,1.77561363837197,-0.0475422940912327));
#8955=CARTESIAN_POINT('',(88.3562164250559,1.77561363837197,-0.0475422940912398));
#8956=CARTESIAN_POINT('Ctrl Pts',(99.1886897654568,1.7756136354609,-0.0475424028141329));
#8957=CARTESIAN_POINT('Ctrl Pts',(99.1873699206532,1.77512914690477,-0.0656370811550229));
#8958=CARTESIAN_POINT('Ctrl Pts',(99.1860471354729,1.7743679485596,-0.0837286617151811));
#8959=CARTESIAN_POINT('Ctrl Pts',(99.1793003110797,1.76907863564114,-0.175857315182797));
#8960=CARTESIAN_POINT('Ctrl Pts',(99.1738633091114,1.76019369025663,-0.249567866918385));
#8961=CARTESIAN_POINT('Ctrl Pts',(99.1667114157917,1.74207524440372,-0.347698136066784));
#8962=CARTESIAN_POINT('Ctrl Pts',(99.164891219588,1.73687998037377,-0.372784416741384));
#8963=CARTESIAN_POINT('Ctrl Pts',(99.1617894940502,1.72698399410244,-0.415855038824187));
#8964=CARTESIAN_POINT('Ctrl Pts',(99.1604976011994,1.72254037392542,-0.433893832062961));
#8965=CARTESIAN_POINT('Ctrl Pts',(99.1586084370482,1.71555068728041,-0.460466159680731));
#8966=CARTESIAN_POINT('Ctrl Pts',(99.1579999776554,1.7132223131871,-0.469054963715754));
#8967=CARTESIAN_POINT('Ctrl Pts',(99.1569156947934,1.70893232588123,-0.484421452230894));
#8968=CARTESIAN_POINT('Ctrl Pts',(99.1564385712949,1.70699477678849,-0.491205328267051));
#8969=CARTESIAN_POINT('Ctrl Pts',(99.1553703744786,1.70254447867655,-0.506442617270516));
#8970=CARTESIAN_POINT('Ctrl Pts',(99.1547806007327,1.70000914543613,-0.514889056157521));
#8971=CARTESIAN_POINT('Ctrl Pts',(99.1529869324508,1.69206200152012,-0.540666132608314));
#8972=CARTESIAN_POINT('Ctrl Pts',(99.1517940331954,1.68644711371781,-0.557933579656584));
#8973=CARTESIAN_POINT('Ctrl Pts',(99.1451408457443,1.65332744171262,-0.654714378491946));
#8974=CARTESIAN_POINT('Ctrl Pts',(99.1399305756441,1.62046211518054,-0.732289831956704));
#8975=CARTESIAN_POINT('Ctrl Pts',(99.1300825417102,1.54769569438742,-0.874912545650337));
#8976=CARTESIAN_POINT('Ctrl Pts',(99.1254481941692,1.50887058439876,-0.940288872112908));
#8977=CARTESIAN_POINT('Ctrl Pts',(99.1163723231202,1.42648412994783,-1.06070714945549));
#8978=CARTESIAN_POINT('Ctrl Pts',(99.1119529097125,1.38361658356158,-1.11604664742778));
#8979=CARTESIAN_POINT('Ctrl Pts',(99.1060748640552,1.32413504167857,-1.18412387890668));
#8980=CARTESIAN_POINT('Ctrl Pts',(99.1047338502697,1.31040341616098,-1.19930221350897));
#8981=CARTESIAN_POINT('Ctrl Pts',(99.1025012126737,1.28730031616615,-1.22396881575017));
#8982=CARTESIAN_POINT('Ctrl Pts',(99.1016159952707,1.27807857362856,-1.23359511554692));
#8983=CARTESIAN_POINT('Ctrl Pts',(99.0998787946056,1.25986787591144,-1.25218131804407));
#8984=CARTESIAN_POINT('Ctrl Pts',(99.0990273049256,1.25088950074996,-1.26115049079156));
#8985=CARTESIAN_POINT('Ctrl Pts',(99.0969700306806,1.2290770269545,-1.28247852151722));
#8986=CARTESIAN_POINT('Ctrl Pts',(99.0957601899482,1.21615180271376,-1.29474176910311));
#8987=CARTESIAN_POINT('Ctrl Pts',(99.0922984825246,1.1789060009306,-1.32903017236865));
#8988=CARTESIAN_POINT('Ctrl Pts',(99.0900271611737,1.1541577104816,-1.35057776217391));
#8989=CARTESIAN_POINT('Ctrl Pts',(99.077599020635,1.01713832830286,-1.46335912793677));
#8990=CARTESIAN_POINT('Ctrl Pts',(99.0669424133231,0.894648189740849,-1.54129234742769));
#8991=CARTESIAN_POINT('Ctrl Pts',(99.0515812841342,0.704130242149068,-1.63207761749249));
#8992=CARTESIAN_POINT('Ctrl Pts',(99.0467963408315,0.642600006962748,-1.65727000778688));
#8993=CARTESIAN_POINT('Ctrl Pts',(99.0412330984514,0.567019447503088,-1.68337035249738));
#8994=CARTESIAN_POINT('Ctrl Pts',(99.0402995400953,0.554191478800444,-1.68763699598252));
#8995=CARTESIAN_POINT('Ctrl Pts',(99.0388351674416,0.533819995090226,-1.69415530905732));
#8996=CARTESIAN_POINT('Ctrl Pts',(99.038299083708,0.526308378360015,-1.69650390370777));
#8997=CARTESIAN_POINT('Ctrl Pts',(99.0372819774564,0.511948624279342,-1.70088909297112));
#8998=CARTESIAN_POINT('Ctrl Pts',(99.0368004945401,0.505103496033442,-1.70293439701532));
#8999=CARTESIAN_POINT('Ctrl Pts',(99.0356256872041,0.488289846014576,-1.70784796794033));
#9000=CARTESIAN_POINT('Ctrl Pts',(99.0349349586907,0.47830798897307,-1.71067037620324));
#9001=CARTESIAN_POINT('Ctrl Pts',(99.0325429061172,0.443428875501544,-1.72020340833021));
#9002=CARTESIAN_POINT('Ctrl Pts',(99.0308650970601,0.418409432791615,-1.72645956948996));
#9003=CARTESIAN_POINT('Ctrl Pts',(99.0221571154692,0.286229280981088,-1.75646894642826));
#9004=CARTESIAN_POINT('Ctrl Pts',(99.0154958048069,0.17716430432951,-1.77079875419169));
#9005=CARTESIAN_POINT('Ctrl Pts',(99.0026524058217,-0.0316621692219442,
-1.77873604865749));
#9006=CARTESIAN_POINT('Ctrl Pts',(98.9965074972078,-0.130919084806953,-1.77419315806105));
#9007=CARTESIAN_POINT('Ctrl Pts',(98.9884601664649,-0.254526036309295,-1.75810385154298));
#9008=CARTESIAN_POINT('Ctrl Pts',(98.9868007823962,-0.279705768338904,-1.75427399021902));
#9009=CARTESIAN_POINT('Ctrl Pts',(98.9841782154192,-0.318955226113086,-1.74743762863328));
#9010=CARTESIAN_POINT('Ctrl Pts',(98.9832266779609,-0.333086153989404,-1.74479921360548));
#9011=CARTESIAN_POINT('Ctrl Pts',(98.9814357495065,-0.359466984547717,-1.7395414440401));
#9012=CARTESIAN_POINT('Ctrl Pts',(98.9805977288283,-0.371724289320995,-1.73696343869477));
#9013=CARTESIAN_POINT('Ctrl Pts',(98.9787041946085,-0.399218392198995,-1.7308764227673));
#9014=CARTESIAN_POINT('Ctrl Pts',(98.9776464288059,-0.414438015027777,-1.72729546399883));
#9015=CARTESIAN_POINT('Ctrl Pts',(98.974411174572,-0.460554014717092,-1.715800460705));
#9016=CARTESIAN_POINT('Ctrl Pts',(98.9722136802158,-0.491284830873417,-1.70725516785119));
#9017=CARTESIAN_POINT('Ctrl Pts',(98.9604427056008,-0.652703533446317,-1.65765059066628));
#9018=CARTESIAN_POINT('Ctrl Pts',(98.9504144440548,-0.778527243201682,-1.60240774180693));
#9019=CARTESIAN_POINT('Ctrl Pts',(98.9345701423892,-0.965804983480632,-1.49287910030096));
#9020=CARTESIAN_POINT('Ctrl Pts',(98.9287660000946,-1.03207821052265,-1.44785518781079));
#9021=CARTESIAN_POINT('Ctrl Pts',(98.9222204793852,-1.10608561051922,-1.38990415039842));
#9022=CARTESIAN_POINT('Ctrl Pts',(98.9212557619064,-1.1169749239136,-1.38116833693476));
#9023=CARTESIAN_POINT('Ctrl Pts',(98.9197539215046,-1.13391468846448,-1.36724723206105));
#9024=CARTESIAN_POINT('Ctrl Pts',(98.9192110885588,-1.14003490586894,-1.36214827899283));
#9025=CARTESIAN_POINT('Ctrl Pts',(98.9181841629665,-1.15161196418613,-1.35237036688754));
#9026=CARTESIAN_POINT('Ctrl Pts',(98.9176995756184,-1.15707495317854,-1.34769925418989));
#9027=CARTESIAN_POINT('Ctrl Pts',(98.9165326220393,-1.17022669439044,-1.33631497922606));
#9028=CARTESIAN_POINT('Ctrl Pts',(98.9158526686074,-1.17788635874265,-1.32956834284475));
#9029=CARTESIAN_POINT('Ctrl Pts',(98.9135447430441,-1.20385341605598,-1.30629600114507));
#9030=CARTESIAN_POINT('Ctrl Pts',(98.9119381097314,-1.22187547872979,-1.28945443899491));
#9031=CARTESIAN_POINT('Ctrl Pts',(98.9032271258343,-1.3188448833139,-1.1949774074261));
#9032=CARTESIAN_POINT('Ctrl Pts',(98.8965070480947,-1.3907585348469,-1.11045884628892));
#9033=CARTESIAN_POINT('Ctrl Pts',(98.883214932035,-1.51493909851543,-0.933362196504009));
#9034=CARTESIAN_POINT('Ctrl Pts',(98.8766740599553,-1.56770794998903,-0.841720424503123));
#9035=CARTESIAN_POINT('Ctrl Pts',(98.8683838946422,-1.62140276711668,-0.725682798524403));
#9036=CARTESIAN_POINT('Ctrl Pts',(98.8669244105442,-1.63039497666059,-0.705247902836286));
#9037=CARTESIAN_POINT('Ctrl Pts',(98.864546954758,-1.64428707962536,-0.671991263311253));
#9038=CARTESIAN_POINT('Ctrl Pts',(98.8636371929861,-1.64942785463916,-0.659272320560589));
#9039=CARTESIAN_POINT('Ctrl Pts',(98.8618782609334,-1.65902827709649,-0.634704261344452));
#9040=CARTESIAN_POINT('Ctrl Pts',(98.8610298838408,-1.6635095913183,-0.622864470650001));
#9041=CARTESIAN_POINT('Ctrl Pts',(98.8590636856041,-1.67355051486739,-0.59545449483932));
#9042=CARTESIAN_POINT('Ctrl Pts',(98.8579429444778,-1.679019982512,-0.579852780675154));
#9043=CARTESIAN_POINT('Ctrl Pts',(98.8543210889802,-1.69587996198853,-0.529519733712121));
#9044=CARTESIAN_POINT('Ctrl Pts',(98.851792545761,-1.7064158976022,-0.494514345614418));
#9045=CARTESIAN_POINT('Ctrl Pts',(98.8400231928364,-1.74983619067927,-0.332272339746914));
#9046=CARTESIAN_POINT('Ctrl Pts',(98.830389147513,-1.76961272206897,-0.201971393440725));
#9047=CARTESIAN_POINT('Ctrl Pts',(98.8155637833109,-1.7776965858352,0.000943296622551324));
#9048=CARTESIAN_POINT('Ctrl Pts',(98.8103646717862,-1.77620987103552,0.0727083615184915));
#9049=CARTESIAN_POINT('Ctrl Pts',(98.8041007872244,-1.76895462034831,0.161787635620858));
#9050=CARTESIAN_POINT('Ctrl Pts',(98.8028744860854,-1.76725930524357,0.179360795521043));
#9051=CARTESIAN_POINT('Ctrl Pts',(98.8010620916201,-1.76433531814633,0.205574856701156));
#9052=CARTESIAN_POINT('Ctrl Pts',(98.8004660308916,-1.76330457451399,0.214236136412348));
#9053=CARTESIAN_POINT('Ctrl Pts',(98.7994418672879,-1.76141272178564,0.229193498241413));
#9054=CARTESIAN_POINT('Ctrl Pts',(98.7990121526483,-1.7605815881873,0.235492910486742));
#9055=CARTESIAN_POINT('Ctrl Pts',(98.7980030010624,-1.75854126144492,0.250342266186049));
#9056=CARTESIAN_POINT('Ctrl Pts',(98.7974251625246,-1.75730350907491,0.258888012897894));
#9057=CARTESIAN_POINT('Ctrl Pts',(98.7957056589216,-1.75341307735095,0.284433946764175));
#9058=CARTESIAN_POINT('Ctrl Pts',(98.7945737065931,-1.75057557837745,0.30140552127845));
#9059=CARTESIAN_POINT('Ctrl Pts',(98.7846299695859,-1.72322291174428,0.451557777221006));
#9060=CARTESIAN_POINT('Ctrl Pts',(98.7764901417329,-1.68379547072324,0.581588340186751));
#9061=CARTESIAN_POINT('Ctrl Pts',(98.7628513182545,-1.59583225269337,0.784704088004222));
#9062=CARTESIAN_POINT('Ctrl Pts',(98.7574997962186,-1.55603159358649,0.860932253593579));
#9063=CARTESIAN_POINT('Ctrl Pts',(98.7502865302608,-1.49724771444616,0.9560257364921));
#9064=CARTESIAN_POINT('Ctrl Pts',(98.7485984007624,-1.48313805091659,0.977771618172882));
#9065=CARTESIAN_POINT('Ctrl Pts',(98.7459406468328,-1.46041969772443,1.01116154987498));
#9066=CARTESIAN_POINT('Ctrl Pts',(98.7449832047023,-1.45213557271491,1.02302279107987));
#9067=CARTESIAN_POINT('Ctrl Pts',(98.7431870959099,-1.43641631867426,1.04495400442521));
#9068=CARTESIAN_POINT('Ctrl Pts',(98.7423498765059,-1.42901780303677,1.05504920106986));
#9069=CARTESIAN_POINT('Ctrl Pts',(98.7404660198791,-1.41221560484216,1.07747463633437));
#9070=CARTESIAN_POINT('Ctrl Pts',(98.7394172292792,-1.40275599756727,1.08976148360643));
#9071=CARTESIAN_POINT('Ctrl Pts',(98.7363080390735,-1.37441226648112,1.12559585276744));
#9072=CARTESIAN_POINT('Ctrl Pts',(98.7342302778677,-1.35508823527885,1.14878665677154));
#9073=CARTESIAN_POINT('Ctrl Pts',(98.7204325224175,-1.22434633752994,1.29779948090917));
#9074=CARTESIAN_POINT('Ctrl Pts',(98.7079785404145,-1.09615172853382,1.40774210732993));
#9075=CARTESIAN_POINT('Ctrl Pts',(98.6919632391324,-0.909565392296823,1.52662703229225));
#9076=CARTESIAN_POINT('Ctrl Pts',(98.688156376503,-0.863390584741517,1.55320865574977));
#9077=CARTESIAN_POINT('Ctrl Pts',(98.683564517283,-0.804687215404461,1.58357420751393));
#9078=CARTESIAN_POINT('Ctrl Pts',(98.6826791809479,-0.793223580484867,1.58934740090699));
#9079=CARTESIAN_POINT('Ctrl Pts',(98.6812728054071,-0.774763722303712,1.59839446637652));
#9080=CARTESIAN_POINT('Ctrl Pts',(98.6807471543394,-0.767807223784897,1.60174772308159));
#9081=CARTESIAN_POINT('Ctrl Pts',(98.6797356776823,-0.754306483941104,1.60814734767734));
#9082=CARTESIAN_POINT('Ctrl Pts',(98.679249538319,-0.747765220445794,1.61119934860822));
#9083=CARTESIAN_POINT('Ctrl Pts',(98.6781599952481,-0.732991115181813,1.6179832475312));
#9084=CARTESIAN_POINT('Ctrl Pts',(98.6775579467952,-0.724747900945792,1.62169240391921));
#9085=CARTESIAN_POINT('Ctrl Pts',(98.6754247116542,-0.695271945151755,1.6346858998415));
#9086=CARTESIAN_POINT('Ctrl Pts',(98.673912859204,-0.673885264126018,1.64361791247423));
#9087=CARTESIAN_POINT('Ctrl Pts',(98.6623046201056,-0.506408404264219,1.70974467585286));
#9088=CARTESIAN_POINT('Ctrl Pts',(98.6530023601573,-0.353483373276005,1.74778090353368));
#9089=CARTESIAN_POINT('Ctrl Pts',(98.6391131644428,-0.132089153537259,1.77255557785057));
#9090=CARTESIAN_POINT('Ctrl Pts',(98.6349425856815,-0.0662934287961824,
1.7762332539265));
#9091=CARTESIAN_POINT('Ctrl Pts',(98.6293500445639,0.0196696588200166,1.77625504264761));
#9092=CARTESIAN_POINT('Ctrl Pts',(98.6280311999854,0.0397874647733673,1.77591829080341));
#9093=CARTESIAN_POINT('Ctrl Pts',(98.6258254644194,0.0731474008574148,1.7747927648004));
#9094=CARTESIAN_POINT('Ctrl Pts',(98.6249446590548,0.0863945041916861,1.77419724767929));
#9095=CARTESIAN_POINT('Ctrl Pts',(98.623198839252,0.112496560855711,1.77273082261834));
#9096=CARTESIAN_POINT('Ctrl Pts',(98.622334139683,0.125351176102582,1.77186825501714));
#9097=CARTESIAN_POINT('Ctrl Pts',(98.6202384786548,0.156320656236037,1.76945145617547));
#9098=CARTESIAN_POINT('Ctrl Pts',(98.6190032497908,0.174422929146081,1.76775880768756));
#9099=CARTESIAN_POINT('Ctrl Pts',(98.6144680747016,0.240312758147703,1.76057590224795));
#9100=CARTESIAN_POINT('Ctrl Pts',(98.6111171043335,0.287894255387175,1.75342347104452));
#9101=CARTESIAN_POINT('Ctrl Pts',(98.6021363238702,0.412514997033795,1.7294814229272));
#9102=CARTESIAN_POINT('Ctrl Pts',(98.5964240258592,0.488824131830416,1.70948043519826));
#9103=CARTESIAN_POINT('Ctrl Pts',(98.5826450819672,0.667703891289564,1.64963590685902));
#9104=CARTESIAN_POINT('Ctrl Pts',(98.5745590136591,0.768412630883759,1.60520181897494));
#9105=CARTESIAN_POINT('Ctrl Pts',(98.565665923048,0.87935361551117,1.54340375703528));
#9106=CARTESIAN_POINT('Ctrl Pts',(98.5644758319805,0.8942088587139,1.53484478359516));
#9107=CARTESIAN_POINT('Ctrl Pts',(98.5627060092614,0.916346437940334,1.5216594930648));
#9108=CARTESIAN_POINT('Ctrl Pts',(98.5621169579187,0.923722319863408,1.517193293806));
#9109=CARTESIAN_POINT('Ctrl Pts',(98.5610998026773,0.936477317073108,1.50934246592391));
#9110=CARTESIAN_POINT('Ctrl Pts',(98.5606701681046,0.941871065149031,1.50598251801909));
#9111=CARTESIAN_POINT('Ctrl Pts',(98.5596544760855,0.954636450601399,1.49793511712676));
#9112=CARTESIAN_POINT('Ctrl Pts',(98.5590700977939,0.961991682806987,1.49322214629639));
#9113=CARTESIAN_POINT('Ctrl Pts',(98.5573102784046,0.984161856493525,1.47878448003472));
#9114=CARTESIAN_POINT('Ctrl Pts',(98.5561452363389,0.998866819080417,1.4688918389474));
#9115=CARTESIAN_POINT('Ctrl Pts',(98.5502832049804,1.07282868776984,1.4175101612288));
#9116=CARTESIAN_POINT('Ctrl Pts',(98.5457696994683,1.1296657879425,1.37264487609026));
#9117=CARTESIAN_POINT('Ctrl Pts',(98.5330777487624,1.28300535612447,1.23560909922294));
#9118=CARTESIAN_POINT('Ctrl Pts',(98.5250250721187,1.37207628615552,1.135886130672));
#9119=CARTESIAN_POINT('Ctrl Pts',(98.5142664367791,1.46952153370502,0.998404293647805));
#9120=CARTESIAN_POINT('Ctrl Pts',(98.5119909188176,1.48902885531175,0.96907041697685));
#9121=CARTESIAN_POINT('Ctrl Pts',(98.5086310911144,1.51614024153341,0.925548837737813));
#9122=CARTESIAN_POINT('Ctrl Pts',(98.5075724747417,1.52444470690188,0.911806004866494));
#9123=CARTESIAN_POINT('Ctrl Pts',(98.5056713691768,1.53892810815905,0.887086774543881));
#9124=CARTESIAN_POINT('Ctrl Pts',(98.5048315551604,1.54517882786778,0.876153550208527));
#9125=CARTESIAN_POINT('Ctrl Pts',(98.5030524136949,1.55810824428382,0.852969766428469));
#9126=CARTESIAN_POINT('Ctrl Pts',(98.5021121885454,1.56475988554641,0.840705182908352));
#9127=CARTESIAN_POINT('Ctrl Pts',(98.4995785587272,1.58219644296248,0.807630979510274));
#9128=CARTESIAN_POINT('Ctrl Pts',(98.4979759411601,1.59271478525861,0.786684755368459));
#9129=CARTESIAN_POINT('Ctrl Pts',(98.4886126614864,1.65120819412982,0.664216375875407));
#9130=CARTESIAN_POINT('Ctrl Pts',(98.4805373497161,1.68987658660363,0.55855251845839));
#9131=CARTESIAN_POINT('Ctrl Pts',(98.4640172343482,1.74719880700822,0.339652453129529));
#9132=CARTESIAN_POINT('Ctrl Pts',(98.4556095231236,1.76539796340563,0.226806767744066));
#9133=CARTESIAN_POINT('Ctrl Pts',(98.4464588489229,1.7737135582986,0.0963452210403971));
#9134=CARTESIAN_POINT('Ctrl Pts',(98.4453013659596,1.77454000222293,0.0796870077196417));
#9135=CARTESIAN_POINT('Ctrl Pts',(98.4435625411103,1.77543811335797,0.054388791647298));
#9136=CARTESIAN_POINT('Ctrl Pts',(98.4429725613684,1.77568155931224,0.0457563415994727));
#9137=CARTESIAN_POINT('Ctrl Pts',(98.4419545159736,1.77599483952051,0.0307695705511481));
#9138=CARTESIAN_POINT('Ctrl Pts',(98.4415249086054,1.77609354557589,0.0244163263853195));
#9139=CARTESIAN_POINT('Ctrl Pts',(98.4405101703523,1.77624684551325,0.00934160670781613));
#9140=CARTESIAN_POINT('Ctrl Pts',(98.4399267076147,1.77627130396795,0.000620094314811771));
#9141=CARTESIAN_POINT('Ctrl Pts',(98.4384718880171,1.77617155357579,-0.0212499771479));
#9142=CARTESIAN_POINT('Ctrl Pts',(98.4376047832566,1.77596558586547,-0.0343977292065965));
#9143=CARTESIAN_POINT('Ctrl Pts',(98.436744300164,1.7756136383717,-0.047542294101169));
#9144=CARTESIAN_POINT('',(98.4812164250559,0.00162964136512414,1.77624925243307));
#9145=CARTESIAN_POINT('Ctrl Pts',(98.2893138640945,1.77561363880419,-0.0475422779488097));
#9146=CARTESIAN_POINT('Ctrl Pts',(98.2931977998273,1.77707651853614,0.00709349711413117));
#9147=CARTESIAN_POINT('Ctrl Pts',(98.2971436447791,1.77601699051399,0.0617704143106846));
#9148=CARTESIAN_POINT('Ctrl Pts',(98.3086015490245,1.76570929891744,0.218842284437513));
#9149=CARTESIAN_POINT('Ctrl Pts',(98.3161848227136,1.75009763405617,0.320593896543771));
#9150=CARTESIAN_POINT('Ctrl Pts',(98.3259897503879,1.71763954577045,0.45382854040931));
#9151=CARTESIAN_POINT('Ctrl Pts',(98.3284180199761,1.70853369093817,0.486989676364695));
#9152=CARTESIAN_POINT('Ctrl Pts',(98.3316004842894,1.69508870632277,0.530916033474651));
#9153=CARTESIAN_POINT('Ctrl Pts',(98.3323956139171,1.69159928941403,0.541931193820995));
#9154=CARTESIAN_POINT('Ctrl Pts',(98.3336429375755,1.68591446006054,0.559286592704036));
#9155=CARTESIAN_POINT('Ctrl Pts',(98.3340990689852,1.68379026039922,0.565649557764315));
#9156=CARTESIAN_POINT('Ctrl Pts',(98.3350506856983,1.679262107583,0.578961920465669));
#9157=CARTESIAN_POINT('Ctrl Pts',(98.3355457022361,1.67685096121182,0.585908685881759));
#9158=CARTESIAN_POINT('Ctrl Pts',(98.3367823785789,1.6706890459633,0.603312174024025));
#9159=CARTESIAN_POINT('Ctrl Pts',(98.3375208724404,1.66688310862648,0.613749285611066));
#9160=CARTESIAN_POINT('Ctrl Pts',(98.3404610780624,1.6512336725457,0.655445473337094));
#9161=CARTESIAN_POINT('Ctrl Pts',(98.3426214107926,1.6386059998908,0.686405218803319));
#9162=CARTESIAN_POINT('Ctrl Pts',(98.3485818342248,1.60082477898677,0.77203888233926));
#9163=CARTESIAN_POINT('Ctrl Pts',(98.3523084282866,1.57375555523373,0.825819871699164));
#9164=CARTESIAN_POINT('Ctrl Pts',(98.3646400300355,1.47470643534915,0.999977647631338));
#9165=CARTESIAN_POINT('Ctrl Pts',(98.3731414198256,1.39123372698692,1.11318418275383));
#9166=CARTESIAN_POINT('Ctrl Pts',(98.3837976143028,1.27834344994996,1.23349830291792));
#9167=CARTESIAN_POINT('Ctrl Pts',(98.3854151378637,1.26098438101382,1.25123871886078));
#9168=CARTESIAN_POINT('Ctrl Pts',(98.3879953173562,1.2329895117206,1.27867420360461));
#9169=CARTESIAN_POINT('Ctrl Pts',(98.388947190896,1.22259743628979,1.28861411729099));
#9170=CARTESIAN_POINT('Ctrl Pts',(98.3907383379673,1.20293128586108,1.30697254318422));
#9171=CARTESIAN_POINT('Ctrl Pts',(98.3915762360143,1.19368658332831,1.31542131427491));
#9172=CARTESIAN_POINT('Ctrl Pts',(98.3934689356629,1.17270905378348,1.33418951707691));
#9173=CARTESIAN_POINT('Ctrl Pts',(98.3945259822322,1.16092797662998,1.34445319670272));
#9174=CARTESIAN_POINT('Ctrl Pts',(98.3976834925259,1.12555424127244,1.37445917576315));
#9175=CARTESIAN_POINT('Ctrl Pts',(98.3998021300482,1.10158350881587,1.39374457630302));
#9176=CARTESIAN_POINT('Ctrl Pts',(98.4048402368584,1.04406461931032,1.43760976514977));
#9177=CARTESIAN_POINT('Ctrl Pts',(98.4077779307064,1.01013114047404,1.46165228186317));
#9178=CARTESIAN_POINT('Ctrl Pts',(98.4186470344951,0.883069555781208,1.54513891247854));
#9179=CARTESIAN_POINT('Ctrl Pts',(98.4267824020307,0.785299093422799,1.59704971862112));
#9180=CARTESIAN_POINT('Ctrl Pts',(98.4396543716882,0.622084332889818,1.66507691792306));
#9181=CARTESIAN_POINT('Ctrl Pts',(98.4444369679918,0.559425251202567,1.68716191560871));
#9182=CARTESIAN_POINT('Ctrl Pts',(98.4500171997923,0.482445674826527,1.7095320726339));
#9183=CARTESIAN_POINT('Ctrl Pts',(98.45096870659,0.469175784994432,1.71322148266652));
#9184=CARTESIAN_POINT('Ctrl Pts',(98.4524546603536,0.448204245114866,1.71879022078136));
#9185=CARTESIAN_POINT('Ctrl Pts',(98.4529946289523,0.440530952882375,1.72077289440693));
#9186=CARTESIAN_POINT('Ctrl Pts',(98.4540196554321,0.425858955921624,1.72445936167206));
#9187=CARTESIAN_POINT('Ctrl Pts',(98.4545051697931,0.418862844188094,1.72617202500167));
#9188=CARTESIAN_POINT('Ctrl Pts',(98.4556791516275,0.401837539283828,1.73023025492238));
#9189=CARTESIAN_POINT('Ctrl Pts',(98.4563651303312,0.391797807747294,1.73253127926466));
#9190=CARTESIAN_POINT('Ctrl Pts',(98.4578326756743,0.370137305477898,1.73729776906998));
#9191=CARTESIAN_POINT('Ctrl Pts',(98.458612741806,0.358510606196195,1.73973426879071));
#9192=CARTESIAN_POINT('Ctrl Pts',(98.4669475181434,0.233184267069116,1.76468796792731));
#9193=CARTESIAN_POINT('Ctrl Pts',(98.4739989313469,0.11755406777982,1.77614329398991));
#9194=CARTESIAN_POINT('Ctrl Pts',(98.4811171398043,0.00162354587747538,
1.77624925801498));
#9195=CARTESIAN_POINT('Ctrl Pts',(98.4812164250559,0.00162964136512414,
1.77624925243307));
#9196=CARTESIAN_POINT('Ctrl Pts',(98.4854530653849,-0.0614205339738133,
1.77630709857919));
#9197=CARTESIAN_POINT('Ctrl Pts',(98.4896897057139,-0.124559988590764,1.7730036213554));
#9198=CARTESIAN_POINT('Ctrl Pts',(98.4939263460429,-0.187397282201051,1.76633697836049));
#9199=CARTESIAN_POINT('Ctrl Pts',(98.4981600988292,-0.250191748156839,1.75967487911128));
#9200=CARTESIAN_POINT('Ctrl Pts',(98.5023938516155,-0.312683948257245,1.74965421013642));
#9201=CARTESIAN_POINT('Ctrl Pts',(98.5066276044018,-0.374485080126635,1.73632513869452));
#9202=CARTESIAN_POINT('Ctrl Pts',(98.5108600832926,-0.436267616631049,1.72300007784176));
#9203=CARTESIAN_POINT('Ctrl Pts',(98.5150925621835,-0.497358992103221,1.70636869804803));
#9204=CARTESIAN_POINT('Ctrl Pts',(98.5193250410744,-0.557380291560129,1.68653232197914));
#9205=CARTESIAN_POINT('Ctrl Pts',(98.5236537296518,-0.618765952317672,1.66624503958037));
#9206=CARTESIAN_POINT('Ctrl Pts',(98.5279824182292,-0.679031739625796,1.64260538592702));
#9207=CARTESIAN_POINT('Ctrl Pts',(98.5323111068066,-0.737790779831893,1.61577499290435));
#9208=CARTESIAN_POINT('Ctrl Pts',(98.5365485336318,-0.795311003045761,1.58951026512515));
#9209=CARTESIAN_POINT('Ctrl Pts',(98.540785960457,-0.85138696102605,1.56018834574077));
#9210=CARTESIAN_POINT('Ctrl Pts',(98.5450233872823,-0.905680318337323,1.52800759928621));
#9211=CARTESIAN_POINT('Ctrl Pts',(98.5493977067357,-0.961727655288556,1.49478723441652));
#9212=CARTESIAN_POINT('Ctrl Pts',(98.5537720261892,-1.01587472029036,1.45852045930447));
#9213=CARTESIAN_POINT('Ctrl Pts',(98.5581463456427,-1.06778385824547,1.41947232962478));
#9214=CARTESIAN_POINT('Ctrl Pts',(98.5625206650961,-1.1196929962006,1.38042419994509));
#9215=CARTESIAN_POINT('Ctrl Pts',(98.5668949845496,-1.16936380077856,1.33859516044597));
#9216=CARTESIAN_POINT('Ctrl Pts',(98.571269304003,-1.21650027826686,1.29429175052484));
#9217=CARTESIAN_POINT('Ctrl Pts',(98.5755681123442,-1.26282306853283,1.25075312237103));
#9218=CARTESIAN_POINT('Ctrl Pts',(98.5798669206853,-1.3068998404826,1.20463586732403));
#9219=CARTESIAN_POINT('Ctrl Pts',(98.5841657290265,-1.34843003259545,1.15620089504144));
#9220=CARTESIAN_POINT('Ctrl Pts',(98.5885929911513,-1.39120119892496,1.10631862505256));
#9221=CARTESIAN_POINT('Ctrl Pts',(98.5930202532761,-1.43127069973378,1.05397820182919));
#9222=CARTESIAN_POINT('Ctrl Pts',(98.5974475154009,-1.46834877583047,0.999507846400997));
#9223=CARTESIAN_POINT('Ctrl Pts',(98.6017345078096,-1.5042521007911,0.946763284720955));
#9224=CARTESIAN_POINT('Ctrl Pts',(98.6060215002182,-1.53735042392031,0.892022197397326));
#9225=CARTESIAN_POINT('Ctrl Pts',(98.6103084926268,-1.56742121352955,0.83561642030153));
#9226=CARTESIAN_POINT('Ctrl Pts',(98.6145928647598,-1.59747362341002,0.779245119283622));
#9227=CARTESIAN_POINT('Ctrl Pts',(98.6188772368928,-1.62450193288729,0.721211590003397));
#9228=CARTESIAN_POINT('Ctrl Pts',(98.6231616090258,-1.64832841992064,0.661874219608161));
#9229=CARTESIAN_POINT('Ctrl Pts',(98.6274449047247,-1.67214892062964,0.602551757526726));
#9230=CARTESIAN_POINT('Ctrl Pts',(98.6317282004237,-1.69276900815509,0.54192657205303));
#9231=CARTESIAN_POINT('Ctrl Pts',(98.6360114961226,-1.71005899179161,0.480377254970144));
#9232=CARTESIAN_POINT('Ctrl Pts',(98.6402952574559,-1.72735085501084,0.418821246901651));
#9233=CARTESIAN_POINT('Ctrl Pts',(98.644579018789,-1.7413117627366,0.356341393772886));
#9234=CARTESIAN_POINT('Ctrl Pts',(98.6488627801223,-1.75186235659193,0.293329756513333));
#9235=CARTESIAN_POINT('Ctrl Pts',(98.6531512994025,-1.76242466892624,0.230248132620194));
#9236=CARTESIAN_POINT('Ctrl Pts',(98.6574398186828,-1.7695690292107,0.166634044264517));
#9237=CARTESIAN_POINT('Ctrl Pts',(98.6617283379631,-1.77326770929479,0.102886800282689));
#9238=CARTESIAN_POINT('Ctrl Pts',(98.6660197376141,-1.77696887358597,0.0390967406608165));
#9239=CARTESIAN_POINT('Ctrl Pts',(98.6703111372652,-1.7772197523833,-0.0248261489702147));
#9240=CARTESIAN_POINT('Ctrl Pts',(98.6746025369162,-1.77404474419002,-0.0884833776015348));
#9241=CARTESIAN_POINT('Ctrl Pts',(98.6789011723523,-1.77086438257393,-0.152247939517972));
#9242=CARTESIAN_POINT('Ctrl Pts',(98.6831998077884,-1.7642466664396,-0.215745447224884));
#9243=CARTESIAN_POINT('Ctrl Pts',(98.6874984432244,-1.75426757065288,-0.27858455279439));
#9244=CARTESIAN_POINT('Ctrl Pts',(98.688472302157,-1.75200679936507,-0.292820797105429));
#9245=CARTESIAN_POINT('Ctrl Pts',(98.6894461610895,-1.74957370910265,-0.307023303107869));
#9246=CARTESIAN_POINT('Ctrl Pts',(98.6904200200221,-1.74696953940082,-0.321187625704485));
#9247=CARTESIAN_POINT('Ctrl Pts',(98.6947188303473,-1.73547420755271,-0.383711810874786));
#9248=CARTESIAN_POINT('Ctrl Pts',(98.6990176406726,-1.72059461319993,-0.44574538270941));
#9249=CARTESIAN_POINT('Ctrl Pts',(98.7033164509978,-1.7023871991581,-0.506894354518425));
#9250=CARTESIAN_POINT('Ctrl Pts',(98.7077437128746,-1.68363573445878,-0.569870501688007));
#9251=CARTESIAN_POINT('Ctrl Pts',(98.7121709747514,-1.66135438932414,-0.631907792220913));
#9252=CARTESIAN_POINT('Ctrl Pts',(98.7165982366282,-1.63566203412561,-0.692584848679265));
#9253=CARTESIAN_POINT('Ctrl Pts',(98.7208852309857,-1.61078368158352,-0.751339493402278));
#9254=CARTESIAN_POINT('Ctrl Pts',(98.7251722253433,-1.58270745083389,-0.808818307680883));
#9255=CARTESIAN_POINT('Ctrl Pts',(98.7294592197008,-1.55159167589601,-0.864654459185978));
#9256=CARTESIAN_POINT('Ctrl Pts',(98.7337435937645,-1.52049491952074,-0.92045648255688));
#9257=CARTESIAN_POINT('Ctrl Pts',(98.7380279678283,-1.48636254800156,-0.974617394987629));
#9258=CARTESIAN_POINT('Ctrl Pts',(98.7423123418921,-1.44939949033832,-1.02679364037134));
#9259=CARTESIAN_POINT('Ctrl Pts',(98.7465956395009,-1.41244571969531,-1.0789567764));
#9260=CARTESIAN_POINT('Ctrl Pts',(98.7508789371096,-1.37266296594167,-1.12913582427183));
#9261=CARTESIAN_POINT('Ctrl Pts',(98.7551622347184,-1.33029916432395,-1.17701665064646));
#9262=CARTESIAN_POINT('Ctrl Pts',(98.7594459979375,-1.28793075760369,-1.22490268184469));
#9263=CARTESIAN_POINT('Ctrl Pts',(98.7637297611566,-1.24298108247334,-1.27048962054459));
#9264=CARTESIAN_POINT('Ctrl Pts',(98.7680135243757,-1.19573666601708,-1.31349833956589));
#9265=CARTESIAN_POINT('Ctrl Pts',(98.772302045495,-1.14843977602159,-1.35655482761206));
#9266=CARTESIAN_POINT('Ctrl Pts',(98.7765905666143,-1.0988434344109,-1.39702704480607));
#9267=CARTESIAN_POINT('Ctrl Pts',(98.7808790877336,-1.04726823442091,-1.43467533179912));
#9268=CARTESIAN_POINT('Ctrl Pts',(98.7851704891983,-0.99565839442585,-1.4723489049152));
#9269=CARTESIAN_POINT('Ctrl Pts',(98.7894618906631,-0.942067474509896,-1.50719450071351));
#9270=CARTESIAN_POINT('Ctrl Pts',(98.7937532921278,-0.886843623844741,-1.53901671509634));
#9271=CARTESIAN_POINT('Ctrl Pts',(98.798051929325,-0.831526660240488,-1.57089258491742));
#9272=CARTESIAN_POINT('Ctrl Pts',(98.8023505665221,-0.774571723567137,-1.59973468013227));
#9273=CARTESIAN_POINT('Ctrl Pts',(98.8066492037192,-0.716348904436194,-1.62539481653322));
#9274=CARTESIAN_POINT('Ctrl Pts',(98.8076230478266,-0.703158689322715,-1.6312080479092));
#9275=CARTESIAN_POINT('Ctrl Pts',(98.8085968919339,-0.689903467078543,-1.63685817102858));
#9276=CARTESIAN_POINT('Ctrl Pts',(98.8095707360413,-0.676587645183508,-1.64234381932805));
#9277=CARTESIAN_POINT('Ctrl Pts',(98.813869548981,-0.617807983189047,-1.66655896394362));
#9278=CARTESIAN_POINT('Ctrl Pts',(98.8181683619208,-0.557607015386957,-1.68766382635497));
#9279=CARTESIAN_POINT('Ctrl Pts',(98.8224671748606,-0.49634646777098,-1.7054923765386));
#9280=CARTESIAN_POINT('Ctrl Pts',(98.8268944364106,-0.433255453858138,-1.72385364413176));
#9281=CARTESIAN_POINT('Ctrl Pts',(98.8313216979606,-0.369040983373696,-1.73873937573369));
#9282=CARTESIAN_POINT('Ctrl Pts',(98.8357489595106,-0.304121627727075,-1.75002117074298));
#9283=CARTESIAN_POINT('Ctrl Pts',(98.8400359565544,-0.241259047189839,-1.76094553590823));
#9284=CARTESIAN_POINT('Ctrl Pts',(98.8443229535983,-0.177736118936162,-1.76849082743003));
#9285=CARTESIAN_POINT('Ctrl Pts',(98.8486099506421,-0.113946952508602,-1.77259136704261));
#9286=CARTESIAN_POINT('Ctrl Pts',(98.8528943274113,-0.0501967749438444,
-1.77668940034597));
#9287=CARTESIAN_POINT('Ctrl Pts',(98.8571787041804,0.0138188162689568,-1.77734682486678));
#9288=CARTESIAN_POINT('Ctrl Pts',(98.8614630809496,0.0777000290380064,-1.77454973669027));
#9289=CARTESIAN_POINT('Ctrl Pts',(98.8657463812783,0.141565191790422,-1.77175335127611));
#9290=CARTESIAN_POINT('Ctrl Pts',(98.870029681607,0.205295539914834,-1.76550419818667));
#9291=CARTESIAN_POINT('Ctrl Pts',(98.8743129819358,0.268492709345181,-1.75584046186676));
#9292=CARTESIAN_POINT('Ctrl Pts',(98.878596747885,0.331696748688168,-1.74617567504056));
#9293=CARTESIAN_POINT('Ctrl Pts',(98.8828805138343,0.39436699676,-1.73309564767349));
#9294=CARTESIAN_POINT('Ctrl Pts',(98.8871642797835,0.456113602137702,-1.71668996747956));
#9295=CARTESIAN_POINT('Ctrl Pts',(98.8914528036302,0.517928788296557,-1.70026606580841));
#9296=CARTESIAN_POINT('Ctrl Pts',(98.8957413274769,0.578817797915282,-1.68050927369018));
#9297=CARTESIAN_POINT('Ctrl Pts',(98.9000298513236,0.638405494324399,-1.65755919572015));
#9298=CARTESIAN_POINT('Ctrl Pts',(98.9043212555173,0.698033212253346,-1.63459370354457));
#9299=CARTESIAN_POINT('Ctrl Pts',(98.908612659711,0.756357419068994,-1.60843086550882));
#9300=CARTESIAN_POINT('Ctrl Pts',(98.9129040639047,0.813025244011015,-1.5792574252163));
#9301=CARTESIAN_POINT('Ctrl Pts',(98.9172027038082,0.869788616219608,-1.55003479576787));
#9302=CARTESIAN_POINT('Ctrl Pts',(98.9215013437118,0.924889603182745,-1.51779169480434));
#9303=CARTESIAN_POINT('Ctrl Pts',(98.9257999836153,0.978003133856311,-1.48275889229073));
#9304=CARTESIAN_POINT('Ctrl Pts',(98.9267738064304,0.990035583448879,-1.47482248842178));
#9305=CARTESIAN_POINT('Ctrl Pts',(98.9277476292454,1.00196616811946,-1.46674307731022));
#9306=CARTESIAN_POINT('Ctrl Pts',(98.9287214520604,1.01379135144946,-1.45852362278651));
#9307=CARTESIAN_POINT('Ctrl Pts',(98.9330204332438,1.06599411343148,-1.42223850008274));
#9308=CARTESIAN_POINT('Ctrl Pts',(98.9373194144271,1.11635265359479,-1.38307333437165));
#9309=CARTESIAN_POINT('Ctrl Pts',(98.9416183956104,1.16453139310864,-1.34124222158581));
#9310=CARTESIAN_POINT('Ctrl Pts',(98.9459097161208,1.2126242793583,-1.29948565075798));
#9311=CARTESIAN_POINT('Ctrl Pts',(98.9502010366311,1.25854470208939,-1.2550728955287));
#9312=CARTESIAN_POINT('Ctrl Pts',(98.9544923571415,1.30198733371713,-1.20826033839573));
#9313=CARTESIAN_POINT('Ctrl Pts',(98.9587793843407,1.34538650256142,-1.16149461553492));
#9314=CARTESIAN_POINT('Ctrl Pts',(98.96306641154,1.38631245406923,-1.11233421824034));
#9315=CARTESIAN_POINT('Ctrl Pts',(98.9673534387392,1.42449525816556,-1.06107366472071));
#9316=CARTESIAN_POINT('Ctrl Pts',(98.9716377202399,1.46265360744384,-1.00984594188335));
#9317=CARTESIAN_POINT('Ctrl Pts',(98.9759220017406,1.49807199391404,-0.956521134085841));
#9318=CARTESIAN_POINT('Ctrl Pts',(98.9802062832412,1.53052079063424,-0.901426742412457));
#9319=CARTESIAN_POINT('Ctrl Pts',(98.9844893630292,1.56296048568047,-0.846347804353431));
#9320=CARTESIAN_POINT('Ctrl Pts',(98.988772442817,1.59243198974081,-0.789500702131185));
#9321=CARTESIAN_POINT('Ctrl Pts',(98.9930555226049,1.61875011542024,-0.731240129045819));
#9322=CARTESIAN_POINT('Ctrl Pts',(98.9973414405387,1.64508568057823,-0.672940950095153));
#9323=CARTESIAN_POINT('Ctrl Pts',(99.0016273584724,1.66826348222424,-0.613226887845016));
#9324=CARTESIAN_POINT('Ctrl Pts',(99.0059132764061,1.68814583070561,-0.552474177470106));
#9325=CARTESIAN_POINT('Ctrl Pts',(99.0102006152251,1.70803477066555,-0.49170132610487));
#9326=CARTESIAN_POINT('Ctrl Pts',(99.0144879540441,1.72462594499934,-0.429889626563904));
#9327=CARTESIAN_POINT('Ctrl Pts',(99.0187752928631,1.7378318986038,-0.367429387359163));
#9328=CARTESIAN_POINT('Ctrl Pts',(99.0230691702742,1.75105799252098,-0.304873890455651));
#9329=CARTESIAN_POINT('Ctrl Pts',(99.0273630476853,1.76088847299791,-0.241668376698973));
#9330=CARTESIAN_POINT('Ctrl Pts',(99.0316569250965,1.76728741874363,-0.178211228744057));
#9331=CARTESIAN_POINT('Ctrl Pts',(99.0345990986562,1.77167198941965,-0.13473026154056));
#9332=CARTESIAN_POINT('Ctrl Pts',(99.037541272216,1.77444653737116,-0.0911312814132852));
#9333=CARTESIAN_POINT('Ctrl Pts',(99.0404834457757,1.77561363837197,-0.0475422940912327));
#9334=CARTESIAN_POINT('Origin',(88.3562164250559,0.,0.));
#9335=CARTESIAN_POINT('',(99.9383713772532,1.77277786422444,-0.0474589613121508));
#9336=CARTESIAN_POINT('',(99.7906304259994,1.77562736014833,-0.0475451276261121));
#9337=CARTESIAN_POINT('',(88.3562164250559,1.77561363837197,-0.0475422940912398));
#9338=CARTESIAN_POINT('',(99.3790868291567,-0.00134908208039473,1.77778173587435));
#9339=CARTESIAN_POINT('Ctrl Pts',(99.3790868291567,-0.00134908208039473,
1.77778173587435));
#9340=CARTESIAN_POINT('Ctrl Pts',(99.3849459429476,-0.0883230632624573,
1.77851575880056));
#9341=CARTESIAN_POINT('Ctrl Pts',(99.4305219620782,-0.764095661216901,1.73316171652182));
#9342=CARTESIAN_POINT('Ctrl Pts',(99.5158148865485,-1.91281695310219,0.866461694035085));
#9343=CARTESIAN_POINT('Ctrl Pts',(99.6349656025676,-1.76465526215908,-1.13813616919857));
#9344=CARTESIAN_POINT('Ctrl Pts',(99.7541163185868,0.000461911234235865,
-2.10006451370548));
#9345=CARTESIAN_POINT('Ctrl Pts',(99.8552515768152,1.49850875722623,-1.28264712973566));
#9346=CARTESIAN_POINT('Ctrl Pts',(99.9166699297041,1.76334219989321,-0.371393921105317));
#9347=CARTESIAN_POINT('Ctrl Pts',(99.9383713772532,1.77277786422444,-0.0474589613121508));
#9348=CARTESIAN_POINT('Ctrl Pts',(99.3782063185287,-0.00140217910956735,
1.77624944655692));
#9349=CARTESIAN_POINT('Ctrl Pts',(99.3685348291268,0.154290094078351,1.77637235072075));
#9350=CARTESIAN_POINT('Ctrl Pts',(99.3592174787437,0.309321614980016,1.75602653963719));
#9351=CARTESIAN_POINT('Ctrl Pts',(99.3472577925782,0.489394120042289,1.70777661516411));
#9352=CARTESIAN_POINT('Ctrl Pts',(99.3452660430548,0.518851342200709,1.69905876162217));
#9353=CARTESIAN_POINT('Ctrl Pts',(99.3422376731009,0.562731298362937,1.68482498703638));
#9354=CARTESIAN_POINT('Ctrl Pts',(99.3412195560868,0.577333250838938,1.67987738943743));
#9355=CARTESIAN_POINT('Ctrl Pts',(99.3393636079286,0.603667558597018,1.67057060461596));
#9356=CARTESIAN_POINT('Ctrl Pts',(99.3385279745531,0.615421877887082,1.66627625702889));
#9357=CARTESIAN_POINT('Ctrl Pts',(99.3367120993374,0.640737028222907,1.65672316751608));
#9358=CARTESIAN_POINT('Ctrl Pts',(99.3357304632278,0.654280522423058,1.65142137843329));
#9359=CARTESIAN_POINT('Ctrl Pts',(99.3330079721719,0.691443889802688,1.63634434706927));
#9360=CARTESIAN_POINT('Ctrl Pts',(99.3312556571195,0.714919401590681,1.62622495542015));
#9361=CARTESIAN_POINT('Ctrl Pts',(99.3186330643329,0.880800968754984,1.5504338359959));
#9362=CARTESIAN_POINT('Ctrl Pts',(99.3071143631717,1.01415424533639,1.46667224023185));
#9363=CARTESIAN_POINT('Ctrl Pts',(99.292198655096,1.17162133479598,1.33591326794866));
#9364=CARTESIAN_POINT('Ctrl Pts',(99.288728587195,1.20723939567059,1.30381533076926));
#9365=CARTESIAN_POINT('Ctrl Pts',(99.2839139085717,1.25567423697466,1.25647845770651));
#9366=CARTESIAN_POINT('Ctrl Pts',(99.2825177311901,1.26959932237344,1.24240634859454));
#9367=CARTESIAN_POINT('Ctrl Pts',(99.2801075291702,1.29347094434881,1.21746208974287));
#9368=CARTESIAN_POINT('Ctrl Pts',(99.2790872479893,1.30352268678777,1.20669369104589));
#9369=CARTESIAN_POINT('Ctrl Pts',(99.2775470268664,1.31863112074085,1.19009894334054));
#9370=CARTESIAN_POINT('Ctrl Pts',(99.2770203539084,1.32378547008393,1.18436293522051));
#9371=CARTESIAN_POINT('Ctrl Pts',(99.2760645086134,1.33312098478529,1.17383683860203));
#9372=CARTESIAN_POINT('Ctrl Pts',(99.2756344966678,1.33731394811641,1.16905769383451));
#9373=CARTESIAN_POINT('Ctrl Pts',(99.2746272215611,1.34711931762362,1.15775973024393));
#9374=CARTESIAN_POINT('Ctrl Pts',(99.2740515276798,1.35271014090362,1.15122253769098));
#9375=CARTESIAN_POINT('Ctrl Pts',(99.272345371931,1.36923069168006,1.13161899441757));
#9376=CARTESIAN_POINT('Ctrl Pts',(99.2712243977414,1.38002053471065,1.11843534091929));
#9377=CARTESIAN_POINT('Ctrl Pts',(99.261236343838,1.47536863006348,0.998452377114076));
#9378=CARTESIAN_POINT('Ctrl Pts',(99.2530512342777,1.54758089085957,0.882396668867394));
#9379=CARTESIAN_POINT('Ctrl Pts',(99.2393878065869,1.64234494390321,0.681959696256119));
#9380=CARTESIAN_POINT('Ctrl Pts',(99.2340621501052,1.67324281528213,0.602181059079847));
#9381=CARTESIAN_POINT('Ctrl Pts',(99.2268803999771,1.70585656694848,0.495768337278834));
#9382=CARTESIAN_POINT('Ctrl Pts',(99.2251960080795,1.71289347520407,0.470880773358365));
#9383=CARTESIAN_POINT('Ctrl Pts',(99.2225428039142,1.72301280476698,0.43185635354207));
#9384=CARTESIAN_POINT('Ctrl Pts',(99.2215861024424,1.72647027081705,0.417819839986028));
#9385=CARTESIAN_POINT('Ctrl Pts',(99.2197906095763,1.73260120769771,0.391553072020312));
#9386=CARTESIAN_POINT('Ctrl Pts',(99.2189532553555,1.73531746886852,0.379333654603007));
#9387=CARTESIAN_POINT('Ctrl Pts',(99.217068072029,1.7411124427657,0.351898427725253));
#9388=CARTESIAN_POINT('Ctrl Pts',(99.2160180766663,1.74412125401575,0.336669075429469));
#9389=CARTESIAN_POINT('Ctrl Pts',(99.2133033188218,1.75133931929291,0.297436497642581));
#9390=CARTESIAN_POINT('Ctrl Pts',(99.2116294618974,1.7552547924634,0.273383233761641));
#9391=CARTESIAN_POINT('Ctrl Pts',(99.2030565709261,1.77261059972131,0.150926969981673));
#9392=CARTESIAN_POINT('Ctrl Pts',(99.195924614015,1.77826940326188,0.0516452116294196));
#9393=CARTESIAN_POINT('Ctrl Pts',(99.1886897654568,1.7756136354609,-0.0475424028141329));
#9394=CARTESIAN_POINT('',(99.2312164566968,-0.000376088333153419,1.7759924949984));
#9395=CARTESIAN_POINT('Ctrl Pts',(99.0404834457757,1.77561363837197,-0.0475422940912327));
#9396=CARTESIAN_POINT('Ctrl Pts',(99.0429463532103,1.77659062415254,-0.0110537461648616));
#9397=CARTESIAN_POINT('Ctrl Pts',(99.0454092606449,1.77644140601071,0.025427782505673));
#9398=CARTESIAN_POINT('Ctrl Pts',(99.0478721680795,1.77517361646096,0.0618279380290967));
#9399=CARTESIAN_POINT('Ctrl Pts',(99.0521709862975,1.77296078591098,0.125361650056849));
#9400=CARTESIAN_POINT('Ctrl Pts',(99.0564698045155,1.7673283209483,0.188905764324683));
#9401=CARTESIAN_POINT('Ctrl Pts',(99.0607686227335,1.75827434492677,0.252062274988406));
#9402=CARTESIAN_POINT('Ctrl Pts',(99.0651958836237,1.74894984877258,0.317105813804496));
#9403=CARTESIAN_POINT('Ctrl Pts',(99.0696231445139,1.73599602715012,0.381737676937767));
#9404=CARTESIAN_POINT('Ctrl Pts',(99.0740504054041,1.71946874504975,0.445523621480441));
#9405=CARTESIAN_POINT('Ctrl Pts',(99.0783374074591,1.70346505923033,0.507288781048526));
#9406=CARTESIAN_POINT('Ctrl Pts',(99.0826244095141,1.68411109550379,0.568260292570386));
#9407=CARTESIAN_POINT('Ctrl Pts',(99.0869114115691,1.66150974684009,0.628052086737548));
#9408=CARTESIAN_POINT('Ctrl Pts',(99.0911957932383,1.63892221301767,0.687807333787172));
#9409=CARTESIAN_POINT('Ctrl Pts',(99.0954801749075,1.61309140837735,0.746383823106717));
#9410=CARTESIAN_POINT('Ctrl Pts',(99.0997645565767,1.58416972777763,0.803411685310175));
#9411=CARTESIAN_POINT('Ctrl Pts',(99.1040478616877,1.55525531447471,0.860425217834618));
#9412=CARTESIAN_POINT('Ctrl Pts',(99.1083311667986,1.52325179482111,0.915890446506549));
#9413=CARTESIAN_POINT('Ctrl Pts',(99.1126144719096,1.48835841589744,0.969460307762655));
#9414=CARTESIAN_POINT('Ctrl Pts',(99.1168982425165,1.45346124487328,1.02303599081944));
#9415=CARTESIAN_POINT('Ctrl Pts',(99.1211820131233,1.41567386897964,1.07471547726131));
#9416=CARTESIAN_POINT('Ctrl Pts',(99.1254657837301,1.37523883859957,1.12418067912027));
#9417=CARTESIAN_POINT('Ctrl Pts',(99.129754312023,1.33475889984356,1.17370081853858));
#9418=CARTESIAN_POINT('Ctrl Pts',(99.1340428403159,1.2916257609992,1.22100137764623));
#9419=CARTESIAN_POINT('Ctrl Pts',(99.1383313686088,1.24612145243364,1.2657983205411));
#9420=CARTESIAN_POINT('Ctrl Pts',(99.1426227771303,1.2005865826129,1.31062534961564));
#9421=CARTESIAN_POINT('Ctrl Pts',(99.1469141856517,1.15267775279318,1.35294508455562));
#9422=CARTESIAN_POINT('Ctrl Pts',(99.1512055941731,1.10271073464048,1.39251323089177));
#9423=CARTESIAN_POINT('Ctrl Pts',(99.1555042381955,1.05265946992754,1.43214809083917));
#9424=CARTESIAN_POINT('Ctrl Pts',(99.1598028822179,1.00054350676621,1.46902181997348));
#9425=CARTESIAN_POINT('Ctrl Pts',(99.1641015262402,0.946707238453464,1.50293362034383));
#9426=CARTESIAN_POINT('Ctrl Pts',(99.1650753121931,0.934511531722722,1.51061577189315));
#9427=CARTESIAN_POINT('Ctrl Pts',(99.1660490981459,0.92222763750181,1.51814611481939));
#9428=CARTESIAN_POINT('Ctrl Pts',(99.1670228840987,0.909859714797821,1.52552265204029));
#9429=CARTESIAN_POINT('Ctrl Pts',(99.1714716133702,0.853357010482439,1.55922227253753));
#9430=CARTESIAN_POINT('Ctrl Pts',(99.1759203426416,0.794882235523169,1.58983725820357));
#9431=CARTESIAN_POINT('Ctrl Pts',(99.180369071913,0.734792781678399,1.61714057227358));
#9432=CARTESIAN_POINT('Ctrl Pts',(99.1848065217802,0.674855679932851,1.64437466093134));
#9433=CARTESIAN_POINT('Ctrl Pts',(99.1892439716474,0.613312456593282,1.66831359787621));
#9434=CARTESIAN_POINT('Ctrl Pts',(99.1936814215145,0.550545679536776,1.68877574510158));
#9435=CARTESIAN_POINT('Ctrl Pts',(99.1981122123532,0.487873093010735,1.70920718594705));
#9436=CARTESIAN_POINT('Ctrl Pts',(99.2025430031918,0.423981029782271,1.72617206002377));
#9437=CARTESIAN_POINT('Ctrl Pts',(99.2069737940304,0.359272284467834,1.73953657280129));
#9438=CARTESIAN_POINT('Ctrl Pts',(99.2113975132016,0.294666816141035,1.75287975543844));
#9439=CARTESIAN_POINT('Ctrl Pts',(99.2158212323728,0.229247702670285,1.7626339160979));
#9440=CARTESIAN_POINT('Ctrl Pts',(99.2202449515439,0.16343141159382,1.76871541979043));
#9441=CARTESIAN_POINT('Ctrl Pts',(99.2239021093813,0.109020054221916,1.77374309402368));
#9442=CARTESIAN_POINT('Ctrl Pts',(99.2275592672186,0.0543376437225603,1.77626153193324));
#9443=CARTESIAN_POINT('Ctrl Pts',(99.2312164250559,-0.000375670171088504,
1.77624996027359));
#9444=CARTESIAN_POINT('Ctrl Pts',(99.2312167715186,-0.000380248985858326,
1.77343075235475));
#9445=CARTESIAN_POINT('Ctrl Pts',(99.249535714385,-0.274007951532822,1.77394632845611));
#9446=CARTESIAN_POINT('Ctrl Pts',(99.307571562591,-1.14020838492317,1.58562537855393));
#9447=CARTESIAN_POINT('Ctrl Pts',(99.4053243161369,-2.08671183082761,0.235097532724869));
#9448=CARTESIAN_POINT('Ctrl Pts',(99.524475032156,-1.32822316119735,-1.62647487068021));
#9449=CARTESIAN_POINT('Ctrl Pts',(99.6436257481753,0.647387598188645,-1.99764857090965));
#9450=CARTESIAN_POINT('Ctrl Pts',(99.7323442127897,1.67669836196288,-0.910947872649348));
#9451=CARTESIAN_POINT('Ctrl Pts',(99.7813457720644,1.77332763342921,-0.185653457768005));
#9452=CARTESIAN_POINT('Ctrl Pts',(99.7906304259995,1.77562736014833,-0.0475451276259355));
#9453=CARTESIAN_POINT('Origin',(66.9212607628943,0.,0.));
#9454=CARTESIAN_POINT('',(33.4926516271063,2.69912154532077E-16,2.204));
#9455=CARTESIAN_POINT('Origin',(33.4926516271063,0.,0.));
#9456=CARTESIAN_POINT('',(90.3498698986825,-0.214101726762253,-2.19357617843498));
#9457=CARTESIAN_POINT('',(90.3498698986825,1.62325119196235,-1.49086269246796));
#9458=CARTESIAN_POINT('Origin',(90.3498698986825,0.,0.));
#9459=CARTESIAN_POINT('',(90.6260484068025,0.00185087634597349,2.20399922283488));
#9460=CARTESIAN_POINT('Ctrl Pts',(90.3498698986825,1.62325119196235,-1.49086269246796));
#9461=CARTESIAN_POINT('Ctrl Pts',(90.3895868040222,2.11930827345322,-0.950755777941539));
#9462=CARTESIAN_POINT('Ctrl Pts',(90.4690206147016,2.5208914807363,0.654645457688011));
#9463=CARTESIAN_POINT('Ctrl Pts',(90.5610799237519,1.20144938824896,2.06273780995529));
#9464=CARTESIAN_POINT('Ctrl Pts',(90.6134223274625,0.235399057971462,2.20457276789839));
#9465=CARTESIAN_POINT('Ctrl Pts',(90.6260478258334,0.00186055395922385,
2.2027266091469));
#9466=CARTESIAN_POINT('',(91.3760484068552,-0.00126552574240722,2.2039996366707));
#9467=CARTESIAN_POINT('Ctrl Pts',(90.6260484068025,0.00185087634597349,
2.20399922283488));
#9468=CARTESIAN_POINT('Ctrl Pts',(90.6300874787337,-0.0729039514327416,
2.20406200050787));
#9469=CARTESIAN_POINT('Ctrl Pts',(90.634126550665,-0.147719807169649,2.20031720231216));
#9470=CARTESIAN_POINT('Ctrl Pts',(90.6381656225962,-0.222177953843929,2.19277289221336));
#9471=CARTESIAN_POINT('Ctrl Pts',(90.6422034326244,-0.29661283800512,2.1852309391382));
#9472=CARTESIAN_POINT('Ctrl Pts',(90.6462412426525,-0.370689755210188,2.17389187899442));
#9473=CARTESIAN_POINT('Ctrl Pts',(90.6502790526807,-0.443993956851574,2.15881573235867));
#9474=CARTESIAN_POINT('Ctrl Pts',(90.6543169380162,-0.517299525655997,2.14373930454462));
#9475=CARTESIAN_POINT('Ctrl Pts',(90.6583548233517,-0.589831878086408,2.12492575105078));
#9476=CARTESIAN_POINT('Ctrl Pts',(90.6623927086872,-0.661186999955675,2.10248608820359));
#9477=CARTESIAN_POINT('Ctrl Pts',(90.6664347773491,-0.732616047094706,2.08002317743688));
#9478=CARTESIAN_POINT('Ctrl Pts',(90.670476846011,-0.802864967400653,2.05392680203279));
#9479=CARTESIAN_POINT('Ctrl Pts',(90.6745189146728,-0.871546247179227,2.02435746325292));
#9480=CARTESIAN_POINT('Ctrl Pts',(90.6785631757033,-0.940264778844592,1.99477208642507));
#9481=CARTESIAN_POINT('Ctrl Pts',(90.6826074367339,-1.00741354460176,1.9617102103385));
#9482=CARTESIAN_POINT('Ctrl Pts',(90.6866516977644,-1.07262878263828,1.92537879251225));
#9483=CARTESIAN_POINT('Ctrl Pts',(90.6907031775646,-1.13796042606586,1.88898252522707));
#9484=CARTESIAN_POINT('Ctrl Pts',(90.6947546573649,-1.20135124130891,1.84930531944377));
#9485=CARTESIAN_POINT('Ctrl Pts',(90.6988061371651,-1.26246612799149,1.80659770720384));
#9486=CARTESIAN_POINT('Ctrl Pts',(90.7016447736901,-1.30528577861491,1.77667496441006));
#9487=CARTESIAN_POINT('Ctrl Pts',(90.704483410215,-1.34698881701027,1.7452654959714));
#9488=CARTESIAN_POINT('Ctrl Pts',(90.70732204674,-1.38747039308724,1.71246661523848));
#9489=CARTESIAN_POINT('Ctrl Pts',(90.7114017643054,-1.44565092995657,1.6653277270162));
#9490=CARTESIAN_POINT('Ctrl Pts',(90.7154814818708,-1.50153452025124,1.61513293526345));
#9491=CARTESIAN_POINT('Ctrl Pts',(90.7195611994362,-1.5547836346165,1.56213438907435));
#9492=CARTESIAN_POINT('Ctrl Pts',(90.7236350692713,-1.60795642348694,1.50921180922406));
#9493=CARTESIAN_POINT('Ctrl Pts',(90.7277089391064,-1.65850190012224,1.45349378779541));
#9494=CARTESIAN_POINT('Ctrl Pts',(90.7317828089415,-1.70611547319863,1.3952727303693));
#9495=CARTESIAN_POINT('Ctrl Pts',(90.7358520916738,-1.75367543426419,1.33711722878705));
#9496=CARTESIAN_POINT('Ctrl Pts',(90.7399213744061,-1.79830975135764,1.27646465745508));
#9497=CARTESIAN_POINT('Ctrl Pts',(90.7439906571384,-1.83975172184307,1.21364311145224));
#9498=CARTESIAN_POINT('Ctrl Pts',(90.7480574630342,-1.88116846798516,1.1508598028263));
#9499=CARTESIAN_POINT('Ctrl Pts',(90.75212426893,-1.91939646253376,1.08591053571015));
#9500=CARTESIAN_POINT('Ctrl Pts',(90.7561910748258,-1.95421105246868,1.01915414065256));
#9501=CARTESIAN_POINT('Ctrl Pts',(90.7602567070635,-1.98901559510216,0.952417011127753));
#9502=CARTESIAN_POINT('Ctrl Pts',(90.7643223393013,-2.0204084694443,0.883874210752672));
#9503=CARTESIAN_POINT('Ctrl Pts',(90.768387971539,-2.0482107022416,0.813909650528229));
#9504=CARTESIAN_POINT('Ctrl Pts',(90.772453731708,-2.07601380987793,0.74394288876377));
#9505=CARTESIAN_POINT('Ctrl Pts',(90.7765194918769,-2.10022587761992,0.672554720968091));
#9506=CARTESIAN_POINT('Ctrl Pts',(90.7805852520459,-2.12071646269066,0.600148052461083));
#9507=CARTESIAN_POINT('Ctrl Pts',(90.7846552374533,-2.14122834208392,0.527666137154293));
#9508=CARTESIAN_POINT('Ctrl Pts',(90.7887252228607,-2.15801088618608,0.454164066194615));
#9509=CARTESIAN_POINT('Ctrl Pts',(90.7927952082681,-2.17098405606415,0.380058190696185));
#9510=CARTESIAN_POINT('Ctrl Pts',(90.7968673685232,-2.18396415831782,0.305912715796166));
#9511=CARTESIAN_POINT('Ctrl Pts',(90.8009395287782,-2.19313077453104,0.231163266298682));
#9512=CARTESIAN_POINT('Ctrl Pts',(90.8050116890333,-2.19845572220061,0.156231999037993));
#9513=CARTESIAN_POINT('Ctrl Pts',(90.8090911138956,-2.20379016941132,0.0811670567253429));
#9514=CARTESIAN_POINT('Ctrl Pts',(90.813170538758,-2.20526924949307,0.00592012497610547));
#9515=CARTESIAN_POINT('Ctrl Pts',(90.8172499636204,-2.20291694593774,-0.0690863901239109));
#9516=CARTESIAN_POINT('Ctrl Pts',(90.8203242299999,-2.20114424317238,-0.125611516924139));
#9517=CARTESIAN_POINT('Ctrl Pts',(90.8233984963795,-2.19719672128774,-0.182000103923053));
#9518=CARTESIAN_POINT('Ctrl Pts',(90.826472762759,-2.19110394319517,-0.23807458939287));
#9519=CARTESIAN_POINT('Ctrl Pts',(90.8305414997454,-2.18304025953379,-0.312288175614706));
#9520=CARTESIAN_POINT('Ctrl Pts',(90.8346102367318,-2.17118595693924,-0.386237671673184));
#9521=CARTESIAN_POINT('Ctrl Pts',(90.8386789737183,-2.15556753379367,-0.459504741275533));
#9522=CARTESIAN_POINT('Ctrl Pts',(90.8427416649012,-2.13997231832122,-0.53266294212804));
#9523=CARTESIAN_POINT('Ctrl Pts',(90.8468043560841,-2.12062418510459,-0.60514026552376));
#9524=CARTESIAN_POINT('Ctrl Pts',(90.850867047267,-2.09760134521141,-0.676523906870472));
#9525=CARTESIAN_POINT('Ctrl Pts',(90.8549249084732,-2.07460587628337,-0.747822682963042));
#9526=CARTESIAN_POINT('Ctrl Pts',(90.8589827696795,-2.04794452602362,-0.818029906979268));
#9527=CARTESIAN_POINT('Ctrl Pts',(90.8630406308857,-2.01774609217716,-0.8867450070363));
#9528=CARTESIAN_POINT('Ctrl Pts',(90.8670958721175,-1.98756715607173,-0.955415740910866));
#9529=CARTESIAN_POINT('Ctrl Pts',(90.8711511133492,-1.95385585989427,-1.02259582539034));
#9530=CARTESIAN_POINT('Ctrl Pts',(90.875206354581,-1.91678970801654,-1.08790312769193));
#9531=CARTESIAN_POINT('Ctrl Pts',(90.8792602957455,-1.87973543915321,-1.15318949316639));
#9532=CARTESIAN_POINT('Ctrl Pts',(90.88331423691,-1.8393286859202,-1.21660385243824));
#9533=CARTESIAN_POINT('Ctrl Pts',(90.8873681780745,-1.79579288744773,-1.2777886779089));
#9534=CARTESIAN_POINT('Ctrl Pts',(90.8914221373556,-1.75225689441882,-1.33897377680743));
#9535=CARTESIAN_POINT('Ctrl Pts',(90.8954760966367,-1.70559210734747,-1.39792893317653));
#9536=CARTESIAN_POINT('Ctrl Pts',(90.8995300559178,-1.65606433175256,-1.45432696774038));
#9537=CARTESIAN_POINT('Ctrl Pts',(90.903588151952,-1.6064860168781,-1.51078255215382));
#9538=CARTESIAN_POINT('Ctrl Pts',(90.9076462479862,-1.55403919597851,-1.5646754435487));
#9539=CARTESIAN_POINT('Ctrl Pts',(90.9117043440205,-1.49902838264026,-1.61571343623767));
#9540=CARTESIAN_POINT('Ctrl Pts',(90.9157645471804,-1.44398900548803,-1.66677792989327));
#9541=CARTESIAN_POINT('Ctrl Pts',(90.9198247503404,-1.38638335227213,-1.71498426556534));
#9542=CARTESIAN_POINT('Ctrl Pts',(90.9238849535004,-1.32654899637501,-1.76008061185176));
#9543=CARTESIAN_POINT('Ctrl Pts',(90.9279524456706,-1.26660722387395,-1.80525791658245));
#9544=CARTESIAN_POINT('Ctrl Pts',(90.9320199378409,-1.20442915406587,-1.8473138115681));
#9545=CARTESIAN_POINT('Ctrl Pts',(90.9360874300111,-1.14038090942948,-1.88604013250217));
#9546=CARTESIAN_POINT('Ctrl Pts',(90.9392661129335,-1.09032818580747,-1.91630416002727));
#9547=CARTESIAN_POINT('Ctrl Pts',(90.9424447958558,-1.0391339147687,-1.94453563114969));
#9548=CARTESIAN_POINT('Ctrl Pts',(90.9456234787781,-0.986981606041235,-1.97065555319449));
#9549=CARTESIAN_POINT('Ctrl Pts',(90.949697228417,-0.920144033992175,-2.00413043118519));
#9550=CARTESIAN_POINT('Ctrl Pts',(90.9537709780558,-0.851472863040309,-2.03426555142575));
#9551=CARTESIAN_POINT('Ctrl Pts',(90.9578447276947,-0.781335344783656,-2.06085687979341));
#9552=CARTESIAN_POINT('Ctrl Pts',(90.9619124935517,-0.711300848961369,-2.08740914913175));
#9553=CARTESIAN_POINT('Ctrl Pts',(90.9659802594088,-0.639804724761734,-2.11042779364493));
#9554=CARTESIAN_POINT('Ctrl Pts',(90.9700480252658,-0.567237476967494,-2.1297553016071));
#9555=CARTESIAN_POINT('Ctrl Pts',(90.9741110298079,-0.494755169047744,-2.14906018674492));
#9556=CARTESIAN_POINT('Ctrl Pts',(90.97817403435,-0.42120468736276,-2.16468239700842));
#9557=CARTESIAN_POINT('Ctrl Pts',(90.9822370388921,-0.346993562062258,-2.1765136038829));
#9558=CARTESIAN_POINT('Ctrl Pts',(90.9862974630882,-0.27282956700218,-2.18833729695643));
#9559=CARTESIAN_POINT('Ctrl Pts',(90.9903578872843,-0.198006231046259,-2.19637468937789));
#9560=CARTESIAN_POINT('Ctrl Pts',(90.9944183114804,-0.122941882356516,-2.20056840238213));
#9561=CARTESIAN_POINT('Ctrl Pts',(90.9984774678744,-0.0479009713020453,
-2.20476080596695));
#9562=CARTESIAN_POINT('Ctrl Pts',(91.0025366242683,0.0273803268527341,-2.20511188635905));
#9563=CARTESIAN_POINT('Ctrl Pts',(91.0065957806623,0.102479553979722,-2.20161621110858));
#9564=CARTESIAN_POINT('Ctrl Pts',(91.0106549801117,0.177579577683765,-2.19812049877951));
#9565=CARTESIAN_POINT('Ctrl Pts',(91.0147141795611,0.25249704984926,-2.19077797377606));
#9566=CARTESIAN_POINT('Ctrl Pts',(91.0187733790105,0.326812124591935,-2.17963525279339));
#9567=CARTESIAN_POINT('Ctrl Pts',(91.022836717627,0.401202978441364,-2.16848116957438));
#9568=CARTESIAN_POINT('Ctrl Pts',(91.0269000562434,0.474989735164241,-2.15351922299617));
#9569=CARTESIAN_POINT('Ctrl Pts',(91.0309633948599,0.547761015715058,-2.1348475050136));
#9570=CARTESIAN_POINT('Ctrl Pts',(91.0350288503013,0.620570206977919,-2.11616605986781));
#9571=CARTESIAN_POINT('Ctrl Pts',(91.0390943057426,0.692362412501551,-2.09377113684108));
#9572=CARTESIAN_POINT('Ctrl Pts',(91.043159761184,0.762742296738048,-2.06781048183018));
#9573=CARTESIAN_POINT('Ctrl Pts',(91.0472324618394,0.833247607837265,-2.04180356127697));
#9574=CARTESIAN_POINT('Ctrl Pts',(91.0513051624947,0.902335130804898,-2.01221840394449));
#9575=CARTESIAN_POINT('Ctrl Pts',(91.0553778631501,0.969630779096078,-1.97925040159893));
#9576=CARTESIAN_POINT('Ctrl Pts',(91.0585099736992,1.02138449923315,-1.95389635850409));
#9577=CARTESIAN_POINT('Ctrl Pts',(91.0616420842482,1.07207886378984,-1.92654256107378));
#9578=CARTESIAN_POINT('Ctrl Pts',(91.0647741947973,1.12155540262169,-1.89729530617933));
#9579=CARTESIAN_POINT('Ctrl Pts',(91.0688479806445,1.18590716176332,-1.85925480563181));
#9580=CARTESIAN_POINT('Ctrl Pts',(91.0729217664916,1.24844494575908,-1.8178635523109));
#9581=CARTESIAN_POINT('Ctrl Pts',(91.0769955523388,1.30879830848776,-1.77331976465035));
#9582=CARTESIAN_POINT('Ctrl Pts',(91.0810633696527,1.3690632470665,-1.72884123841652));
#9583=CARTESIAN_POINT('Ctrl Pts',(91.0851311869666,1.42714973775237,-1.68121962924715));
#9584=CARTESIAN_POINT('Ctrl Pts',(91.0891990042805,1.48271384986785,-1.63069789949275));
#9585=CARTESIAN_POINT('Ctrl Pts',(91.0932620830264,1.53821323579128,-1.58023502209931));
#9586=CARTESIAN_POINT('Ctrl Pts',(91.0973251617723,1.59119572955431,-1.52687905559947));
#9587=CARTESIAN_POINT('Ctrl Pts',(91.1013882405182,1.64134952364412,-1.47091391360379));
#9588=CARTESIAN_POINT('Ctrl Pts',(91.1054487528421,1.69147163835721,-1.41498412169177));
#9589=CARTESIAN_POINT('Ctrl Pts',(91.109509265166,1.73876828130666,-1.35644877928074));
#9590=CARTESIAN_POINT('Ctrl Pts',(91.1135697774898,1.7829646278059,-1.29562847143499));
#9591=CARTESIAN_POINT('Ctrl Pts',(91.1176290358398,1.82714732551904,-1.23482694621355));
#9592=CARTESIAN_POINT('Ctrl Pts',(91.1216882941898,1.86823134738425,-1.1717422424517));
#9593=CARTESIAN_POINT('Ctrl Pts',(91.1257475525398,1.9059833003935,-1.10672655096962));
#9594=CARTESIAN_POINT('Ctrl Pts',(91.1298068676916,1.94373578167153,-1.04170994971314));
#9595=CARTESIAN_POINT('Ctrl Pts',(91.1338661828434,1.97815586340892,-0.974762720713493));
#9596=CARTESIAN_POINT('Ctrl Pts',(91.1379254979952,2.00905532200643,-0.906263048522695));
#9597=CARTESIAN_POINT('Ctrl Pts',(91.1419889730131,2.03998644545502,-0.837693179894235));
#9598=CARTESIAN_POINT('Ctrl Pts',(91.146052448031,2.06738954448393,-0.767568127170326));
#9599=CARTESIAN_POINT('Ctrl Pts',(91.1501159230489,2.09112425233576,-0.696286838374254));
#9600=CARTESIAN_POINT('Ctrl Pts',(91.1541815265921,2.11487139287808,-0.624968211086075));
#9601=CARTESIAN_POINT('Ctrl Pts',(91.1582471301353,2.13494618808701,-0.552492601980794));
#9602=CARTESIAN_POINT('Ctrl Pts',(91.1623127336786,2.15125870146638,-0.47927236449139));
#9603=CARTESIAN_POINT('Ctrl Pts',(91.1663856001343,2.1676003559943,-0.40592132423925));
#9604=CARTESIAN_POINT('Ctrl Pts',(91.17045846659,2.18016622400246,-0.331823469819038));
#9605=CARTESIAN_POINT('Ctrl Pts',(91.1745313330457,2.18891792995835,-0.2573990984966));
#9606=CARTESIAN_POINT('Ctrl Pts',(91.1776625256359,2.19564618317733,-0.20018213777551));
#9607=CARTESIAN_POINT('Ctrl Pts',(91.1807937182261,2.20012116454199,-0.142772367545864));
#9608=CARTESIAN_POINT('Ctrl Pts',(91.1839249108164,2.20234638625319,-0.0853603828337333));
#9609=CARTESIAN_POINT('Ctrl Pts',(91.187997411325,2.20524056037039,-0.0106890458901615));
#9610=CARTESIAN_POINT('Ctrl Pts',(91.1920699118336,2.20433838784057,0.0642740422392719));
#9611=CARTESIAN_POINT('Ctrl Pts',(91.1961424123423,2.19960548666169,0.139110398776636));
#9612=CARTESIAN_POINT('Ctrl Pts',(91.2002089201829,2.19487954992769,0.213836633918954));
#9613=CARTESIAN_POINT('Ctrl Pts',(91.2042754280235,2.18633410587648,0.288436035025831));
#9614=CARTESIAN_POINT('Ctrl Pts',(91.2083419358642,2.17398674374528,0.362488121211967));
#9615=CARTESIAN_POINT('Ctrl Pts',(91.2124036752274,2.16165386040528,0.43645337227642));
#9616=CARTESIAN_POINT('Ctrl Pts',(91.2164654145906,2.14552799453576,0.509872114776402));
#9617=CARTESIAN_POINT('Ctrl Pts',(91.2205271539538,2.12567856202451,0.582328645139008));
#9618=CARTESIAN_POINT('Ctrl Pts',(91.2245863092188,2.10584175781765,0.654739078308608));
#9619=CARTESIAN_POINT('Ctrl Pts',(91.2286454644839,2.08228621371744,0.726188054632568));
#9620=CARTESIAN_POINT('Ctrl Pts',(91.232704619749,2.0551322121439,0.796271053478975));
#9621=CARTESIAN_POINT('Ctrl Pts',(91.2367625053054,2.02798670437495,0.866332130278421));
#9622=CARTESIAN_POINT('Ctrl Pts',(91.2408203908618,1.99724514638297,0.935027632873771));
#9623=CARTESIAN_POINT('Ctrl Pts',(91.2448782764182,1.96307684258466,1.00197071319866));
#9624=CARTESIAN_POINT('Ctrl Pts',(91.2489362049661,1.92890817678793,1.06891450275659));
#9625=CARTESIAN_POINT('Ctrl Pts',(91.2529941335141,1.89131291182923,1.13410540859003));
#9626=CARTESIAN_POINT('Ctrl Pts',(91.257052062062,1.85050668370051,1.19718044319967));
#9627=CARTESIAN_POINT('Ctrl Pts',(91.2611141386116,1.80965874357502,1.26031995290932));
#9628=CARTESIAN_POINT('Ctrl Pts',(91.2651762151612,1.76559354584184,1.32133887042383));
#9629=CARTESIAN_POINT('Ctrl Pts',(91.2692382917108,1.71857011781289,1.37990316695071));
#9630=CARTESIAN_POINT('Ctrl Pts',(91.2733024880002,1.67152215124388,1.43849802446381));
#9631=CARTESIAN_POINT('Ctrl Pts',(91.2773666842895,1.62151319824356,1.49463535323905));
#9632=CARTESIAN_POINT('Ctrl Pts',(91.2814308805788,1.56884088670155,1.5480162377099));
#9633=CARTESIAN_POINT('Ctrl Pts',(91.2855023412743,1.51607442787032,1.60149253598397));
#9634=CARTESIAN_POINT('Ctrl Pts',(91.2895738019698,1.46063545467096,1.65220222600835));
#9635=CARTESIAN_POINT('Ctrl Pts',(91.2936452626652,1.40285621719685,1.69988541786561));
#9636=CARTESIAN_POINT('Ctrl Pts',(91.2967887173887,1.35824657202552,1.73670020397874));
#9637=CARTESIAN_POINT('Ctrl Pts',(91.2999321721121,1.312242636158,1.7717117089801));
#9638=CARTESIAN_POINT('Ctrl Pts',(91.3030756268355,1.26500851005774,1.80481840346377));
#9639=CARTESIAN_POINT('Ctrl Pts',(91.3071951970518,1.20310709387826,1.84820549332355));
#9640=CARTESIAN_POINT('Ctrl Pts',(91.3113147672681,1.13885577516707,1.8884852462642));
#9641=CARTESIAN_POINT('Ctrl Pts',(91.3154343374845,1.07259506399885,1.9253975767839));
#9642=CARTESIAN_POINT('Ctrl Pts',(91.3195475167814,1.00643714677331,1.96225264314328));
#9643=CARTESIAN_POINT('Ctrl Pts',(91.3236606960783,0.938276428746113,1.9957504383066));
#9644=CARTESIAN_POINT('Ctrl Pts',(91.3277738753752,0.868483277122665,2.02567341823856));
#9645=CARTESIAN_POINT('Ctrl Pts',(91.3318810969693,0.798791216850553,2.05555305646138));
#9646=CARTESIAN_POINT('Ctrl Pts',(91.3359883185635,0.727471847580355,2.08186799348214));
#9647=CARTESIAN_POINT('Ctrl Pts',(91.3400955401576,0.654919597791209,2.10444679676845));
#9648=CARTESIAN_POINT('Ctrl Pts',(91.344199215925,0.582429983460193,2.12700610743129));
#9649=CARTESIAN_POINT('Ctrl Pts',(91.3483028916924,0.508710043147842,2.14583555337324));
#9650=CARTESIAN_POINT('Ctrl Pts',(91.3524065674598,0.434172636937849,2.16081237531962));
#9651=CARTESIAN_POINT('Ctrl Pts',(91.356508427657,0.359668207966178,2.17578257114026));
#9652=CARTESIAN_POINT('Ctrl Pts',(91.3606102878542,0.284347483751757,2.18690343172747));
#9653=CARTESIAN_POINT('Ctrl Pts',(91.3647121480514,0.208635661003606,2.19410281458221));
#9654=CARTESIAN_POINT('Ctrl Pts',(91.3684909009685,0.138887727795815,2.20073509546337));
#9655=CARTESIAN_POINT('Ctrl Pts',(91.3722696538855,0.0688082964965979,2.20403987268341));
#9656=CARTESIAN_POINT('Ctrl Pts',(91.3760484068025,-0.00126552476430762,
2.20399963667127));
#9657=CARTESIAN_POINT('',(92.1260484067482,-0.00117773768617704,2.20399968532982));
#9658=CARTESIAN_POINT('Ctrl Pts',(91.3760484068552,-0.00126552574240776,
2.2039996366707));
#9659=CARTESIAN_POINT('Ctrl Pts',(91.3805750013567,-0.0852074454640055,
2.2039514376336));
#9660=CARTESIAN_POINT('Ctrl Pts',(91.3851015958581,-0.168975608381795,2.19910358289283));
#9661=CARTESIAN_POINT('Ctrl Pts',(91.3896281903595,-0.252053052579413,2.18953996508066));
#9662=CARTESIAN_POINT('Ctrl Pts',(91.3941731607358,-0.335467752682458,2.17993752341424));
#9663=CARTESIAN_POINT('Ctrl Pts',(91.3987181311122,-0.418185860182198,2.16558108788022));
#9664=CARTESIAN_POINT('Ctrl Pts',(91.4032631014886,-0.499701398972763,2.14660534609058));
#9665=CARTESIAN_POINT('Ctrl Pts',(91.4078314961518,-0.581637060052887,2.12753180537567));
#9666=CARTESIAN_POINT('Ctrl Pts',(91.412399890815,-0.662357477674704,2.10379135432718));
#9667=CARTESIAN_POINT('Ctrl Pts',(91.4169682854782,-0.741370049144116,2.07556894615237));
#9668=CARTESIAN_POINT('Ctrl Pts',(91.4187209712703,-0.771683588499686,2.06474128841378));
#9669=CARTESIAN_POINT('Ctrl Pts',(91.4204736570625,-0.801745989238771,2.05325441876248));
#9670=CARTESIAN_POINT('Ctrl Pts',(91.4222263428546,-0.8315303725407,2.04112058427285));
#9671=CARTESIAN_POINT('Ctrl Pts',(91.4262994818301,-0.900747532304323,2.01292226464003));
#9672=CARTESIAN_POINT('Ctrl Pts',(91.4303726208057,-0.968662122249928,1.98114472878017));
#9673=CARTESIAN_POINT('Ctrl Pts',(91.4344457597813,-1.03487872486445,1.94592960428247));
#9674=CARTESIAN_POINT('Ctrl Pts',(91.4385129163849,-1.10099807267219,1.91076620155836));
#9675=CARTESIAN_POINT('Ctrl Pts',(91.4425800729885,-1.16542396652118,1.87217545668805));
#9676=CARTESIAN_POINT('Ctrl Pts',(91.4466472295922,-1.22778064353879,1.83034715050218));
#9677=CARTESIAN_POINT('Ctrl Pts',(91.4507096300371,-1.29006440026404,1.78856775860204));
#9678=CARTESIAN_POINT('Ctrl Pts',(91.4547720304821,-1.350283353155,1.74355859198948));
#9679=CARTESIAN_POINT('Ctrl Pts',(91.4588344309271,-1.40808750137832,1.69555465510911));
#9680=CARTESIAN_POINT('Ctrl Pts',(91.4628942545007,-1.46585498313863,1.64758116819868));
#9681=CARTESIAN_POINT('Ctrl Pts',(91.4669540780743,-1.52121033348808,1.59661698492927));
#9682=CARTESIAN_POINT('Ctrl Pts',(91.4710139016479,-1.57383474947358,1.54293881322281));
#9683=CARTESIAN_POINT('Ctrl Pts',(91.4750724617826,-1.62644278845851,1.48927734645136));
#9684=CARTESIAN_POINT('Ctrl Pts',(91.4791310219174,-1.67632124646478,1.43290390888715));
#9685=CARTESIAN_POINT('Ctrl Pts',(91.4831895820521,-1.72318766461713,1.37413255274422));
#9686=CARTESIAN_POINT('Ctrl Pts',(91.4872481904981,-1.77005464064554,1.31536049701439));
#9687=CARTESIAN_POINT('Ctrl Pts',(91.491306798944,-1.8139092093616,1.25419084043354));
#9688=CARTESIAN_POINT('Ctrl Pts',(91.4953654073899,-1.85450977849573,1.19096997504711));
#9689=CARTESIAN_POINT('Ctrl Pts',(91.4994281673881,-1.89515187796876,1.12768444101142));
#9690=CARTESIAN_POINT('Ctrl Pts',(91.5034909273863,-1.93253307243781,1.06234391084669));
#9691=CARTESIAN_POINT('Ctrl Pts',(91.5075536873845,-1.96645606353663,0.995322334814222));
#9692=CARTESIAN_POINT('Ctrl Pts',(91.511618570171,-2.00039677936625,0.928265740071575));
#9693=CARTESIAN_POINT('Ctrl Pts',(91.5156834529574,-2.03087549983843,0.859526787188141));
#9694=CARTESIAN_POINT('Ctrl Pts',(91.5197483357439,-2.05774284607534,0.789500081966922));
#9695=CARTESIAN_POINT('Ctrl Pts',(91.5238204801591,-2.08465818894722,0.71934827893443));
#9696=CARTESIAN_POINT('Ctrl Pts',(91.5278926245744,-2.10794912307746,0.647904583136306));
#9697=CARTESIAN_POINT('Ctrl Pts',(91.5319647689896,-2.12751610903421,0.575579017859356));
#9698=CARTESIAN_POINT('Ctrl Pts',(91.5351021989511,-2.14259171582389,0.519854963814099));
#9699=CARTESIAN_POINT('Ctrl Pts',(91.5382396289125,-2.15545777028684,0.463607753674997));
#9700=CARTESIAN_POINT('Ctrl Pts',(91.5413770588739,-2.16608968285123,0.407027622951379));
#9701=CARTESIAN_POINT('Ctrl Pts',(91.5454500518947,-2.17989196886407,0.333575631866891));
#9702=CARTESIAN_POINT('Ctrl Pts',(91.5495230449155,-2.1899805161034,0.259279095173511));
#9703=CARTESIAN_POINT('Ctrl Pts',(91.5535960379363,-2.19626008992354,0.184547060147347));
#9704=CARTESIAN_POINT('Ctrl Pts',(91.5576630456856,-2.20253043589715,0.109924843999052));
#9705=CARTESIAN_POINT('Ctrl Pts',(91.5617300534348,-2.20500288170145,0.034868871960869));
#9706=CARTESIAN_POINT('Ctrl Pts',(91.5657970611841,-2.2036333135183,-0.0402022331763572));
#9707=CARTESIAN_POINT('Ctrl Pts',(91.5698593091387,-2.20226534819985,-0.115185479361682));
#9708=CARTESIAN_POINT('Ctrl Pts',(91.5739215570934,-2.19706431102125,-0.190183348458034));
#9709=CARTESIAN_POINT('Ctrl Pts',(91.5779838050481,-2.188038056443,-0.264774363481676));
#9710=CARTESIAN_POINT('Ctrl Pts',(91.5820434739773,-2.17901753242112,-0.339318022427398));
#9711=CARTESIAN_POINT('Ctrl Pts',(91.5861031429065,-2.16617666738495,-0.413454867052116));
#9712=CARTESIAN_POINT('Ctrl Pts',(91.5901628118357,-2.14957527116945,-0.486767042410209));
#9713=CARTESIAN_POINT('Ctrl Pts',(91.5942212153926,-2.13297904950067,-0.560056366842309));
#9714=CARTESIAN_POINT('Ctrl Pts',(91.5982796189495,-2.1126247292547,-0.63252106697144));
#9715=CARTESIAN_POINT('Ctrl Pts',(91.6023380225064,-2.08862320050254,-0.703753597733288));
#9716=CARTESIAN_POINT('Ctrl Pts',(91.6063964726597,-2.06462139617726,-0.774986946350117));
#9717=CARTESIAN_POINT('Ctrl Pts',(91.6104549228131,-2.0369724543631,-0.844987645597734));
#9718=CARTESIAN_POINT('Ctrl Pts',(91.6145133729665,-2.00583658980416,-0.913364973601909));
#9719=CARTESIAN_POINT('Ctrl Pts',(91.618575973101,-1.97466888716769,-0.981812221060761));
#9720=CARTESIAN_POINT('Ctrl Pts',(91.6226385732356,-1.94000733987067,-1.04863234686805));
#9721=CARTESIAN_POINT('Ctrl Pts',(91.6267011733701,-1.90205932544707,-1.11345692439351));
#9722=CARTESIAN_POINT('Ctrl Pts',(91.6307658951693,-1.8640914929368,-1.17831535610383));
#9723=CARTESIAN_POINT('Ctrl Pts',(91.6348306169685,-1.8228340376301,-1.24117576461928));
#9724=CARTESIAN_POINT('Ctrl Pts',(91.6388953387677,-1.77853766264782,-1.30169880638465));
#9725=CARTESIAN_POINT('Ctrl Pts',(91.6429673221698,-1.73416215243794,-1.36232997222761));
#9726=CARTESIAN_POINT('Ctrl Pts',(91.6470393055718,-1.6867371803264,-1.42061505978353));
#9727=CARTESIAN_POINT('Ctrl Pts',(91.6511112889739,-1.63655341271886,-1.47624826073336));
#9728=CARTESIAN_POINT('Ctrl Pts',(91.6542501176136,-1.59786999202185,-1.51913229713918));
#9729=CARTESIAN_POINT('Ctrl Pts',(91.6573889462533,-1.55754816328923,-1.56044129681809));
#9730=CARTESIAN_POINT('Ctrl Pts',(91.660527774893,-1.5157347010061,-1.60005134797791));
#9731=CARTESIAN_POINT('Ctrl Pts',(91.6646008602942,-1.46147566926288,-1.6514511342161));
#9732=CARTESIAN_POINT('Ctrl Pts',(91.6686739456953,-1.40449453518078,-1.7001869538125));
#9733=CARTESIAN_POINT('Ctrl Pts',(91.6727470310965,-1.34508352594941,-1.74595713241176));
#9734=CARTESIAN_POINT('Ctrl Pts',(91.6768141325442,-1.28575980011181,-1.79166006797689));
#9735=CARTESIAN_POINT('Ctrl Pts',(91.6808812339918,-1.22401366180412,-1.83440572391679));
#9736=CARTESIAN_POINT('Ctrl Pts',(91.6849483354395,-1.16017308285962,-1.87393020622648));
#9737=CARTESIAN_POINT('Ctrl Pts',(91.6890106786162,-1.09640719366077,-1.91340844720221));
#9738=CARTESIAN_POINT('Ctrl Pts',(91.6930730217929,-1.03055213607067,-1.94967275180106));
#9739=CARTESIAN_POINT('Ctrl Pts',(91.6971353649696,-0.962966436641571,-1.98250135987389));
#9740=CARTESIAN_POINT('Ctrl Pts',(91.7011951300076,-0.895423630021125,-2.01530913349186));
#9741=CARTESIAN_POINT('Ctrl Pts',(91.7052548950456,-0.826152789483229,-2.04468532935635));
#9742=CARTESIAN_POINT('Ctrl Pts',(91.7093146600835,-0.755537546089829,-2.07045381896061));
#9743=CARTESIAN_POINT('Ctrl Pts',(91.7133731604978,-0.684944299464992,-2.09621428163648));
#9744=CARTESIAN_POINT('Ctrl Pts',(91.7174316609121,-0.613007929694532,-2.11836910575678));
#9745=CARTESIAN_POINT('Ctrl Pts',(91.7214901613263,-0.5401310772917,-2.13679068215483));
#9746=CARTESIAN_POINT('Ctrl Pts',(91.7255487089482,-0.467253377200514,-2.15521247282882));
#9747=CARTESIAN_POINT('Ctrl Pts',(91.7296072565701,-0.393435636091098,-2.16990081428895));
#9748=CARTESIAN_POINT('Ctrl Pts',(91.733665804192,-0.3190930785952,-2.18077866992335));
#9749=CARTESIAN_POINT('Ctrl Pts',(91.7377285020664,-0.244674498734269,-2.19166764920401));
#9750=CARTESIAN_POINT('Ctrl Pts',(91.7417911999409,-0.169730504251898,-2.19873829212051));
#9751=CARTESIAN_POINT('Ctrl Pts',(91.7458538978153,-0.0946831335760688,
-2.20196528224589));
#9752=CARTESIAN_POINT('Ctrl Pts',(91.749918717659,-0.0195965652486128,-2.20519395784584));
#9753=CARTESIAN_POINT('Ctrl Pts',(91.7539835375028,0.0555930089127864,-2.20457498672492));
#9754=CARTESIAN_POINT('Ctrl Pts',(91.7580483573465,0.130464520518895,-2.20013522513635));
#9755=CARTESIAN_POINT('Ctrl Pts',(91.7621204381796,0.205469775137128,-2.19568753279982));
#9756=CARTESIAN_POINT('Ctrl Pts',(91.7661925190127,0.280155357103372,-2.18740547012963));
#9757=CARTESIAN_POINT('Ctrl Pts',(91.7702645998458,0.354106731721911,-2.1753676522715));
#9758=CARTESIAN_POINT('Ctrl Pts',(91.7734025635346,0.41109399150345,-2.1660912560311));
#9759=CARTESIAN_POINT('Ctrl Pts',(91.7765405272233,0.467645376738735,-2.15458564351988));
#9760=CARTESIAN_POINT('Ctrl Pts',(91.7796784909121,0.523577371692799,-2.14090698907058));
#9761=CARTESIAN_POINT('Ctrl Pts',(91.7837515628427,0.596177013136447,-2.1231521171182));
#9762=CARTESIAN_POINT('Ctrl Pts',(91.7878246347732,0.668012507929734,-2.10166596546539));
#9763=CARTESIAN_POINT('Ctrl Pts',(91.7918977067038,0.738671967899062,-2.07653069417241));
#9764=CARTESIAN_POINT('Ctrl Pts',(91.7959647946945,0.809227618761578,-2.0514323502783));
#9765=CARTESIAN_POINT('Ctrl Pts',(91.8000318826852,0.878610219013585,-2.02269568939249));
#9766=CARTESIAN_POINT('Ctrl Pts',(91.8040989706759,0.94642026728458,-1.99045338495354));
#9767=CARTESIAN_POINT('Ctrl Pts',(91.808161300483,1.01415098295711,-1.95824880155825));
#9768=CARTESIAN_POINT('Ctrl Pts',(91.8122236302901,1.0803123728134,-1.9225469270248));
#9769=CARTESIAN_POINT('Ctrl Pts',(91.8162859600972,1.14452379342688,-1.88352894490097));
#9770=CARTESIAN_POINT('Ctrl Pts',(91.820345711826,1.20869446351587,-1.84453572477774));
#9771=CARTESIAN_POINT('Ctrl Pts',(91.8244054635548,1.27091721306682,-1.80223082053647));
#9772=CARTESIAN_POINT('Ctrl Pts',(91.8284652152836,1.33083614956635,-1.75684124012599));
#9773=CARTESIAN_POINT('Ctrl Pts',(91.8325237024687,1.3907364223348,-1.71146579779893));
#9774=CARTESIAN_POINT('Ctrl Pts',(91.8365821896538,1.4483339264722,-1.66300787509311));
#9775=CARTESIAN_POINT('Ctrl Pts',(91.8406406768389,1.5033032499452,-1.6117367460923));
#9776=CARTESIAN_POINT('Ctrl Pts',(91.8446992113313,1.55827321416192,-1.56046501945536));
#9777=CARTESIAN_POINT('Ctrl Pts',(91.8487577458237,1.61061458895495,-1.50638034839004));
#9778=CARTESIAN_POINT('Ctrl Pts',(91.8528162803161,1.66003764990204,-1.44978998510395));
#9779=CARTESIAN_POINT('Ctrl Pts',(91.8568789653094,1.7095112538365,-1.3931417491171));
#9780=CARTESIAN_POINT('Ctrl Pts',(91.8609416503026,1.75606026939359,-1.33398306421869));
#9781=CARTESIAN_POINT('Ctrl Pts',(91.8650043352959,1.79943475082582,-1.27265493261938));
#9782=CARTESIAN_POINT('Ctrl Pts',(91.8690691423759,1.84283188831269,-1.21129476712698));
#9783=CARTESIAN_POINT('Ctrl Pts',(91.873133949456,1.88305093396025,-1.14776330210772));
#9784=CARTESIAN_POINT('Ctrl Pts',(91.877198756536,1.91988631850551,-1.08242899259738));
#9785=CARTESIAN_POINT('Ctrl Pts',(91.8812708249458,1.95678750540418,-1.01697797054615));
#9786=CARTESIAN_POINT('Ctrl Pts',(91.8853428933555,1.9902927444986,-0.94971809914239));
#9787=CARTESIAN_POINT('Ctrl Pts',(91.8894149617653,2.02024350971191,-0.881040385831942));
#9788=CARTESIAN_POINT('Ctrl Pts',(91.8925530434872,2.04332464180943,-0.828114880864567));
#9789=CARTESIAN_POINT('Ctrl Pts',(91.8956911252092,2.06429580802403,-0.77434782608217));
#9790=CARTESIAN_POINT('Ctrl Pts',(91.8988292069312,2.08310478479363,-0.719923923459901));
#9791=CARTESIAN_POINT('Ctrl Pts',(91.902902262903,2.10751779310294,-0.649284717339446));
#9792=CARTESIAN_POINT('Ctrl Pts',(91.9069753188747,2.12838068918864,-0.577266087120647));
#9793=CARTESIAN_POINT('Ctrl Pts',(91.9110483748465,2.14553935622089,-0.504258734091213));
#9794=CARTESIAN_POINT('Ctrl Pts',(91.9151154465387,2.16267281312546,-0.431358646077604));
#9795=CARTESIAN_POINT('Ctrl Pts',(91.9191825182309,2.1761127379984,-0.357473180329287));
#9796=CARTESIAN_POINT('Ctrl Pts',(91.923249589923,2.18575418144706,-0.283009996796427));
#9797=CARTESIAN_POINT('Ctrl Pts',(91.9273119029999,2.1953843440717,-0.208633937776962));
#9798=CARTESIAN_POINT('Ctrl Pts',(91.9313742160768,2.2012247941891,-0.133681975061804));
#9799=CARTESIAN_POINT('Ctrl Pts',(91.9354365291537,2.20322157239273,-0.0585722028209135));
#9800=CARTESIAN_POINT('Ctrl Pts',(91.9394962638958,2.20521708324879,0.016489897531451));
#9801=CARTESIAN_POINT('Ctrl Pts',(91.943555998638,2.20337375058481,0.0917091325659119));
#9802=CARTESIAN_POINT('Ctrl Pts',(91.9476157333801,2.19768954064834,0.166663382075649));
#9803=CARTESIAN_POINT('Ctrl Pts',(91.9516742033463,2.19200710157932,0.241594280223914));
#9804=CARTESIAN_POINT('Ctrl Pts',(91.9557326733125,2.18248619710266,0.316259880969424));
#9805=CARTESIAN_POINT('Ctrl Pts',(91.9597911432787,2.16917683287236,0.390240781735893));
#9806=CARTESIAN_POINT('Ctrl Pts',(91.9638496603438,2.1558673141854,0.464222541058963));
#9807=CARTESIAN_POINT('Ctrl Pts',(91.967908177409,2.13876933475411,0.537519115024085));
#9808=CARTESIAN_POINT('Ctrl Pts',(91.9719666944742,2.11798415696202,0.609720518645964));
#9809=CARTESIAN_POINT('Ctrl Pts',(91.9760293618367,2.09717772395114,0.681995756451299));
#9810=CARTESIAN_POINT('Ctrl Pts',(91.9800920291992,2.07267669532325,0.753173127615016));
#9811=CARTESIAN_POINT('Ctrl Pts',(91.9841546965617,2.04463225312056,0.822857794214245));
#9812=CARTESIAN_POINT('Ctrl Pts',(91.9882194858703,2.01657316320282,0.892578857370496));
#9813=CARTESIAN_POINT('Ctrl Pts',(91.9922842751789,1.98496717502972,0.96080522973781));
#9814=CARTESIAN_POINT('Ctrl Pts',(91.9963490644875,1.95001258876522,1.02716449688313));
#9815=CARTESIAN_POINT('Ctrl Pts',(92.0004211150953,1.91499555997531,1.09364230756357));
#9816=CARTESIAN_POINT('Ctrl Pts',(92.0044931657031,1.87661822892308,1.15824593975784));
#9817=CARTESIAN_POINT('Ctrl Pts',(92.0085652163109,1.83512334000208,1.22063029905849));
#9818=CARTESIAN_POINT('Ctrl Pts',(92.0117034518574,1.80314418552858,1.26870848687107));
#9819=CARTESIAN_POINT('Ctrl Pts',(92.0148416874039,1.76931430283252,1.31546910416486));
#9820=CARTESIAN_POINT('Ctrl Pts',(92.0179799229504,1.73376065666336,1.36076816005014));
#9821=CARTESIAN_POINT('Ctrl Pts',(92.02200424305,1.68816839605315,1.41885745844422));
#9822=CARTESIAN_POINT('Ctrl Pts',(92.0260285631496,1.63955510766071,1.47477792474616));
#9823=CARTESIAN_POINT('Ctrl Pts',(92.0300528832492,1.58815718622276,1.52819264225719));
#9824=CARTESIAN_POINT('Ctrl Pts',(92.0340704250322,1.53684583627448,1.58151739131159));
#9825=CARTESIAN_POINT('Ctrl Pts',(92.0380879668152,1.48275950468375,1.6323444236848));
#9826=CARTESIAN_POINT('Ctrl Pts',(92.0421055085981,1.42617564392087,1.68036871926577));
#9827=CARTESIAN_POINT('Ctrl Pts',(92.0461192504473,1.36964530218518,1.72834759176061));
#9828=CARTESIAN_POINT('Ctrl Pts',(92.0501329922964,1.31062248584389,1.77352866761993));
#9829=CARTESIAN_POINT('Ctrl Pts',(92.0541467341455,1.24942149077193,1.81564367054697));
#9830=CARTESIAN_POINT('Ctrl Pts',(92.0581580516425,1.18825746189424,1.85773323546636));
#9831=CARTESIAN_POINT('Ctrl Pts',(92.0621693691395,1.12491826638348,1.89676012336794));
#9832=CARTESIAN_POINT('Ctrl Pts',(92.0661806866365,1.05974987830951,1.93249739855529));
#9833=CARTESIAN_POINT('Ctrl Pts',(92.0701909521499,0.994598580899787,1.96822530150268));
#9834=CARTESIAN_POINT('Ctrl Pts',(92.0742012176632,0.927619472836517,2.00066506916662));
#9835=CARTESIAN_POINT('Ctrl Pts',(92.0782114831766,0.859184460530739,2.02963495801154));
#9836=CARTESIAN_POINT('Ctrl Pts',(92.0822246038918,0.790700724323783,2.05862547264366));
#9837=CARTESIAN_POINT('Ctrl Pts',(92.0862377246071,0.720759463365022,2.0841409770544));
#9838=CARTESIAN_POINT('Ctrl Pts',(92.0902508453224,0.649753047421367,2.10604771488365));
#9839=CARTESIAN_POINT('Ctrl Pts',(92.0942652306258,0.578724256405135,2.12796135581937));
#9840=CARTESIAN_POINT('Ctrl Pts',(92.0982796159292,0.506630116881663,2.14626384139877));
#9841=CARTESIAN_POINT('Ctrl Pts',(92.1022940012325,0.43387604195787,2.16087194905551));
#9842=CARTESIAN_POINT('Ctrl Pts',(92.1063150631176,0.361000965064446,2.1755043523933));
#9843=CARTESIAN_POINT('Ctrl Pts',(92.1103361250028,0.287464245593512,2.18643002725376));
#9844=CARTESIAN_POINT('Ctrl Pts',(92.1143571868879,0.213678759559795,2.19361742054374));
#9845=CARTESIAN_POINT('Ctrl Pts',(92.1182542601747,0.142168433484382,2.20058319207182));
#9846=CARTESIAN_POINT('Ctrl Pts',(92.1221513334614,0.0704248760134409,2.20403794717584));
#9847=CARTESIAN_POINT('Ctrl Pts',(92.1260484067482,-0.00117773768617677,
2.20399968532982));
#9848=CARTESIAN_POINT('',(92.8760484068423,0.00195929737048231,2.20399912911821));
#9849=CARTESIAN_POINT('Ctrl Pts',(92.1260484068025,-0.00117773868358856,
2.20399968532929));
#9850=CARTESIAN_POINT('Ctrl Pts',(92.1297424841915,-0.0690506209188907,
2.2039634164861));
#9851=CARTESIAN_POINT('Ctrl Pts',(92.1334365615805,-0.1368377559261,2.2007921759398));
#9852=CARTESIAN_POINT('Ctrl Pts',(92.1371306389695,-0.204330579702541,2.19450792074178));
#9853=CARTESIAN_POINT('Ctrl Pts',(92.141203704471,-0.27874772454576,2.18757894217584));
#9854=CARTESIAN_POINT('Ctrl Pts',(92.1452767699724,-0.352955528673427,2.17684701259296));
#9855=CARTESIAN_POINT('Ctrl Pts',(92.1493498354739,-0.426534513105433,2.16233307081262));
#9856=CARTESIAN_POINT('Ctrl Pts',(92.1534169168641,-0.500005395954242,2.1478404527852));
#9857=CARTESIAN_POINT('Ctrl Pts',(92.1574839982543,-0.572848828793578,2.12957694611157));
#9858=CARTESIAN_POINT('Ctrl Pts',(92.1615510796445,-0.644650186407671,2.10761527256863));
#9859=CARTESIAN_POINT('Ctrl Pts',(92.1656134026252,-0.716367537771774,2.08567929377437));
#9860=CARTESIAN_POINT('Ctrl Pts',(92.169675725606,-0.787044781913827,2.06005388339878));
#9861=CARTESIAN_POINT('Ctrl Pts',(92.1737380485868,-0.856278842209428,2.03086251242778));
#9862=CARTESIAN_POINT('Ctrl Pts',(92.1777977933541,-0.925468962083327,2.00168966819269));
#9863=CARTESIAN_POINT('Ctrl Pts',(92.1818575381215,-0.993217276852615,1.96895553944629));
#9864=CARTESIAN_POINT('Ctrl Pts',(92.1859172828888,-1.05913848129819,1.93283255286985));
#9865=CARTESIAN_POINT('Ctrl Pts',(92.1899757629871,-1.12503915033849,1.89672081912434));
#9866=CARTESIAN_POINT('Ctrl Pts',(92.1940342430855,-1.18911342067678,1.85722255284776));
#9867=CARTESIAN_POINT('Ctrl Pts',(92.1980927231838,-1.25099994751136,1.81455645581133));
#9868=CARTESIAN_POINT('Ctrl Pts',(92.2021512504738,-1.31288719395815,1.77188986265651));
#9869=CARTESIAN_POINT('Ctrl Pts',(92.2062097777639,-1.37258625431501,1.72605563808882));
#9870=CARTESIAN_POINT('Ctrl Pts',(92.2102683050539,-1.42976552330211,1.67731527995683));
#9871=CARTESIAN_POINT('Ctrl Pts',(92.2143309827146,-1.48700326550853,1.62852507848648));
#9872=CARTESIAN_POINT('Ctrl Pts',(92.2183936603752,-1.54171570642555,1.57682311916356));
#9873=CARTESIAN_POINT('Ctrl Pts',(92.2224563380358,-1.59360564660085,1.52251011265012));
#9874=CARTESIAN_POINT('Ctrl Pts',(92.2265211376994,-1.64552268973992,1.46816873756577));
#9875=CARTESIAN_POINT('Ctrl Pts',(92.230585937363,-1.69461398432032,1.41121396142467));
#9876=CARTESIAN_POINT('Ctrl Pts',(92.2346507370266,-1.74062220736324,1.35198015193786));
#9877=CARTESIAN_POINT('Ctrl Pts',(92.2387227979655,-1.78671261855897,1.29264052837992));
#9878=CARTESIAN_POINT('Ctrl Pts',(92.2427948589044,-1.82970868373798,1.23101413168966));
#9879=CARTESIAN_POINT('Ctrl Pts',(92.2468669198433,-1.86939631216582,1.16746452967995));
#9880=CARTESIAN_POINT('Ctrl Pts',(92.2500050648918,-1.89998169300921,1.1184898527615));
#9881=CARTESIAN_POINT('Ctrl Pts',(92.2531432099402,-1.92860305751758,1.06837358672696));
#9882=CARTESIAN_POINT('Ctrl Pts',(92.2562813549886,-1.95518168535522,1.01729080269682));
#9883=CARTESIAN_POINT('Ctrl Pts',(92.260354418832,-1.98967864020635,0.950989392965538));
#9884=CARTESIAN_POINT('Ctrl Pts',(92.2644274826753,-2.02086581555238,0.882803416388159));
#9885=CARTESIAN_POINT('Ctrl Pts',(92.2685005465187,-2.04853352782865,0.813096787204264));
#9886=CARTESIAN_POINT('Ctrl Pts',(92.2725676262122,-2.07616059067158,0.743492571076739));
#9887=CARTESIAN_POINT('Ctrl Pts',(92.2766347059057,-2.10027828190842,0.672372578128671));
#9888=CARTESIAN_POINT('Ctrl Pts',(92.2807017855992,-2.12072307109084,0.600124700160767));
#9889=CARTESIAN_POINT('Ctrl Pts',(92.2847641068334,-2.14114393999043,0.527961351784204));
#9890=CARTESIAN_POINT('Ctrl Pts',(92.2888264280676,-2.1579003151836,0.4546731972809));
#9891=CARTESIAN_POINT('Ctrl Pts',(92.2928887493018,-2.17087757788415,0.380665918936582));
#9892=CARTESIAN_POINT('Ctrl Pts',(92.2969484922929,-2.18384660427429,0.306705610968948));
#9893=CARTESIAN_POINT('Ctrl Pts',(92.301008235284,-2.1930411954764,0.232027553946412));
#9894=CARTESIAN_POINT('Ctrl Pts',(92.3050679782751,-2.19839750858312,0.157049018639201));
#9895=CARTESIAN_POINT('Ctrl Pts',(92.3091264565699,-2.20375215308451,0.0820938407387217));
#9896=CARTESIAN_POINT('Ctrl Pts',(92.3131849348648,-2.20527085951197,0.00683884633960688));
#9897=CARTESIAN_POINT('Ctrl Pts',(92.3172434131597,-2.20294166114478,-0.0682937595442691));
#9898=CARTESIAN_POINT('Ctrl Pts',(92.3213019386216,-2.20061243570799,-0.143427238608045));
#9899=CARTESIAN_POINT('Ctrl Pts',(92.3253604640835,-2.19443523327064,-0.218437849156203));
#9900=CARTESIAN_POINT('Ctrl Pts',(92.3294189895454,-2.18445017045167,-0.292905194241523));
#9901=CARTESIAN_POINT('Ctrl Pts',(92.3334816653521,-2.17445489666966,-0.367448691407455));
#9902=CARTESIAN_POINT('Ctrl Pts',(92.3375443411588,-2.16064404998701,-0.441447339419365));
#9903=CARTESIAN_POINT('Ctrl Pts',(92.3416070169655,-2.14310934695328,-0.514488412893325));
#9904=CARTESIAN_POINT('Ctrl Pts',(92.3456718147579,-2.1255654853278,-0.587567636621174));
#9905=CARTESIAN_POINT('Ctrl Pts',(92.3497366125503,-2.10429402923873,-0.659687831422038));
#9906=CARTESIAN_POINT('Ctrl Pts',(92.3538014103427,-2.0794365896898,-0.730451551753623));
#9907=CARTESIAN_POINT('Ctrl Pts',(92.3578734694033,-2.05453474534072,-0.801341682886763));
#9908=CARTESIAN_POINT('Ctrl Pts',(92.3619455284638,-2.02603430355675,-0.870870057001498));
#9909=CARTESIAN_POINT('Ctrl Pts',(92.3660175875243,-1.99412484198433,-0.938659743773515));
#9910=CARTESIAN_POINT('Ctrl Pts',(92.3691557486855,-1.96953358937916,-0.990902346101763));
#9911=CARTESIAN_POINT('Ctrl Pts',(92.3722939098467,-1.94291867194688,-1.04211273039333));
#9912=CARTESIAN_POINT('Ctrl Pts',(92.3754320710079,-1.91438458534593,-1.09212987295006));
#9913=CARTESIAN_POINT('Ctrl Pts',(92.3795051363958,-1.87734977593337,-1.1570478557071));
#9914=CARTESIAN_POINT('Ctrl Pts',(92.3835782017837,-1.83693769024174,-1.220205082403));
#9915=CARTESIAN_POINT('Ctrl Pts',(92.3876512671716,-1.79334058564205,-1.28122813889214));
#9916=CARTESIAN_POINT('Ctrl Pts',(92.3917183484339,-1.74980753367201,-1.34216154063763));
#9917=CARTESIAN_POINT('Ctrl Pts',(92.3957854296962,-1.70309902859019,-1.40096661217287));
#9918=CARTESIAN_POINT('Ctrl Pts',(92.3998525109586,-1.65345248745313,-1.45729573928392));
#9919=CARTESIAN_POINT('Ctrl Pts',(92.4039148337905,-1.60386403210157,-1.51355896207375));
#9920=CARTESIAN_POINT('Ctrl Pts',(92.4079771566225,-1.55134468426143,-1.56735163936944));
#9921=CARTESIAN_POINT('Ctrl Pts',(92.4120394794544,-1.49617331510964,-1.61835762770589));
#9922=CARTESIAN_POINT('Ctrl Pts',(92.4160992240601,-1.44103696145939,-1.66933124417464));
#9923=CARTESIAN_POINT('Ctrl Pts',(92.4201589686658,-1.38325227623498,-1.71752135802385));
#9924=CARTESIAN_POINT('Ctrl Pts',(92.4242187132716,-1.32313538205734,-1.76264822376672));
#9925=CARTESIAN_POINT('Ctrl Pts',(92.4282771931957,-1.26303721534587,-1.80776103170001));
#9926=CARTESIAN_POINT('Ctrl Pts',(92.4323356731198,-1.20060866376322,-1.84981219971173));
#9927=CARTESIAN_POINT('Ctrl Pts',(92.4363941530439,-1.1361981046941,-1.88856291049293));
#9928=CARTESIAN_POINT('Ctrl Pts',(92.4404526801473,-1.07178679686028,-1.92731407174631));
#9929=CARTESIAN_POINT('Ctrl Pts',(92.4445112072507,-1.00539384584266,-1.96276445498689));
#9930=CARTESIAN_POINT('Ctrl Pts',(92.4485697343542,-0.937394329159364,-1.99471999831051));
#9931=CARTESIAN_POINT('Ctrl Pts',(92.4526324118101,-0.869325274449837,-2.02670822018124));
#9932=CARTESIAN_POINT('Ctrl Pts',(92.456695089266,-0.799646806351258,-2.05519426171501));
#9933=CARTESIAN_POINT('Ctrl Pts',(92.460757766722,-0.728755512362739,-2.08003158706807));
#9934=CARTESIAN_POINT('Ctrl Pts',(92.4648225661705,-0.657827190871765,-2.10488188529938));
#9935=CARTESIAN_POINT('Ctrl Pts',(92.468887365619,-0.58568524050643,-2.12607953745661));
#9936=CARTESIAN_POINT('Ctrl Pts',(92.4729521650675,-0.512740439975553,-2.14352822263055));
#9937=CARTESIAN_POINT('Ctrl Pts',(92.4770242257767,-0.439665332595621,-2.16100807771884));
#9938=CARTESIAN_POINT('Ctrl Pts',(92.4810962864858,-0.365784980496466,-2.1747255016663));
#9939=CARTESIAN_POINT('Ctrl Pts',(92.4851683471949,-0.291518908767242,-2.18463560481632));
#9940=CARTESIAN_POINT('Ctrl Pts',(92.4883064938056,-0.234285523036974,-2.19227285750796));
#9941=CARTESIAN_POINT('Ctrl Pts',(92.4914446404162,-0.176823250123836,-2.19764997578432));
#9942=CARTESIAN_POINT('Ctrl Pts',(92.4945827870269,-0.119324044631328,-2.20076754164833));
#9943=CARTESIAN_POINT('Ctrl Pts',(92.4986558519924,-0.0446946443849952,
-2.20481389443992));
#9944=CARTESIAN_POINT('Ctrl Pts',(92.502728916958,0.0302847283983598,-2.20506765315536));
#9945=CARTESIAN_POINT('Ctrl Pts',(92.5068019819235,0.10519605238616,-2.2014880854918));
#9946=CARTESIAN_POINT('Ctrl Pts',(92.51086906276,0.179997316987484,-2.19791377691325));
#9947=CARTESIAN_POINT('Ctrl Pts',(92.5149361435965,0.254730258330918,-2.19051734618733));
#9948=CARTESIAN_POINT('Ctrl Pts',(92.5190032244329,0.328974071322962,-2.1793099963973));
#9949=CARTESIAN_POINT('Ctrl Pts',(92.5230655468359,0.403131019985645,-2.16811575906586));
#9950=CARTESIAN_POINT('Ctrl Pts',(92.5271278692388,0.476799507535252,-2.15311953205287));
#9951=CARTESIAN_POINT('Ctrl Pts',(92.5311901916418,0.549562719159225,-2.13438441188796));
#9952=CARTESIAN_POINT('Ctrl Pts',(92.5352499358168,0.622279750266912,-2.11566118231313));
#9953=CARTESIAN_POINT('Ctrl Pts',(92.5393096799918,0.694092184373747,-2.09320388721637));
#9954=CARTESIAN_POINT('Ctrl Pts',(92.5433694241668,0.764593615353688,-2.06712665392336));
#9955=CARTESIAN_POINT('Ctrl Pts',(92.5474279036591,0.835073083881017,-2.04105754415341));
#9956=CARTESIAN_POINT('Ctrl Pts',(92.5514863831514,0.904241912626709,-2.01137090066691));
#9957=CARTESIAN_POINT('Ctrl Pts',(92.5555448626437,0.971710619063381,-1.97823013646023));
#9958=CARTESIAN_POINT('Ctrl Pts',(92.5596033893149,1.0391801098077,-1.94508898700006));
#9959=CARTESIAN_POINT('Ctrl Pts',(92.563661915986,1.10494901124095,-1.90849384920838));
#9960=CARTESIAN_POINT('Ctrl Pts',(92.5677204426572,1.16865099081085,-1.86865482678766));
#9961=CARTESIAN_POINT('Ctrl Pts',(92.5717831196832,1.23241811367999,-1.82877506394762));
#9962=CARTESIAN_POINT('Ctrl Pts',(92.5758457967091,1.29411368805856,-1.78564504579));
#9963=CARTESIAN_POINT('Ctrl Pts',(92.5799084737351,1.35339967222153,-1.73951870562827));
#9964=CARTESIAN_POINT('Ctrl Pts',(92.5839732727543,1.41271662228537,-1.69336827303227));
#9965=CARTESIAN_POINT('Ctrl Pts',(92.5880380717735,1.46962111415404,-1.64421871423083));
#9966=CARTESIAN_POINT('Ctrl Pts',(92.5921028707926,1.52380962237535,-1.59236309764962));
#9967=CARTESIAN_POINT('Ctrl Pts',(92.5961749310783,1.57809493174209,-1.54041484734869));
#9968=CARTESIAN_POINT('Ctrl Pts',(92.600246991364,1.62965423832684,-1.48575123149518));
#9969=CARTESIAN_POINT('Ctrl Pts',(92.6043190516497,1.67822250537906,-1.42870053630537));
#9970=CARTESIAN_POINT('Ctrl Pts',(92.6074572021151,1.7156518456056,-1.38473417699251));
#9971=CARTESIAN_POINT('Ctrl Pts',(92.6105953525806,1.75130556742079,-1.33935084853213));
#9972=CARTESIAN_POINT('Ctrl Pts',(92.613733503046,1.78508015467132,-1.29271220362408));
#9973=CARTESIAN_POINT('Ctrl Pts',(92.617806567852,1.82891682986636,-1.23217902484069));
#9974=CARTESIAN_POINT('Ctrl Pts',(92.621879632658,1.86975547438596,-1.16929679093106));
#9975=CARTESIAN_POINT('Ctrl Pts',(92.625952697464,1.90733536041205,-1.10439477675414));
#9976=CARTESIAN_POINT('Ctrl Pts',(92.6300197781367,1.94486003419431,-1.03958811640106));
#9977=CARTESIAN_POINT('Ctrl Pts',(92.6340868588094,1.9791352178715,-0.972767977151691));
#9978=CARTESIAN_POINT('Ctrl Pts',(92.6381539394821,2.00994232671424,-0.904294113263235));
#9979=CARTESIAN_POINT('Ctrl Pts',(92.6422162617157,2.04071339158268,-0.835900363033059));
#9980=CARTESIAN_POINT('Ctrl Pts',(92.6462785839493,2.06802424824332,-0.765857165481326));
#9981=CARTESIAN_POINT('Ctrl Pts',(92.6503409061829,2.09170209012148,-0.694549037996206));
#9982=CARTESIAN_POINT('Ctrl Pts',(92.6544006501853,2.11536490439987,-0.62328616759172));
#9983=CARTESIAN_POINT('Ctrl Pts',(92.6584603941876,2.13539912935187,-0.550760412332747));
#9984=CARTESIAN_POINT('Ctrl Pts',(92.6625201381899,2.15168048912937,-0.477375190704345));
#9985=CARTESIAN_POINT('Ctrl Pts',(92.6665786175064,2.16795677696044,-0.404012829937562));
#9986=CARTESIAN_POINT('Ctrl Pts',(92.670637096823,2.18048241744174,-0.32979200020964));
#9987=CARTESIAN_POINT('Ctrl Pts',(92.6746955761395,2.189183728598,-0.255128599811503));
#9988=CARTESIAN_POINT('Ctrl Pts',(92.6787541026321,2.19788514089883,-0.180464331521415));
#9989=CARTESIAN_POINT('Ctrl Pts',(92.6828126291247,2.20276208212055,-0.10535795680518));
#9990=CARTESIAN_POINT('Ctrl Pts',(92.6868711556172,2.20379265668724,-0.0302312145207114));
#9991=CARTESIAN_POINT('Ctrl Pts',(92.6909338324614,2.20482428514549,0.0449723542663247));
#9992=CARTESIAN_POINT('Ctrl Pts',(92.6949965093056,2.20200168562654,0.120195853738261));
#9993=CARTESIAN_POINT('Ctrl Pts',(92.6990591861497,2.1953551296397,0.195017575527558));
#9994=CARTESIAN_POINT('Ctrl Pts',(92.703123984985,2.18870510206669,0.269878377715137));
#9995=CARTESIAN_POINT('Ctrl Pts',(92.7071887838203,2.17822720718454,0.344336511074202));
#9996=CARTESIAN_POINT('Ctrl Pts',(92.7112535826556,2.16400331096335,0.417978073754652));
#9997=CARTESIAN_POINT('Ctrl Pts',(92.7153256427561,2.1497540054939,0.491751188066224));
#9998=CARTESIAN_POINT('Ctrl Pts',(92.7193977028566,2.13174544698614,0.564704353817959));
#9999=CARTESIAN_POINT('Ctrl Pts',(92.7234697629571,2.11010995572858,0.63643693696638));
#10000=CARTESIAN_POINT('Ctrl Pts',(92.7266079149931,2.09343646386817,0.691717985453458));
#10001=CARTESIAN_POINT('Ctrl Pts',(92.7297460670292,2.07460994892254,0.746274379256409));
#10002=CARTESIAN_POINT('Ctrl Pts',(92.7328842190652,2.05371019199788,0.799931526622132));
#10003=CARTESIAN_POINT('Ctrl Pts',(92.7369572840645,2.02658401473007,0.869574120857797));
#10004=CARTESIAN_POINT('Ctrl Pts',(92.7410303490637,1.99585907533792,0.937969653685009));
#10005=CARTESIAN_POINT('Ctrl Pts',(92.745103414063,1.96167085979995,1.00472057698234));
#10006=CARTESIAN_POINT('Ctrl Pts',(92.7491704949322,1.92753287344565,1.07137343010157));
#10007=CARTESIAN_POINT('Ctrl Pts',(92.7532375758013,1.88994192900946,1.13638604950373));
#10008=CARTESIAN_POINT('Ctrl Pts',(92.7573046566705,1.84908196421617,1.1993797937311));
#10009=CARTESIAN_POINT('Ctrl Pts',(92.7613669791044,1.80826980508606,1.26229983604184));
#10010=CARTESIAN_POINT('Ctrl Pts',(92.7654293015382,1.76419648295336,1.3232052974903));
#10011=CARTESIAN_POINT('Ctrl Pts',(92.7694916239721,1.71709155235281,1.38174259572419));
#10012=CARTESIAN_POINT('Ctrl Pts',(92.773551368177,1.67001651777894,1.4402427421651));
#10013=CARTESIAN_POINT('Ctrl Pts',(92.7776111123818,1.61991399141386,1.49637733689366));
#10014=CARTESIAN_POINT('Ctrl Pts',(92.7816708565866,1.56705570899619,1.54982334635353));
#10015=CARTESIAN_POINT('Ctrl Pts',(92.7857293361077,1.51421389289049,1.60325270641382));
#10016=CARTESIAN_POINT('Ctrl Pts',(92.7897878156287,1.45861836070841,1.6539948048556));
#10017=CARTESIAN_POINT('Ctrl Pts',(92.7938462951497,1.40057875018951,1.70176237016735));
#10018=CARTESIAN_POINT('Ctrl Pts',(92.7979048218484,1.34253846499085,1.74953049075177));
#10019=CARTESIAN_POINT('Ctrl Pts',(92.8019633485471,1.28205441484255,1.79432370752333));
#10020=CARTESIAN_POINT('Ctrl Pts',(92.8060218752458,1.21946920537885,1.8358951106021));
#10021=CARTESIAN_POINT('Ctrl Pts',(92.8100845522973,1.1568199946859,1.87750902565647));
#10022=CARTESIAN_POINT('Ctrl Pts',(92.8141472293487,1.09206573244855,1.91589428290774));
#10023=CARTESIAN_POINT('Ctrl Pts',(92.8182099064002,1.02557726386979,1.9508478351305));
#10024=CARTESIAN_POINT('Ctrl Pts',(92.8222747054438,0.959054067449693,1.98581964407419));
#10025=CARTESIAN_POINT('Ctrl Pts',(92.8263395044873,0.890795294716255,2.01735597810705));
#10026=CARTESIAN_POINT('Ctrl Pts',(92.8304043035309,0.821193184476299,2.04530138458118));
#10027=CARTESIAN_POINT('Ctrl Pts',(92.8344763638389,0.751466738611704,2.07329671209301));
#10028=CARTESIAN_POINT('Ctrl Pts',(92.8385484241469,0.680392614288185,2.09768814386498));
#10029=CARTESIAN_POINT('Ctrl Pts',(92.8426204844549,0.608379235982138,2.11836982258193));
#10030=CARTESIAN_POINT('Ctrl Pts',(92.8457586346647,0.552881826526517,2.13430824428888));
#10031=CARTESIAN_POINT('Ctrl Pts',(92.8488967848745,0.496826933752397,2.14804443234602));
#10032=CARTESIAN_POINT('Ctrl Pts',(92.8520349350843,0.440404527712738,2.15955084496062));
#10033=CARTESIAN_POINT('Ctrl Pts',(92.8578492539753,0.335865917584354,2.1808697582563));
#10034=CARTESIAN_POINT('Ctrl Pts',(92.8636635728662,0.229731969372485,2.19460365402509));
#10035=CARTESIAN_POINT('Ctrl Pts',(92.8694778917572,0.122912597202681,2.20057003829664));
#10036=CARTESIAN_POINT('Ctrl Pts',(92.8716680634389,0.082675250682759,2.20281749085632));
#10037=CARTESIAN_POINT('Ctrl Pts',(92.8738582351207,0.0423408978578493,
2.20396323092196));
#10038=CARTESIAN_POINT('Ctrl Pts',(92.8760484068025,0.00195929810404175,
2.20399912911756));
#10039=CARTESIAN_POINT('',(93.6260484067633,4.74792226950262E-5,2.20399999948859));
#10040=CARTESIAN_POINT('Ctrl Pts',(92.8760484068423,0.00195929737048818,
2.20399912911821));
#10041=CARTESIAN_POINT('Ctrl Pts',(92.8800549703073,-0.0719122824601498,
2.20406479901354));
#10042=CARTESIAN_POINT('Ctrl Pts',(92.8840615337723,-0.145903667991656,
2.20041230851384));
#10043=CARTESIAN_POINT('Ctrl Pts',(92.8880680972373,-0.219604015837993,
2.19303216488674));
#10044=CARTESIAN_POINT('Ctrl Pts',(92.892071309022,-0.293242709849697,2.18565819509963));
#10045=CARTESIAN_POINT('Ctrl Pts',(92.8960745208068,-0.3665903610426,2.17456280216026));
#10046=CARTESIAN_POINT('Ctrl Pts',(92.9000777325915,-0.439237413510549,
2.15978853005857));
#10047=CARTESIAN_POINT('Ctrl Pts',(92.9040789764028,-0.511848752786769,
2.14502152096886));
#10048=CARTESIAN_POINT('Ctrl Pts',(92.9080802202141,-0.583759694539525,
2.1265793172489));
#10049=CARTESIAN_POINT('Ctrl Pts',(92.9120814640254,-0.654568895058323,
2.10455590603389));
#10050=CARTESIAN_POINT('Ctrl Pts',(92.9160821208197,-0.725367707256604,
2.08253572584328));
#10051=CARTESIAN_POINT('Ctrl Pts',(92.920082777614,-0.795064629188487,2.05693552828468));
#10052=CARTESIAN_POINT('Ctrl Pts',(92.9240834344083,-0.863273309956541,
2.0278992066463));
#10053=CARTESIAN_POINT('Ctrl Pts',(92.9280876445556,-0.931542573156908,
1.99883709516752));
#10054=CARTESIAN_POINT('Ctrl Pts',(92.9320918547029,-0.998320500086283,
1.96633295551533));
#10055=CARTESIAN_POINT('Ctrl Pts',(92.9360960648502,-1.06324149190924,1.93057854797017));
#10056=CARTESIAN_POINT('Ctrl Pts',(92.9401019558659,-1.12818973595942,1.89480913160874));
#10057=CARTESIAN_POINT('Ctrl Pts',(92.9441078468817,-1.19127907374594,1.85578699064998));
#10058=CARTESIAN_POINT('Ctrl Pts',(92.9481137378974,-1.25217171549734,1.81374805166221));
#10059=CARTESIAN_POINT('Ctrl Pts',(92.9521268553409,-1.31317420454101,1.77163327652273));
#10060=CARTESIAN_POINT('Ctrl Pts',(92.9561399727845,-1.37197169089296,1.72649113356451));
#10061=CARTESIAN_POINT('Ctrl Pts',(92.960153090228,-1.42825884302409,1.67859842646283));
#10062=CARTESIAN_POINT('Ctrl Pts',(92.9638306105198,-1.47983897917582,1.63471074944508));
#10063=CARTESIAN_POINT('Ctrl Pts',(92.9675081308117,-1.52931129181564,1.58851397528272));
#10064=CARTESIAN_POINT('Ctrl Pts',(92.9711856511035,-1.5764697644302,1.54024643542435));
#10065=CARTESIAN_POINT('Ctrl Pts',(92.9752587160244,-1.62870048113314,1.48678736305582));
#10066=CARTESIAN_POINT('Ctrl Pts',(92.9793317809454,-1.67830959326401,1.43056542275226));
#10067=CARTESIAN_POINT('Ctrl Pts',(92.9834048458663,-1.72499095324703,1.3718681464397));
#10068=CARTESIAN_POINT('Ctrl Pts',(92.987471926656,-1.77160372915663,1.31325710793833));
#10069=CARTESIAN_POINT('Ctrl Pts',(92.9915390074458,-1.81529699831034,1.25217832445775));
#10070=CARTESIAN_POINT('Ctrl Pts',(92.9956060882355,-1.85580183704518,1.1889556516623));
#10071=CARTESIAN_POINT('Ctrl Pts',(92.9996684105887,-1.89625928559648,1.12580694864828));
#10072=CARTESIAN_POINT('Ctrl Pts',(93.0037307329418,-1.93353545896034,1.06051973979805));
#10073=CARTESIAN_POINT('Ctrl Pts',(93.007793055295,-1.96740309055949,0.99344908236757));
#10074=CARTESIAN_POINT('Ctrl Pts',(93.0118527994184,-2.0012492274252,0.926420992599341));
#10075=CARTESIAN_POINT('Ctrl Pts',(93.0159125435418,-2.0316909006833,0.857612125508566));
#10076=CARTESIAN_POINT('Ctrl Pts',(93.0199722876652,-2.05854608239204,0.78740334433402));
#10077=CARTESIAN_POINT('Ctrl Pts',(93.0240307671041,-2.0853928982212,0.717216434477091));
#10078=CARTESIAN_POINT('Ctrl Pts',(93.0280892465431,-2.10865527030138,0.645630922051442));
#10079=CARTESIAN_POINT('Ctrl Pts',(93.0321477259821,-2.12819939080647,0.57304742645872));
#10080=CARTESIAN_POINT('Ctrl Pts',(93.0362062525982,-2.14774373849916,0.500463087130436));
#10081=CARTESIAN_POINT('Ctrl Pts',(93.0402647792143,-2.16356962638733,0.426881203107006));
#10082=CARTESIAN_POINT('Ctrl Pts',(93.0443233058304,-2.17559361893673,0.352715757008075));
#10083=CARTESIAN_POINT('Ctrl Pts',(93.0483859827991,-2.1876299075268,0.278474467437261));
#10084=CARTESIAN_POINT('Ctrl Pts',(93.0524486597678,-2.19585646025411,0.203648896438431));
#10085=CARTESIAN_POINT('Ctrl Pts',(93.0565113367365,-2.20024145044579,0.12866063788201));
#10086=CARTESIAN_POINT('Ctrl Pts',(93.060576135697,-2.20462873097793,0.0536332119307196));
#10087=CARTESIAN_POINT('Ctrl Pts',(93.0646409346575,-2.20517044978059,-0.0215565929029333));
#10088=CARTESIAN_POINT('Ctrl Pts',(93.0687057336181,-2.20188696162339,-0.0964873475276276));
#10089=CARTESIAN_POINT('Ctrl Pts',(93.0727777938436,-2.19859760791717,-0.171551956758485));
#10090=CARTESIAN_POINT('Ctrl Pts',(93.0768498540691,-2.19146944369823,-0.246356115437402));
#10091=CARTESIAN_POINT('Ctrl Pts',(93.0809219142946,-2.18057467730157,-0.320484128641563));
#10092=CARTESIAN_POINT('Ctrl Pts',(93.0840600652373,-2.17217857814179,-0.377611204773327));
#10093=CARTESIAN_POINT('Ctrl Pts',(93.0871982161799,-2.16154653352215,-0.434336816769531));
#10094=CARTESIAN_POINT('Ctrl Pts',(93.0903363671226,-2.14873188981487,-0.49047656997314));
#10095=CARTESIAN_POINT('Ctrl Pts',(93.0944094320672,-2.13209952348991,-0.56334140820073));
#10096=CARTESIAN_POINT('Ctrl Pts',(93.0984824970118,-2.11172454344625,-0.635499781504664));
#10097=CARTESIAN_POINT('Ctrl Pts',(93.1025555619564,-2.08768274156705,-0.706538583916761));
#10098=CARTESIAN_POINT('Ctrl Pts',(93.1066226427702,-2.06367626180753,-0.777473016402938));
#10099=CARTESIAN_POINT('Ctrl Pts',(93.1106897235839,-2.03601380795103,-0.847290695225555));
#10100=CARTESIAN_POINT('Ctrl Pts',(93.1147568043977,-2.00482187045235,-0.915590119953207));
#10101=CARTESIAN_POINT('Ctrl Pts',(93.1188191267755,-1.9736664271486,-0.983809635168375));
#10102=CARTESIAN_POINT('Ctrl Pts',(93.1228814491532,-1.93898990183575,-1.05051399333959));
#10103=CARTESIAN_POINT('Ctrl Pts',(93.1269437715309,-1.9009675803897,-1.11531980091243));
#10104=CARTESIAN_POINT('Ctrl Pts',(93.1310035156792,-1.86296939052679,-1.1800844782577));
#10105=CARTESIAN_POINT('Ctrl Pts',(93.1350632598274,-1.82162985933606,-1.24295258532953));
#10106=CARTESIAN_POINT('Ctrl Pts',(93.1391230039756,-1.77717047369368,-1.30356476917389));
#10107=CARTESIAN_POINT('Ctrl Pts',(93.1431814834397,-1.73272493795903,-1.36415807121993));
#10108=CARTESIAN_POINT('Ctrl Pts',(93.1472399629038,-1.68516175963341,-1.42249646059683));
#10109=CARTESIAN_POINT('Ctrl Pts',(93.1512984423678,-1.63474515718172,-1.47825040878428));
#10110=CARTESIAN_POINT('Ctrl Pts',(93.1553569690093,-1.58432796866732,-1.5340050050779));
#10111=CARTESIAN_POINT('Ctrl Pts',(93.1594154956507,-1.53105761173668,-1.58717474759307));
#10112=CARTESIAN_POINT('Ctrl Pts',(93.1634740222921,-1.47523682930359,-1.63746520496355));
#10113=CARTESIAN_POINT('Ctrl Pts',(93.1675366992863,-1.41935896311644,-1.68780709063678));
#10114=CARTESIAN_POINT('Ctrl Pts',(93.1715993762805,-1.36092581865817,-1.73526349100998));
#10115=CARTESIAN_POINT('Ctrl Pts',(93.1756620532747,-1.30027449879505,-1.77957922773427));
#10116=CARTESIAN_POINT('Ctrl Pts',(93.1797268522608,-1.23959149991492,-1.82391811117623));
#10117=CARTESIAN_POINT('Ctrl Pts',(93.183791651247,-1.17668841822423,-1.86511280242322));
#10118=CARTESIAN_POINT('Ctrl Pts',(93.1878564502331,-1.11193049106998,-1.90295207060737));
#10119=CARTESIAN_POINT('Ctrl Pts',(93.1919285104841,-1.04705688182033,-1.94085893400379));
#10120=CARTESIAN_POINT('Ctrl Pts',(93.1960005707352,-0.980322233403132,
-1.97539818189542));
#10121=CARTESIAN_POINT('Ctrl Pts',(93.2000726309862,-0.912115058956017,
-2.0064052729261));
#10122=CARTESIAN_POINT('Ctrl Pts',(93.2032107817047,-0.859550907076969,
-2.03030102077779));
#10123=CARTESIAN_POINT('Ctrl Pts',(93.2063489324232,-0.806112702462154,
-2.05209994820842));
#10124=CARTESIAN_POINT('Ctrl Pts',(93.2094870831417,-0.751984331871373,
-2.07174698373618));
#10125=CARTESIAN_POINT('Ctrl Pts',(93.2135601480768,-0.681730099992325,
-2.09724724126542));
#10126=CARTESIAN_POINT('Ctrl Pts',(93.2176332130119,-0.610041822848098,
-2.11921907646067));
#10127=CARTESIAN_POINT('Ctrl Pts',(93.221706277947,-0.537307779208416,-2.13750236266586));
#10128=CARTESIAN_POINT('Ctrl Pts',(93.2257733587512,-0.464680596138525,
-2.15575878713913));
#10129=CARTESIAN_POINT('Ctrl Pts',(93.2298404395554,-0.391011156236629,
-2.17033730651605));
#10130=CARTESIAN_POINT('Ctrl Pts',(93.2339075203595,-0.316705453413108,
-2.1811266941144));
#10131=CARTESIAN_POINT('Ctrl Pts',(93.2379698427276,-0.242486687378207,
-2.19190345825757));
#10132=CARTESIAN_POINT('Ctrl Pts',(93.2420321650956,-0.167633607545572,
-2.19889983019213));
#10133=CARTESIAN_POINT('Ctrl Pts',(93.2460944874636,-0.0925634274613625,
-2.20205540618228));
#10134=CARTESIAN_POINT('Ctrl Pts',(93.250154231602,-0.0175408920837323,
-2.20520897942658));
#10135=CARTESIAN_POINT('Ctrl Pts',(93.2542139757405,0.0576979942920653,
-2.20452657394543));
#10136=CARTESIAN_POINT('Ctrl Pts',(93.2582737198789,0.132731191454727,-2.19999964336702));
#10137=CARTESIAN_POINT('Ctrl Pts',(93.2623321993331,0.207741014410062,-2.19547412300992));
#10138=CARTESIAN_POINT('Ctrl Pts',(93.2663906787874,0.282544799089149,-2.18710648415298));
#10139=CARTESIAN_POINT('Ctrl Pts',(93.2704491582416,0.356722419692342,-2.17494025556769));
#10140=CARTESIAN_POINT('Ctrl Pts',(93.2745076848732,0.43090090256517,-2.1627738855574));
#10141=CARTESIAN_POINT('Ctrl Pts',(93.2785662115047,0.504452736034628,-2.14680891719227));
#10142=CARTESIAN_POINT('Ctrl Pts',(93.2826247381363,0.576966419918423,-2.12714027517851));
#10143=CARTESIAN_POINT('Ctrl Pts',(93.2866874151206,0.649554258142763,-2.10745151951034));
#10144=CARTESIAN_POINT('Ctrl Pts',(93.2907500921049,0.721101364916498,-2.08405165209815));
#10145=CARTESIAN_POINT('Ctrl Pts',(93.2948127690892,0.791210615063416,-2.05708574507991));
#10146=CARTESIAN_POINT('Ctrl Pts',(93.2988775680654,0.861356484234057,-2.03010575339828));
#10147=CARTESIAN_POINT('Ctrl Pts',(93.3029423670417,0.930062564526948,-1.99955620710848));
#10148=CARTESIAN_POINT('Ctrl Pts',(93.307007166018,0.996953424529923,-1.96562963686399));
#10149=CARTESIAN_POINT('Ctrl Pts',(93.3110792262592,1.06396377685304,-1.93164246096138));
#10150=CARTESIAN_POINT('Ctrl Pts',(93.3151512865005,1.1291520170853,-1.89426644921628));
#10151=CARTESIAN_POINT('Ctrl Pts',(93.3192233467418,1.19216934477753,-1.85373899278532));
#10152=CARTESIAN_POINT('Ctrl Pts',(93.3223614975481,1.24073392044573,-1.82250633350637));
#10153=CARTESIAN_POINT('Ctrl Pts',(93.3254996483545,1.2880097103385,-1.78940293750926));
#10154=CARTESIAN_POINT('Ctrl Pts',(93.3286377991608,1.33385079356041,-1.75455352170239));
#10155=CARTESIAN_POINT('Ctrl Pts',(93.3327108640952,1.39334879736683,-1.70932180969656));
#10156=CARTESIAN_POINT('Ctrl Pts',(93.3367839290295,1.45065817780139,-1.66097301929738));
#10157=CARTESIAN_POINT('Ctrl Pts',(93.3408569939638,1.50543397192874,-1.60974673665234));
#10158=CARTESIAN_POINT('Ctrl Pts',(93.3449240747671,1.560129289675,-1.55859571546009));
#10159=CARTESIAN_POINT('Ctrl Pts',(93.3489911555705,1.61229806563741,-1.50457591895396));
#10160=CARTESIAN_POINT('Ctrl Pts',(93.3530582363738,1.6616268385985,-1.44796831776429));
#10161=CARTESIAN_POINT('Ctrl Pts',(93.3571205587409,1.71089789748109,-1.3914269467957));
#10162=CARTESIAN_POINT('Ctrl Pts',(93.361182881108,1.75733524284504,-1.33230414464942));
#10163=CARTESIAN_POINT('Ctrl Pts',(93.3652452034752,1.80066205083603,-1.27091784891038));
#10164=CARTESIAN_POINT('Ctrl Pts',(93.3693049476127,1.84396136065031,-1.20957051314292));
#10165=CARTESIAN_POINT('Ctrl Pts',(93.3733646917502,1.88415377597543,-1.14596292359402));
#10166=CARTESIAN_POINT('Ctrl Pts',(93.3774244358877,1.92100344358486,-1.08044517201712));
#10167=CARTESIAN_POINT('Ctrl Pts',(93.3814829153409,1.9578416318513,-1.0149478304138));
#10168=CARTESIAN_POINT('Ctrl Pts',(93.3855413947942,1.99133890600378,-0.947541924111951));
#10169=CARTESIAN_POINT('Ctrl Pts',(93.3895998742474,2.02130421893966,-0.878604151194797));
#10170=CARTESIAN_POINT('Ctrl Pts',(93.393658400878,2.05126988020382,-0.809665576918541));
#10171=CARTESIAN_POINT('Ctrl Pts',(93.3977169275086,2.07770331004053,-0.739195539267929));
#10172=CARTESIAN_POINT('Ctrl Pts',(93.4017754541391,2.10046133286916,-0.667591333917327));
#10173=CARTESIAN_POINT('Ctrl Pts',(93.4058381311224,2.12324262863151,-0.595913904282804));
#10174=CARTESIAN_POINT('Ctrl Pts',(93.4099008081056,2.14234086680234,-0.52310044687806));
#10175=CARTESIAN_POINT('Ctrl Pts',(93.4139634850889,2.15766280910038,-0.449563346176113));
#10176=CARTESIAN_POINT('Ctrl Pts',(93.4180282840641,2.17299275425912,-0.375987836037407));
#10177=CARTESIAN_POINT('Ctrl Pts',(93.4220930830392,2.18454240227297,-0.301688402146922));
#10178=CARTESIAN_POINT('Ctrl Pts',(93.4261578820144,2.1922701575948,-0.227084909492602));
#10179=CARTESIAN_POINT('Ctrl Pts',(93.4302299422546,2.20001171760397,-0.152348146846223));
#10180=CARTESIAN_POINT('Ctrl Pts',(93.4343020024947,2.20391772297867,-0.0773067180315107));
#10181=CARTESIAN_POINT('Ctrl Pts',(93.4383740627349,2.20399871236733,-0.00238241120780133));
#10182=CARTESIAN_POINT('Ctrl Pts',(93.4415122135499,2.20406112718956,0.0553583295131656));
#10183=CARTESIAN_POINT('Ctrl Pts',(93.444650364365,2.2018529080311,0.113029456811266));
#10184=CARTESIAN_POINT('Ctrl Pts',(93.44778851518,2.19739981579467,0.170440750836054));
#10185=CARTESIAN_POINT('Ctrl Pts',(93.4518615801172,2.19162006366708,0.244955948628872));
#10186=CARTESIAN_POINT('Ctrl Pts',(93.4559346450543,2.18203458412387,0.319320518212626));
#10187=CARTESIAN_POINT('Ctrl Pts',(93.4600077099914,2.16865783993518,0.393114707544327));
#10188=CARTESIAN_POINT('Ctrl Pts',(93.4640747907976,2.1553007488062,0.46680047874468));
#10189=CARTESIAN_POINT('Ctrl Pts',(93.4681418716038,2.13816353642985,0.539917067561367));
#10190=CARTESIAN_POINT('Ctrl Pts',(93.4722089524101,2.11731251727188,0.612048776000599));
#10191=CARTESIAN_POINT('Ctrl Pts',(93.4762712747801,2.09648589355834,0.684096091198791));
#10192=CARTESIAN_POINT('Ctrl Pts',(93.4803335971501,2.07195422772864,0.755160358996972));
#10193=CARTESIAN_POINT('Ctrl Pts',(93.4843959195202,2.04383475563522,0.824836645438059));
#10194=CARTESIAN_POINT('Ctrl Pts',(93.4884556636607,2.01573313009541,0.894468710509103));
#10195=CARTESIAN_POINT('Ctrl Pts',(93.4925154078012,1.98404839512368,0.962714100649501));
#10196=CARTESIAN_POINT('Ctrl Pts',(93.4965751519417,1.94894701069206,1.02918489568906));
#10197=CARTESIAN_POINT('Ctrl Pts',(93.5006336313979,1.91385656098102,1.09563498386526));
#10198=CARTESIAN_POINT('Ctrl Pts',(93.5046921108542,1.87535179783926,1.16031115260634));
#10199=CARTESIAN_POINT('Ctrl Pts',(93.5087505903104,1.83364582058261,1.22284872517411));
#10200=CARTESIAN_POINT('Ctrl Pts',(93.512809116944,1.79193935851936,1.28538702470308));
#10201=CARTESIAN_POINT('Ctrl Pts',(93.5168676435776,1.74703187485705,1.34578628246384));
#10202=CARTESIAN_POINT('Ctrl Pts',(93.5209261702112,1.69917971884093,1.40371089725757));
#10203=CARTESIAN_POINT('Ctrl Pts',(93.5249888471975,1.65127862799127,1.46169474723773));
#10204=CARTESIAN_POINT('Ctrl Pts',(93.5290515241838,1.60042715616635,1.51719853180398));
#10205=CARTESIAN_POINT('Ctrl Pts',(93.5331142011701,1.54692139171317,1.56992044634759));
#10206=CARTESIAN_POINT('Ctrl Pts',(93.5371790001484,1.49338768046484,1.62266989827076));
#10207=CARTESIAN_POINT('Ctrl Pts',(93.5412437991266,1.43719727289644,1.67263426908128));
#10208=CARTESIAN_POINT('Ctrl Pts',(93.5453085981049,1.37868052577792,1.71955110649283));
#10209=CARTESIAN_POINT('Ctrl Pts',(93.5493806583481,1.32005924566588,1.76655175508157));
#10210=CARTESIAN_POINT('Ctrl Pts',(93.5534527185913,1.25910371316289,1.81049371659205));
#10211=CARTESIAN_POINT('Ctrl Pts',(93.5575247788346,1.19617414883073,1.85115731521367));
#10212=CARTESIAN_POINT('Ctrl Pts',(93.5606629296228,1.14767720867898,1.88249489286315));
#10213=CARTESIAN_POINT('Ctrl Pts',(93.563801080411,1.09800850212365,1.91188629785332));
#10214=CARTESIAN_POINT('Ctrl Pts',(93.5669392311991,1.04734186562866,1.93925011705594));
#10215=CARTESIAN_POINT('Ctrl Pts',(93.5712291614867,0.97807931161546,1.97665713944072));
#10216=CARTESIAN_POINT('Ctrl Pts',(93.5755190917743,0.906707522894725,2.01040537985972));
#10217=CARTESIAN_POINT('Ctrl Pts',(93.5798090220618,0.833627277572188,2.04026507152565));
#10218=CARTESIAN_POINT('Ctrl Pts',(93.5840864142973,0.760760621716913,2.07003749315565));
#10219=CARTESIAN_POINT('Ctrl Pts',(93.5883638065327,0.686195825607445,2.09594385041639));
#10220=CARTESIAN_POINT('Ctrl Pts',(93.5926411987682,0.610356510638483,2.11780096560588));
#10221=CARTESIAN_POINT('Ctrl Pts',(93.5969110194947,0.534651440558738,2.13961939102071));
#10222=CARTESIAN_POINT('Ctrl Pts',(93.6011808402213,0.457676723409933,2.15740271911496));
#10223=CARTESIAN_POINT('Ctrl Pts',(93.6054506609479,0.379874733097137,2.17101616464604));
#10224=CARTESIAN_POINT('Ctrl Pts',(93.6097108188649,0.302248812427545,2.18459880229562));
#10225=CARTESIAN_POINT('Ctrl Pts',(93.613970976782,0.223799742236276,2.19403028120832));
#10226=CARTESIAN_POINT('Ctrl Pts',(93.618231134699,0.144982223500534,2.19922626277262));
#10227=CARTESIAN_POINT('Ctrl Pts',(93.6208368920538,0.0967729004828302,
2.20240442363896));
#10228=CARTESIAN_POINT('Ctrl Pts',(93.6234426494085,0.0484260077747917,
2.20399895730396));
#10229=CARTESIAN_POINT('Ctrl Pts',(93.6260484067633,4.74792226957855E-5,
2.2039999994886));
#10230=CARTESIAN_POINT('',(94.3760484067719,-0.00198161751639934,2.20399910916316));
#10231=CARTESIAN_POINT('Ctrl Pts',(93.6260484068025,4.74784943464956E-5,
2.20399999948861));
#10232=CARTESIAN_POINT('Ctrl Pts',(93.6302924706585,-0.0787478721400754,
2.20400169689542));
#10233=CARTESIAN_POINT('Ctrl Pts',(93.6345365345146,-0.157464660372779,
2.19977356426505));
#10234=CARTESIAN_POINT('Ctrl Pts',(93.6387805983706,-0.235645064551175,
2.1913665607453));
#10235=CARTESIAN_POINT('Ctrl Pts',(93.6430360559872,-0.314035354545841,
2.18293698749321));
#10236=CARTESIAN_POINT('Ctrl Pts',(93.6472915136038,-0.391885973482654,
2.17030616852904));
#10237=CARTESIAN_POINT('Ctrl Pts',(93.6515469712204,-0.468746913744802,
2.15357663686592));
#10238=CARTESIAN_POINT('Ctrl Pts',(93.6558083437779,-0.545714688092428,
2.13682385172438));
#10239=CARTESIAN_POINT('Ctrl Pts',(93.6600697163354,-0.621689645794342,
2.11596110459831));
#10240=CARTESIAN_POINT('Ctrl Pts',(93.664331088893,-0.696237353990324,2.09114072862363));
#10241=CARTESIAN_POINT('Ctrl Pts',(93.6686040125675,-0.770987135410994,
2.06625307313717));
#10242=CARTESIAN_POINT('Ctrl Pts',(93.6728769362419,-0.844301550522626,
2.03738649373384));
#10243=CARTESIAN_POINT('Ctrl Pts',(93.6771498599164,-0.915765840088244,
2.00474161081359));
#10244=CARTESIAN_POINT('Ctrl Pts',(93.6801298890171,-0.96560657649917,1.98197436559667));
#10245=CARTESIAN_POINT('Ctrl Pts',(93.6831099181177,-1.01454790143108,1.95737035493228));
#10246=CARTESIAN_POINT('Ctrl Pts',(93.6860899472184,-1.06245716940618,1.93101029597913));
#10247=CARTESIAN_POINT('Ctrl Pts',(93.6901630121542,-1.12793893246917,1.89498171095476));
#10248=CARTESIAN_POINT('Ctrl Pts',(93.69423607709,-1.19171226772072,1.85554908062932));
#10249=CARTESIAN_POINT('Ctrl Pts',(93.6983091420258,-1.25340083861911,1.8128988768679));
#10250=CARTESIAN_POINT('Ctrl Pts',(93.7023762228307,-1.31499877691252,1.77031133461759));
#10251=CARTESIAN_POINT('Ctrl Pts',(93.7064433036356,-1.374517642539,1.72451587371866));
#10252=CARTESIAN_POINT('Ctrl Pts',(93.7105103844404,-1.43160619890503,1.67574451849221));
#10253=CARTESIAN_POINT('Ctrl Pts',(93.7145727068091,-1.48862796233871,1.62703022517165));
#10254=CARTESIAN_POINT('Ctrl Pts',(93.7186350291778,-1.54322470456571,1.57534726356366));
#10255=CARTESIAN_POINT('Ctrl Pts',(93.7226973515465,-1.59507601626904,1.52096959283323));
#10256=CARTESIAN_POINT('Ctrl Pts',(93.7267570956856,-1.64689441955874,1.46662643391788));
#10257=CARTESIAN_POINT('Ctrl Pts',(93.7308168398247,-1.69597052134901,1.40959230435394));
#10258=CARTESIAN_POINT('Ctrl Pts',(93.7348765839638,-1.74201973109914,1.35017897201122));
#10259=CARTESIAN_POINT('Ctrl Pts',(93.7389350634187,-1.7880545956816,1.29078414800381));
#10260=CARTESIAN_POINT('Ctrl Pts',(93.7429935428735,-1.83106414807162,1.22901196990301));
#10261=CARTESIAN_POINT('Ctrl Pts',(93.7470520223284,-1.87080422327517,1.16520708810743));
#10262=CARTESIAN_POINT('Ctrl Pts',(93.7511105489606,-1.91054476043274,1.10140146461919));
#10263=CARTESIAN_POINT('Ctrl Pts',(93.7551690755927,-1.94701549404096,1.03556349674723));
#10264=CARTESIAN_POINT('Ctrl Pts',(93.7592276022249,-1.98001659714391,0.968065222510682));
#10265=CARTESIAN_POINT('Ctrl Pts',(93.7632902792098,-2.0130514480154,0.900497922819763));
#10266=CARTESIAN_POINT('Ctrl Pts',(93.7673529561947,-2.04260937278205,0.831267356102898));
#10267=CARTESIAN_POINT('Ctrl Pts',(93.7714156331796,-2.06853773294696,0.76076780122101));
#10268=CARTESIAN_POINT('Ctrl Pts',(93.7754804321565,-2.09447963585023,0.69023142345406));
#10269=CARTESIAN_POINT('Ctrl Pts',(93.7795452311333,-2.11678805711947,0.618425193987838));
#10270=CARTESIAN_POINT('Ctrl Pts',(93.7836100301101,-2.13536034821463,0.545758356118066));
#10271=CARTESIAN_POINT('Ctrl Pts',(93.7876820903519,-2.15396581643057,0.47296170785255));
#10272=CARTESIAN_POINT('Ctrl Pts',(93.7917541505937,-2.16882172886429,0.399301849134778));
#10273=CARTESIAN_POINT('Ctrl Pts',(93.7958262108356,-2.17987672713035,0.325197562284023));
#10274=CARTESIAN_POINT('Ctrl Pts',(93.7989643616362,-2.18839630925815,0.268088773783823));
#10275=CARTESIAN_POINT('Ctrl Pts',(93.8021025124368,-2.19465955223917,0.210716246280975));
#10276=CARTESIAN_POINT('Ctrl Pts',(93.8052406632374,-2.19866407578353,0.153271921299827));
#10277=CARTESIAN_POINT('Ctrl Pts',(93.8093137281735,-2.20386162219569,0.0787138516827568));
#10278=CARTESIAN_POINT('Ctrl Pts',(93.8133867931097,-2.20527242698567,0.00374732412319403));
#10279=CARTESIAN_POINT('Ctrl Pts',(93.8174598580458,-2.20284931181229,-0.0712103184104735));
#10280=CARTESIAN_POINT('Ctrl Pts',(93.821526938851,-2.20042975667016,-0.146057833471603));
#10281=CARTESIAN_POINT('Ctrl Pts',(93.8255940196562,-2.19418748022996,-0.220896016174146));
#10282=CARTESIAN_POINT('Ctrl Pts',(93.8296611004614,-2.18412719039319,-0.295303938655015));
#10283=CARTESIAN_POINT('Ctrl Pts',(93.8337234228304,-2.17407867097592,-0.369624804751169));
#10284=CARTESIAN_POINT('Ctrl Pts',(93.8377857451995,-2.16022107678299,-0.443515939987352));
#10285=CARTESIAN_POINT('Ctrl Pts',(93.8418480675685,-2.14261106456059,-0.516559605488601));
#10286=CARTESIAN_POINT('Ctrl Pts',(93.845907811708,-2.12501222886481,-0.589556912448955));
#10287=CARTESIAN_POINT('Ctrl Pts',(93.8499675558474,-2.10366581267472,-0.661707354019261));
#10288=CARTESIAN_POINT('Ctrl Pts',(93.8540272999869,-2.07867965808225,-0.732602811266139));
#10289=CARTESIAN_POINT('Ctrl Pts',(93.8580857794421,-2.05370128713207,-0.803476183286705));
#10290=CARTESIAN_POINT('Ctrl Pts',(93.8621442588973,-2.02508558758278,-0.873094897180993));
#10291=CARTESIAN_POINT('Ctrl Pts',(93.8662027383525,-1.99298994249238,-0.941066995024375));
#10292=CARTESIAN_POINT('Ctrl Pts',(93.8702612649851,-1.96089392430978,-1.00903988300173));
#10293=CARTESIAN_POINT('Ctrl Pts',(93.8743197916176,-1.92531808575484,-1.07536568593995));
#10294=CARTESIAN_POINT('Ctrl Pts',(93.8783783182502,-1.88646685228122,-1.13967487260368));
#10295=CARTESIAN_POINT('Ctrl Pts',(93.8824409952354,-1.84757588854667,-1.20404982347969));
#10296=CARTESIAN_POINT('Ctrl Pts',(93.8865036722207,-1.80540308856911,-1.26640363031909));
#10297=CARTESIAN_POINT('Ctrl Pts',(93.890566349206,-1.76019713877674,-1.32639437296838));
#10298=CARTESIAN_POINT('Ctrl Pts',(93.8946311481832,-1.71496757729636,-1.38641644960591));
#10299=CARTESIAN_POINT('Ctrl Pts',(93.8986959471604,-1.66670201787713,-1.44407263769095));
#10300=CARTESIAN_POINT('Ctrl Pts',(93.9027607461376,-1.61568881005288,-1.49905492530124));
#10301=CARTESIAN_POINT('Ctrl Pts',(93.9068328063798,-1.56458447338786,-1.55413543202667));
#10302=CARTESIAN_POINT('Ctrl Pts',(93.9109048666219,-1.51072302704085,-1.60653216397486));
#10303=CARTESIAN_POINT('Ctrl Pts',(93.9149769268641,-1.45442862809842,-1.65597504986269));
#10304=CARTESIAN_POINT('Ctrl Pts',(93.9181150776616,-1.41104510663045,-1.69407842322932));
#10305=CARTESIAN_POINT('Ctrl Pts',(93.9212532284591,-1.36621738319208,-1.7304282558195));
#10306=CARTESIAN_POINT('Ctrl Pts',(93.9243913792565,-1.32010549383252,-1.76491854915551));
#10307=CARTESIAN_POINT('Ctrl Pts',(93.9284644441925,-1.26025600545494,-1.809684149499));
#10308=CARTESIAN_POINT('Ctrl Pts',(93.9325375091285,-1.19801147619516,-1.8514883263379));
#10309=CARTESIAN_POINT('Ctrl Pts',(93.9366105740644,-1.13369711820735,-1.89006530156192));
#10310=CARTESIAN_POINT('Ctrl Pts',(93.9406776548695,-1.06947725062046,-1.9285855996462));
#10311=CARTESIAN_POINT('Ctrl Pts',(93.9447447356745,-1.00319399795282,-1.9638878661549));
#10312=CARTESIAN_POINT('Ctrl Pts',(93.9488118164795,-0.935203698473259,
-1.9957479906947));
#10313=CARTESIAN_POINT('Ctrl Pts',(93.9528741388484,-0.867292946835827,
-2.02757083926754));
#10314=CARTESIAN_POINT('Ctrl Pts',(93.9569364612172,-0.797679546589344,
-2.05595934554963));
#10315=CARTESIAN_POINT('Ctrl Pts',(93.960998783586,-0.726745302627086,-2.08073478970999));
#10316=CARTESIAN_POINT('Ctrl Pts',(93.9650585277253,-0.655856078421628,
-2.10549450966708));
#10317=CARTESIAN_POINT('Ctrl Pts',(93.9691182718646,-0.583648123627884,
-2.12664556086921));
#10318=CARTESIAN_POINT('Ctrl Pts',(93.9731780160039,-0.51052289090503,-2.14405745675389));
#10319=CARTESIAN_POINT('Ctrl Pts',(93.9772364954589,-0.437420438024153,
-2.16146392851585));
#10320=CARTESIAN_POINT('Ctrl Pts',(93.9812949749139,-0.363401738728236,
-2.17513344712636));
#10321=CARTESIAN_POINT('Ctrl Pts',(93.9853534543689,-0.288881504754601,
-2.18498592128433));
#10322=CARTESIAN_POINT('Ctrl Pts',(93.9894119810013,-0.214360404529088,
-2.19483850997124));
#10323=CARTESIAN_POINT('Ctrl Pts',(93.9934705076336,-0.139338231626751,
-2.2008739053018));
#10324=CARTESIAN_POINT('Ctrl Pts',(93.997529034266,-0.0642363368181861,
-2.20306370607665));
#10325=CARTESIAN_POINT('Ctrl Pts',(94.001591711251,0.0109423591011084,-2.20525574619755));
#10326=CARTESIAN_POINT('Ctrl Pts',(94.0056543882361,0.0862004614105676,
-2.20359432463246));
#10327=CARTESIAN_POINT('Ctrl Pts',(94.0097170652212,0.161115844789395,-2.19810320152576));
#10328=CARTESIAN_POINT('Ctrl Pts',(94.0137818641982,0.236070357501068,-2.19260921033011));
#10329=CARTESIAN_POINT('Ctrl Pts',(94.0178466631752,0.310681320593962,-2.18328159346358));
#10330=CARTESIAN_POINT('Ctrl Pts',(94.0219114621522,0.384533618134413,-2.17019581985692));
#10331=CARTESIAN_POINT('Ctrl Pts',(94.0259835223942,0.458517843748993,-2.15708667012023));
#10332=CARTESIAN_POINT('Ctrl Pts',(94.0300555826361,0.531740230831165,-2.1402060613951));
#10333=CARTESIAN_POINT('Ctrl Pts',(94.0341276428781,0.603798151067578,-2.11968011567014));
#10334=CARTESIAN_POINT('Ctrl Pts',(94.0372657936773,0.659329898276897,-2.10386170701373));
#10335=CARTESIAN_POINT('Ctrl Pts',(94.0404039444765,0.714170302893095,-2.0858793505723));
#10336=CARTESIAN_POINT('Ctrl Pts',(94.0435420952757,0.768143562992485,-2.06581012356732));
#10337=CARTESIAN_POINT('Ctrl Pts',(94.0476151602117,0.838196472255843,-2.03976189643083));
#10338=CARTESIAN_POINT('Ctrl Pts',(94.0516882251476,0.907058004530739,-2.01009609125474));
#10339=CARTESIAN_POINT('Ctrl Pts',(94.0557612900836,0.974328568233429,-1.97694204293505));
#10340=CARTESIAN_POINT('Ctrl Pts',(94.0598283708887,1.04150029828942,-1.9438367044123));
#10341=CARTESIAN_POINT('Ctrl Pts',(94.0638954516937,1.10708527583775,-1.90725350710972));
#10342=CARTESIAN_POINT('Ctrl Pts',(94.0679625324988,1.17070206600156,-1.86737052366682));
#10343=CARTESIAN_POINT('Ctrl Pts',(94.0720248548676,1.23424442527713,-1.82753420284043));
#10344=CARTESIAN_POINT('Ctrl Pts',(94.0760871772365,1.2958227697159,-1.78440601856351));
#10345=CARTESIAN_POINT('Ctrl Pts',(94.0801494996053,1.35508001660587,-1.73821004156443));
#10346=CARTESIAN_POINT('Ctrl Pts',(94.0842092437446,1.41429965476574,-1.69204338371402));
#10347=CARTESIAN_POINT('Ctrl Pts',(94.0882689878839,1.47120074304027,-1.64281308962916));
#10348=CARTESIAN_POINT('Ctrl Pts',(94.0923287320232,1.5254560929374,-1.59078587764669));
#10349=CARTESIAN_POINT('Ctrl Pts',(94.0963872114782,1.5796945413047,-1.53877487308852));
#10350=CARTESIAN_POINT('Ctrl Pts',(94.1004456909333,1.63128854330689,-1.4839690107931));
#10351=CARTESIAN_POINT('Ctrl Pts',(94.1045041703883,1.6799460833365,-1.42667345846285));
#10352=CARTESIAN_POINT('Ctrl Pts',(94.1085626970207,1.72860418898035,-1.36937724010674));
#10353=CARTESIAN_POINT('Ctrl Pts',(94.1126212236531,1.77432545717723,-1.30959163934571));
#10354=CARTESIAN_POINT('Ctrl Pts',(94.1166797502854,1.81685772038635,-1.24765541070943));
#10355=CARTESIAN_POINT('Ctrl Pts',(94.1207424272705,1.859433478171,-1.18565584450841));
#10356=CARTESIAN_POINT('Ctrl Pts',(94.1248051042556,1.8988134477374,-1.1215016530489));
#10357=CARTESIAN_POINT('Ctrl Pts',(94.1288677812407,1.93478888318488,-1.05556050395238));
#10358=CARTESIAN_POINT('Ctrl Pts',(94.1329325802177,1.97078310909609,-0.989584912888582));
#10359=CARTESIAN_POINT('Ctrl Pts',(94.1369973791947,2.00336905259656,-0.921820936202544));
#10360=CARTESIAN_POINT('Ctrl Pts',(94.1410621781718,2.03238522655091,-0.852658367048386));
#10361=CARTESIAN_POINT('Ctrl Pts',(94.1451342384138,2.06145323434216,-0.783372247444925));
#10362=CARTESIAN_POINT('Ctrl Pts',(94.1492062986557,2.08693857293896,-0.712682994813434));
#10363=CARTESIAN_POINT('Ctrl Pts',(94.1532783588977,2.10872909485679,-0.64099735140206));
#10364=CARTESIAN_POINT('Ctrl Pts',(94.1564165096968,2.12552205461277,-0.585752500937799));
#10365=CARTESIAN_POINT('Ctrl Pts',(94.1595546604958,2.14012164517855,-0.529916248586732));
#10366=CARTESIAN_POINT('Ctrl Pts',(94.1626928112948,2.15249739642118,-0.473678116868447));
#10367=CARTESIAN_POINT('Ctrl Pts',(94.1667658762308,2.16856011668904,-0.400685588134812));
#10368=CARTESIAN_POINT('Ctrl Pts',(94.1708389411669,2.18093677105545,-0.326734326814922));
#10369=CARTESIAN_POINT('Ctrl Pts',(94.1749120061029,2.18951955782837,-0.252230263622469));
#10370=CARTESIAN_POINT('Ctrl Pts',(94.178979086908,2.19808973480484,-0.177835661505563));
#10371=CARTESIAN_POINT('Ctrl Pts',(94.1830461677131,2.20287705653575,-0.102890340399728));
#10372=CARTESIAN_POINT('Ctrl Pts',(94.1871132485181,2.20382452279676,-0.0278113775216291));
#10373=CARTESIAN_POINT('Ctrl Pts',(94.191175570887,2.2047708805335,0.047179743862388));
#10374=CARTESIAN_POINT('Ctrl Pts',(94.1952378932559,2.20188630254724,0.122303721344895));
#10375=CARTESIAN_POINT('Ctrl Pts',(94.1993002156248,2.19516564424378,0.197139022853949));
#10376=CARTESIAN_POINT('Ctrl Pts',(94.2033599597641,2.18844925133294,0.271926828726487));
#10377=CARTESIAN_POINT('Ctrl Pts',(94.2074197039035,2.17790165198512,0.346425847851594));
#10378=CARTESIAN_POINT('Ctrl Pts',(94.2114794480428,2.16356974397609,0.420216566726289));
#10379=CARTESIAN_POINT('Ctrl Pts',(94.2155379274979,2.14924230061747,0.493984298447898));
#10380=CARTESIAN_POINT('Ctrl Pts',(94.219596406953,2.13113298018927,0.567043699610763));
#10381=CARTESIAN_POINT('Ctrl Pts',(94.223654886408,2.10934005432727,0.638983986662144));
#10382=CARTESIAN_POINT('Ctrl Pts',(94.2277134130404,2.08754687513587,0.710925109975224));
#10383=CARTESIAN_POINT('Ctrl Pts',(94.2317719396729,2.06207014563213,0.781746636912583));
#10384=CARTESIAN_POINT('Ctrl Pts',(94.2358304663053,2.03305795748616,0.851053077958238));
#10385=CARTESIAN_POINT('Ctrl Pts',(94.2398931432904,2.00401610073764,0.92043039353579));
#10386=CARTESIAN_POINT('Ctrl Pts',(94.2439558202755,1.97143175027588,0.988289087819992));
#10387=CARTESIAN_POINT('Ctrl Pts',(94.2480184972606,1.93550082579324,1.05425450122524));
#10388=CARTESIAN_POINT('Ctrl Pts',(94.2520832962377,1.8995511340956,1.12025436927126));
#10389=CARTESIAN_POINT('Ctrl Pts',(94.2561480952148,1.86025163726231,1.18435857973248));
#10390=CARTESIAN_POINT('Ctrl Pts',(94.2602128941918,1.81784245713697,1.24622020567403));
#10391=CARTESIAN_POINT('Ctrl Pts',(94.2642849544339,1.77535751821137,1.30819233982512));
#10392=CARTESIAN_POINT('Ctrl Pts',(94.2683570146759,1.72975209038513,1.36791350754539));
#10393=CARTESIAN_POINT('Ctrl Pts',(94.2724290749179,1.6813072743529,1.42506906822372));
#10394=CARTESIAN_POINT('Ctrl Pts',(94.2755672257166,1.64397306781175,1.46911624771802));
#10395=CARTESIAN_POINT('Ctrl Pts',(94.2787053765153,1.60495337895619,1.51164034679363));
#10396=CARTESIAN_POINT('Ctrl Pts',(94.281843527314,1.56439099102276,1.55251306828858));
#10397=CARTESIAN_POINT('Ctrl Pts',(94.2858578104481,1.51250409322624,1.60479694088391));
#10398=CARTESIAN_POINT('Ctrl Pts',(94.2898720935823,1.45787927345134,1.6545912562367));
#10399=CARTESIAN_POINT('Ctrl Pts',(94.2938863767164,1.40078855700466,1.70158967397102));
#10400=CARTESIAN_POINT('Ctrl Pts',(94.2978953705898,1.34377306387337,1.74852616610658));
#10401=CARTESIAN_POINT('Ctrl Pts',(94.3019043644632,1.28429848979287,1.79267375274742));
#10402=CARTESIAN_POINT('Ctrl Pts',(94.3059133583366,1.22267430555594,1.83376212812167));
#10403=CARTESIAN_POINT('Ctrl Pts',(94.3099184525911,1.16111006424676,1.87481053611059));
#10404=CARTESIAN_POINT('Ctrl Pts',(94.3139235468457,1.09740076587819,1.91280536170242));
#10405=CARTESIAN_POINT('Ctrl Pts',(94.3179286411002,1.03188823788919,1.94751705114639));
#10406=CARTESIAN_POINT('Ctrl Pts',(94.321931219972,0.966416854769319,1.98220694005903));
#10407=CARTESIAN_POINT('Ctrl Pts',(94.3259337988439,0.899144922756926,2.01361755394063));
#10408=CARTESIAN_POINT('Ctrl Pts',(94.3299363777157,0.830440935359365,2.04156407023622));
#10409=CARTESIAN_POINT('Ctrl Pts',(94.3339394248967,0.76172890946859,2.06951385632575));
#10410=CARTESIAN_POINT('Ctrl Pts',(94.3379424720776,0.691584942794871,2.09399853324094));
#10411=CARTESIAN_POINT('Ctrl Pts',(94.3419455192586,0.620398482558594,2.11488101860105));
#10412=CARTESIAN_POINT('Ctrl Pts',(94.3459485969863,0.549211479107214,2.13576366331282));
#10413=CARTESIAN_POINT('Ctrl Pts',(94.349951674714,0.476982441804223,2.15304393266763));
#10414=CARTESIAN_POINT('Ctrl Pts',(94.3539547524417,0.404114697745888,2.16663502027124));
#10415=CARTESIAN_POINT('Ctrl Pts',(94.3579621228321,0.331168814648818,2.18024068214958));
#10416=CARTESIAN_POINT('Ctrl Pts',(94.3619694932225,0.257583343810738,2.19014918215616));
#10417=CARTESIAN_POINT('Ctrl Pts',(94.3659768636129,0.183769558616102,2.19632528313227));
#10418=CARTESIAN_POINT('Ctrl Pts',(94.3693340446659,0.12193194018719,2.2014993217557));
#10419=CARTESIAN_POINT('Ctrl Pts',(94.3726912257189,0.0599343460611356,
2.20405477785988));
#10420=CARTESIAN_POINT('Ctrl Pts',(94.3760484067719,-0.00198161751640419,
2.20399910916316));
#10421=CARTESIAN_POINT('',(95.1260484068548,0.00109146085463435,2.20399972974436));
#10422=CARTESIAN_POINT('Ctrl Pts',(94.3760484068025,-0.00198161808060188,
2.20399910916266));
#10423=CARTESIAN_POINT('Ctrl Pts',(94.3817549998797,-0.107227419108485,
2.20390448254445));
#10424=CARTESIAN_POINT('Ctrl Pts',(94.3874615929569,-0.212146408604953,
2.19626776901676));
#10425=CARTESIAN_POINT('Ctrl Pts',(94.3931681860342,-0.31586069941933,2.18124918763591));
#10426=CARTESIAN_POINT('Ctrl Pts',(94.3957768718005,-0.363272174278653,
2.17438366227803));
#10427=CARTESIAN_POINT('Ctrl Pts',(94.3983855575668,-0.410432337347612,
2.16597614678547));
#10428=CARTESIAN_POINT('Ctrl Pts',(94.4009942433332,-0.457259089225866,
2.1560450193167));
#10429=CARTESIAN_POINT('Ctrl Pts',(94.4050673082692,-0.530371920063354,
2.14053907851307));
#10430=CARTESIAN_POINT('Ctrl Pts',(94.4091403732052,-0.602836125855812,
2.12128006755923));
#10431=CARTESIAN_POINT('Ctrl Pts',(94.4132134381412,-0.674237480213912,
2.09833739428977));
#10432=CARTESIAN_POINT('Ctrl Pts',(94.4172805189463,-0.745533931983874,
2.07542842830538));
#10433=CARTESIAN_POINT('Ctrl Pts',(94.4213475997513,-0.815770181810802,
2.04884668992764));
#10434=CARTESIAN_POINT('Ctrl Pts',(94.4254146805564,-0.884542825083242,
2.01871245862152));
#10435=CARTESIAN_POINT('Ctrl Pts',(94.4294770029253,-0.953235005180726,
1.98861348400775));
#10436=CARTESIAN_POINT('Ctrl Pts',(94.4335393252941,-1.02046654575262,1.9549704648919));
#10437=CARTESIAN_POINT('Ctrl Pts',(94.437601647663,-1.08585139390071,1.91795274977354));
#10438=CARTESIAN_POINT('Ctrl Pts',(94.4416613918023,-1.15119474432084,1.88095852864676));
#10439=CARTESIAN_POINT('Ctrl Pts',(94.4457211359416,-1.2146933136601,1.84059409635276));
#10440=CARTESIAN_POINT('Ctrl Pts',(94.4497808800809,-1.2759843737873,1.79707536788267));
#10441=CARTESIAN_POINT('Ctrl Pts',(94.453839359536,-1.33725634063282,1.75357019628922));
#10442=CARTESIAN_POINT('Ctrl Pts',(94.457897838991,-1.39632177457106,1.70691295571196));
#10443=CARTESIAN_POINT('Ctrl Pts',(94.4619563184461,-1.45284710892216,1.65736274789091));
#10444=CARTESIAN_POINT('Ctrl Pts',(94.4660148450784,-1.50937310034565,1.60781196407905));
#10445=CARTESIAN_POINT('Ctrl Pts',(94.4700733717108,-1.5633585756961,1.55536846233581));
#10446=CARTESIAN_POINT('Ctrl Pts',(94.4741318983432,-1.61450446676175,1.50033040587943));
#10447=CARTESIAN_POINT('Ctrl Pts',(94.4781945753283,-1.66570266091831,1.44523606610469));
#10448=CARTESIAN_POINT('Ctrl Pts',(94.4822572523134,-1.71405514626068,1.38754222374569));
#10449=CARTESIAN_POINT('Ctrl Pts',(94.4863199292985,-1.7593015726799,1.32758200363143));
#10450=CARTESIAN_POINT('Ctrl Pts',(94.4903847282755,-1.80457163192863,1.26759046547126));
#10451=CARTESIAN_POINT('Ctrl Pts',(94.4944495272525,-1.84673213356332,1.20533058792501));
#10452=CARTESIAN_POINT('Ctrl Pts',(94.4985143262296,-1.88556623555352,1.14116430514652));
#10453=CARTESIAN_POINT('Ctrl Pts',(94.5025863864716,-1.92446970990525,1.07688339717164));
#10454=CARTESIAN_POINT('Ctrl Pts',(94.5066584467136,-1.96003468920312,1.01068970284516));
#10455=CARTESIAN_POINT('Ctrl Pts',(94.5107305069556,-1.9920906561783,0.942969149849091));
#10456=CARTESIAN_POINT('Ctrl Pts',(94.5138686577544,-2.01679472546827,0.890780013428237));
#10457=CARTESIAN_POINT('Ctrl Pts',(94.5170068085533,-2.03941571223733,0.837684570322939));
#10458=CARTESIAN_POINT('Ctrl Pts',(94.5201449593522,-2.05989571383001,0.78386583555145));
#10459=CARTESIAN_POINT('Ctrl Pts',(94.5242180242882,-2.08647709303151,0.714013487609342));
#10460=CARTESIAN_POINT('Ctrl Pts',(94.5282910892241,-2.1095526001422,0.642672814808761));
#10461=CARTESIAN_POINT('Ctrl Pts',(94.5323641541601,-2.1289561356839,0.570229578620661));
#10462=CARTESIAN_POINT('Ctrl Pts',(94.5364312349652,-2.14833116362775,0.497892775749264));
#10463=CARTESIAN_POINT('Ctrl Pts',(94.5404983157703,-2.164044808468,0.424457082991674));
#10464=CARTESIAN_POINT('Ctrl Pts',(94.5445653965753,-2.17597959149856,0.350326729470851));
#10465=CARTESIAN_POINT('Ctrl Pts',(94.5486277189442,-2.18790041097486,0.276283107582392));
#10466=CARTESIAN_POINT('Ctrl Pts',(94.5526900413131,-2.19605107709203,0.201546908690907));
#10467=CARTESIAN_POINT('Ctrl Pts',(94.556752363682,-2.20036475489787,0.126534364515138));
#10468=CARTESIAN_POINT('Ctrl Pts',(94.5608121078213,-2.20467569494667,0.0515694284663048));
#10469=CARTESIAN_POINT('Ctrl Pts',(94.5648718519606,-2.20515445176705,-0.0236710293636508));
#10470=CARTESIAN_POINT('Ctrl Pts',(94.5689315960999,-2.20178596711089,-0.0987651509065199));
#10471=CARTESIAN_POINT('Ctrl Pts',(94.572990075555,-2.19841853179905,-0.173835879262582));
#10472=CARTESIAN_POINT('Ctrl Pts',(94.57704855501,-2.19120625593485,-0.248759885171571));
#10473=CARTESIAN_POINT('Ctrl Pts',(94.5811070344651,-2.18018617975546,-0.323116421129124));
#10474=CARTESIAN_POINT('Ctrl Pts',(94.5851655610975,-2.16916597547443,-0.397473821435904));
#10475=CARTESIAN_POINT('Ctrl Pts',(94.5892240877299,-2.15433795476321,-0.47126326665469));
#10476=CARTESIAN_POINT('Ctrl Pts',(94.5932826143623,-2.13579068078345,-0.544071840732983));
#10477=CARTESIAN_POINT('Ctrl Pts',(94.5973452913474,-2.11722443988891,-0.616954870713584));
#10478=CARTESIAN_POINT('Ctrl Pts',(94.6014079683325,-2.09493146867303,-0.688854562780362));
#10479=CARTESIAN_POINT('Ctrl Pts',(94.6054706453176,-2.06905069359172,-0.759371600303586));
#10480=CARTESIAN_POINT('Ctrl Pts',(94.6095354442947,-2.04315640062639,-0.829925469843297));
#10481=CARTESIAN_POINT('Ctrl Pts',(94.6136002432717,-2.01367075939374,-0.899094807061877));
#10482=CARTESIAN_POINT('Ctrl Pts',(94.6176650422488,-1.98078048399045,-0.966501254133985));
#10483=CARTESIAN_POINT('Ctrl Pts',(94.6217371024908,-1.947831454143,-1.03402811455874));
#10484=CARTESIAN_POINT('Ctrl Pts',(94.6258091627328,-1.91146587328994,-1.09978537613696));
#10485=CARTESIAN_POINT('Ctrl Pts',(94.6298812229749,-1.87191572165627,-1.16342061655108));
#10486=CARTESIAN_POINT('Ctrl Pts',(94.6330193737737,-1.84143622661748,-1.21246138919992));
#10487=CARTESIAN_POINT('Ctrl Pts',(94.6361575245726,-1.80906632918666,-1.26024239862049));
#10488=CARTESIAN_POINT('Ctrl Pts',(94.6392956753715,-1.77492847957935,-1.30661581667226));
#10489=CARTESIAN_POINT('Ctrl Pts',(94.6433687403075,-1.7306203225984,-1.36680474803195));
#10490=CARTESIAN_POINT('Ctrl Pts',(94.6474418052434,-1.68316168372401,-1.42485341916433));
#10491=CARTESIAN_POINT('Ctrl Pts',(94.6515148701794,-1.6327867971314,-1.48041321093585));
#10492=CARTESIAN_POINT('Ctrl Pts',(94.6555819509845,-1.58248592112336,-1.53589137448057));
#10493=CARTESIAN_POINT('Ctrl Pts',(94.6596490317896,-1.5292776220016,-1.58888756782984));
#10494=CARTESIAN_POINT('Ctrl Pts',(94.6637161125946,-1.47343799962834,-1.63908403117449));
#10495=CARTESIAN_POINT('Ctrl Pts',(94.6677784349635,-1.41766370894944,-1.68922176525376));
#10496=CARTESIAN_POINT('Ctrl Pts',(94.6718407573323,-1.35926456482471,-1.73656595970663));
#10497=CARTESIAN_POINT('Ctrl Pts',(94.6759030797012,-1.2985541950541,-1.78083491725298));
#10498=CARTESIAN_POINT('Ctrl Pts',(94.6799628238405,-1.2378823562655,-1.82507577866988));
#10499=CARTESIAN_POINT('Ctrl Pts',(94.6840225679798,-1.17490258747322,-1.86624499563372));
#10500=CARTESIAN_POINT('Ctrl Pts',(94.6880823121191,-1.10996129907252,-1.90410134041265));
#10501=CARTESIAN_POINT('Ctrl Pts',(94.6921407915742,-1.04504024106613,-1.94194589225059));
#10502=CARTESIAN_POINT('Ctrl Pts',(94.6961992710292,-0.978159288886569,
-1.97647938063708));
#10503=CARTESIAN_POINT('Ctrl Pts',(94.7002577504843,-0.909692147535444,
-2.00750496804176));
#10504=CARTESIAN_POINT('Ctrl Pts',(94.7043162771167,-0.841224210295729,
-2.0385309160999));
#10505=CARTESIAN_POINT('Ctrl Pts',(94.708374803749,-0.771170482907496,-2.06604868677474));
#10506=CARTESIAN_POINT('Ctrl Pts',(94.7124333303814,-0.699926004260587,
-2.08990899049691));
#10507=CARTESIAN_POINT('Ctrl Pts',(94.7164960073665,-0.628608669195191,
-2.1137936943734));
#10508=CARTESIAN_POINT('Ctrl Pts',(94.7205586843516,-0.556098604959127,
-2.13401331032924));
#10509=CARTESIAN_POINT('Ctrl Pts',(94.7246213613367,-0.482806708072885,
-2.15046824729867));
#10510=CARTESIAN_POINT('Ctrl Pts',(94.7286861603137,-0.409476529823017,
-2.16693177890752));
#10511=CARTESIAN_POINT('Ctrl Pts',(94.7327509592908,-0.335364176754445,
-2.17962663506225));
#10512=CARTESIAN_POINT('Ctrl Pts',(94.7368157582678,-0.260888821958733,
-2.18850474584292));
#10513=CARTESIAN_POINT('Ctrl Pts',(94.7408878185098,-0.186280426073485,
-2.19739871627991));
#10514=CARTESIAN_POINT('Ctrl Pts',(94.7449598787518,-0.11130821029882,-2.20246229040065));
#10515=CARTESIAN_POINT('Ctrl Pts',(94.7490319389938,-0.0363940751997966,
-2.20369949659439));
#10516=CARTESIAN_POINT('Ctrl Pts',(94.7521700897927,0.0213388263136973,
-2.20465295488688));
#10517=CARTESIAN_POINT('Ctrl Pts',(94.7553082405916,0.0790371629527067,
-2.20333497533854));
#10518=CARTESIAN_POINT('Ctrl Pts',(94.7584463913905,0.136510339980724,-2.19976838032515));
#10519=CARTESIAN_POINT('Ctrl Pts',(94.7625194563265,0.211105857250251,-2.19513922958611));
#10520=CARTESIAN_POINT('Ctrl Pts',(94.7665925212625,0.28560949395828,-2.18670248013346));
#10521=CARTESIAN_POINT('Ctrl Pts',(94.7706655861985,0.359601324857395,-2.17446611543174));
#10522=CARTESIAN_POINT('Ctrl Pts',(94.7747326670035,0.43348444725053,-2.16224772834876));
#10523=CARTESIAN_POINT('Ctrl Pts',(94.7787997478086,0.506856789596386,-2.14624088657335));
#10524=CARTESIAN_POINT('Ctrl Pts',(94.7828668286137,0.579301680042337,-2.12650548165297));
#10525=CARTESIAN_POINT('Ctrl Pts',(94.7869291509825,0.651661810827729,-2.10679316692173));
#10526=CARTESIAN_POINT('Ctrl Pts',(94.7909914733514,0.723096187216718,-2.0833610809537));
#10527=CARTESIAN_POINT('Ctrl Pts',(94.7950537957203,0.79319811429643,-2.05632019672924));
#10528=CARTESIAN_POINT('Ctrl Pts',(94.7991135398596,0.863255549865023,-2.02929647451232));
#10529=CARTESIAN_POINT('Ctrl Pts',(94.8031732839989,0.931981769914055,-1.99866867047218));
#10530=CARTESIAN_POINT('Ctrl Pts',(94.8072330281382,0.998986331668492,-1.9645972384027));
#10531=CARTESIAN_POINT('Ctrl Pts',(94.8112915075933,1.06597002028138,-1.93053642020497));
#10532=CARTESIAN_POINT('Ctrl Pts',(94.8153499870483,1.13123269013548,-1.89303432015572));
#10533=CARTESIAN_POINT('Ctrl Pts',(94.8194084665034,1.19440641938499,-1.85229838452986));
#10534=CARTESIAN_POINT('Ctrl Pts',(94.8234669931358,1.25758088299038,-1.81156197537371));
#10535=CARTESIAN_POINT('Ctrl Pts',(94.8275255197682,1.31866595747844,-1.76759191625749));
#10536=CARTESIAN_POINT('Ctrl Pts',(94.8315840464006,1.37732212565063,-1.72063934692696));
#10537=CARTESIAN_POINT('Ctrl Pts',(94.8356467233857,1.43603827711441,-1.6736387627031));
#10538=CARTESIAN_POINT('Ctrl Pts',(94.8397094003708,1.49232018855618,-1.62364987664444));
#10539=CARTESIAN_POINT('Ctrl Pts',(94.8437720773559,1.54586152209201,-1.57096408441294));
#10540=CARTESIAN_POINT('Ctrl Pts',(94.8478368763329,1.59943082100116,-1.51825077366908));
#10541=CARTESIAN_POINT('Ctrl Pts',(94.85190167531,1.65025636839036,-1.46283810379346));
#10542=CARTESIAN_POINT('Ctrl Pts',(94.855966474287,1.69807064518424,-1.40505234207256));
#10543=CARTESIAN_POINT('Ctrl Pts',(94.8600385345291,1.74597033632085,-1.34716335317376));
#10544=CARTESIAN_POINT('Ctrl Pts',(94.8641105947711,1.79084772662142,-1.28689318840831));
#10545=CARTESIAN_POINT('Ctrl Pts',(94.8681826550131,1.83247760753661,-1.22459863542178));
#10546=CARTESIAN_POINT('Ctrl Pts',(94.871320805812,1.8645598549217,-1.17659106932453));
#10547=CARTESIAN_POINT('Ctrl Pts',(94.8744589566109,1.8947142439976,-1.12738184315265));
#10548=CARTESIAN_POINT('Ctrl Pts',(94.8775971074097,1.92285668869812,-1.0771435163101));
#10549=CARTESIAN_POINT('Ctrl Pts',(94.8816701723457,1.95938329690438,-1.01193824715018));
#10550=CARTESIAN_POINT('Ctrl Pts',(94.8857432372817,1.99265985766841,-0.944747167922621));
#10551=CARTESIAN_POINT('Ctrl Pts',(94.8898163022177,2.02246555692644,-0.875927548970939));
#10552=CARTESIAN_POINT('Ctrl Pts',(94.8938833830228,2.05222746576875,-0.807209039531793));
#10553=CARTESIAN_POINT('Ctrl Pts',(94.8979504638278,2.07852844926698,-0.736867175240501));
#10554=CARTESIAN_POINT('Ctrl Pts',(94.9020175446329,2.10119308455649,-0.665284616846028));
#10555=CARTESIAN_POINT('Ctrl Pts',(94.9060798670018,2.12383120249215,-0.59378580919392));
#10556=CARTESIAN_POINT('Ctrl Pts',(94.9101421893706,2.14284128150927,-0.52104964433311));
#10557=CARTESIAN_POINT('Ctrl Pts',(94.9142045117395,2.15809623810248,-0.447478074421437));
#10558=CARTESIAN_POINT('Ctrl Pts',(94.9182642558788,2.17334151284958,-0.373953198095192));
#10559=CARTESIAN_POINT('Ctrl Pts',(94.9223240000181,2.18483629780017,-0.29959443518531));
#10560=CARTESIAN_POINT('Ctrl Pts',(94.9263837441574,2.19250390352807,-0.224816887742446));
#10561=CARTESIAN_POINT('Ctrl Pts',(94.9304422236125,2.2001691206571,-0.150062634867785));
#10562=CARTESIAN_POINT('Ctrl Pts',(94.9345007030675,2.20400947702594,-0.0748903311412995));
#10563=CARTESIAN_POINT('Ctrl Pts',(94.9385591825226,2.20399998241828,0.000278388606040127));
#10564=CARTESIAN_POINT('Ctrl Pts',(94.942617709155,2.20399048770026,0.0754479821437415));
#10565=CARTESIAN_POINT('Ctrl Pts',(94.9466762357873,2.20013105500196,0.150613514159087));
#10566=CARTESIAN_POINT('Ctrl Pts',(94.9507347624197,2.1924488084373,0.225353549743164));
#10567=CARTESIAN_POINT('Ctrl Pts',(94.9547974394048,2.18475870581164,0.30017001639128));
#10568=CARTESIAN_POINT('Ctrl Pts',(94.9588601163899,2.17323803158467,0.374559641677874));
#10569=CARTESIAN_POINT('Ctrl Pts',(94.962922793375,2.15796572196852,0.448107066234035));
#10570=CARTESIAN_POINT('Ctrl Pts',(94.9669875923521,2.14268543541547,0.521692905619417));
#10571=CARTESIAN_POINT('Ctrl Pts',(94.9710523913291,2.12364973224626,0.594435205933648));
#10572=CARTESIAN_POINT('Ctrl Pts',(94.9751171903062,2.10098789089885,0.665932340629578));
#10573=CARTESIAN_POINT('Ctrl Pts',(94.9791892505482,2.07828556695056,0.737557196190026));
#10574=CARTESIAN_POINT('Ctrl Pts',(94.9832613107902,2.05194433384007,0.807931995367446));
#10575=CARTESIAN_POINT('Ctrl Pts',(94.9873333710322,2.022142046902,0.876674136809688));
#10576=CARTESIAN_POINT('Ctrl Pts',(94.9904715218311,1.99917478585852,0.929650564775497));
#10577=CARTESIAN_POINT('Ctrl Pts',(94.9936096726299,1.97415298327347,0.981657723094009));
#10578=CARTESIAN_POINT('Ctrl Pts',(94.9967478234288,1.9471761147697,1.0325314416861));
#10579=CARTESIAN_POINT('Ctrl Pts',(95.0008208883648,1.91216232982829,1.09856139774659));
#10580=CARTESIAN_POINT('Ctrl Pts',(95.0048939533008,1.87371854060252,1.16293566041432));
#10581=CARTESIAN_POINT('Ctrl Pts',(95.0089670182368,1.83202538915432,1.22527506034113));
#10582=CARTESIAN_POINT('Ctrl Pts',(95.0130340990418,1.79039349311968,1.28752287146761));
#10583=CARTESIAN_POINT('Ctrl Pts',(95.0171011798469,1.74552197633398,1.34774136186964));
#10584=CARTESIAN_POINT('Ctrl Pts',(95.0211682606519,1.6976374152314,1.40557575619618));
#10585=CARTESIAN_POINT('Ctrl Pts',(95.0252305830208,1.64980887849607,1.46334248496888));
#10586=CARTESIAN_POINT('Ctrl Pts',(95.0292929053897,1.59897460422833,1.51873029357842));
#10587=CARTESIAN_POINT('Ctrl Pts',(95.0333552277586,1.54540357443698,1.57141458314393));
#10588=CARTESIAN_POINT('Ctrl Pts',(95.0374149718979,1.4918665445108,1.62406543563069));
#10589=CARTESIAN_POINT('Ctrl Pts',(95.0414747160372,1.43559654537654,1.67401584003322));
#10590=CARTESIAN_POINT('Ctrl Pts',(95.0455344601765,1.37690091599836,1.72097642852041));
#10591=CARTESIAN_POINT('Ctrl Pts',(95.0495929396315,1.3182235713779,1.76792238792889));
#10592=CARTESIAN_POINT('Ctrl Pts',(95.0536514190866,1.25712246935887,1.81188008255283));
#10593=CARTESIAN_POINT('Ctrl Pts',(95.0577098985416,1.19393845136267,1.85260005785321));
#10594=CARTESIAN_POINT('Ctrl Pts',(95.061768425174,1.13075369889094,1.89332050649837));
#10595=CARTESIAN_POINT('Ctrl Pts',(95.0658269518064,1.06548638467391,1.93080290395108));
#10596=CARTESIAN_POINT('Ctrl Pts',(95.0698854784388,0.9985054187136,1.9648417057869));
#10597=CARTESIAN_POINT('Ctrl Pts',(95.0739481554239,0.931455956311528,1.99891531656843));
#10598=CARTESIAN_POINT('Ctrl Pts',(95.078010832409,0.862689769272217,2.02953808269096));
#10599=CARTESIAN_POINT('Ctrl Pts',(95.0820735093941,0.792598733999952,2.05655129935085));
#10600=CARTESIAN_POINT('Ctrl Pts',(95.0861383083712,0.722471089217977,2.08357862538455));
#10601=CARTESIAN_POINT('Ctrl Pts',(95.0902031073482,0.651017672324267,2.10699249871576));
#10602=CARTESIAN_POINT('Ctrl Pts',(95.0942679063253,0.57864609381734,2.12668396761483));
#10603=CARTESIAN_POINT('Ctrl Pts',(95.0983399665673,0.506145232359268,2.14641061290861));
#10604=CARTESIAN_POINT('Ctrl Pts',(95.1024120268093,0.432723400366107,2.16240146991543));
#10605=CARTESIAN_POINT('Ctrl Pts',(95.1064840870513,0.358798537729981,2.17459872374717));
#10606=CARTESIAN_POINT('Ctrl Pts',(95.1096222378502,0.301828023309634,2.18399859005102));
#10607=CARTESIAN_POINT('Ctrl Pts',(95.1127603886491,0.244558981630548,2.19114645589506));
#10608=CARTESIAN_POINT('Ctrl Pts',(95.1158985394479,0.187183294628014,2.19603697924516));
#10609=CARTESIAN_POINT('Ctrl Pts',(95.1192818285661,0.12532567530837,2.20130952842877));
#10610=CARTESIAN_POINT('Ctrl Pts',(95.1226651176843,0.0632421790914876,
2.2039689515483));
#10611=CARTESIAN_POINT('Ctrl Pts',(95.1260484068025,0.00109146181604489,
2.20399972974388));
#10612=CARTESIAN_POINT('',(95.8760484067755,0.00133902696002769,2.20399959324107));
#10613=CARTESIAN_POINT('Ctrl Pts',(95.1260484068548,0.00109146085464169,
2.20399972974436));
#10614=CARTESIAN_POINT('Ctrl Pts',(95.1300735385946,-0.072849847740999,
2.20403634682865));
#10615=CARTESIAN_POINT('Ctrl Pts',(95.1340986703343,-0.146942092471922,
2.20034777635078));
#10616=CARTESIAN_POINT('Ctrl Pts',(95.138123802074,-0.220773424115571,2.19291474873153));
#10617=CARTESIAN_POINT('Ctrl Pts',(95.1421623626321,-0.294851075035982,
2.18545692272457));
#10618=CARTESIAN_POINT('Ctrl Pts',(95.1462009231901,-0.368665574139318,
2.17422954668617));
#10619=CARTESIAN_POINT('Ctrl Pts',(95.1502394837482,-0.441799140599636,
2.15926596772269));
#10620=CARTESIAN_POINT('Ctrl Pts',(95.1542550801847,-0.514516853915588,
2.14438747487855));
#10621=CARTESIAN_POINT('Ctrl Pts',(95.1582706766213,-0.586560870724673,
2.12581523600944));
#10622=CARTESIAN_POINT('Ctrl Pts',(95.1622862730578,-0.657526071900074,
2.10363387136917));
#10623=CARTESIAN_POINT('Ctrl Pts',(95.1662998439655,-0.728455477133412,
2.08146369535136));
#10624=CARTESIAN_POINT('Ctrl Pts',(95.1703134148733,-0.798306679744222,
2.0556881501414));
#10625=CARTESIAN_POINT('Ctrl Pts',(95.1743269857811,-0.866687961998495,
2.02644219669027));
#10626=CARTESIAN_POINT('Ctrl Pts',(95.178339900323,-0.935058061409059,1.9972010260235));
#10627=CARTESIAN_POINT('Ctrl Pts',(95.1823528148649,-1.00195826810386,1.96449076691085));
#10628=CARTESIAN_POINT('Ctrl Pts',(95.1863657294069,-1.06701681521606,1.92849452061606));
#10629=CARTESIAN_POINT('Ctrl Pts',(95.1904226899119,-1.1327894483958,1.89210317761064));
#10630=CARTESIAN_POINT('Ctrl Pts',(95.1944796504169,-1.19667928584886,1.85235349304124));
#10631=CARTESIAN_POINT('Ctrl Pts',(95.1985366109219,-1.25832955190855,1.8094813452461));
#10632=CARTESIAN_POINT('Ctrl Pts',(95.202554691631,-1.31938899393611,1.76702006178043));
#10633=CARTESIAN_POINT('Ctrl Pts',(95.2065727723401,-1.37825125334203,1.72149626042148));
#10634=CARTESIAN_POINT('Ctrl Pts',(95.2105908530492,-1.43460238853593,1.6731802015345));
#10635=CARTESIAN_POINT('Ctrl Pts',(95.2146672534522,-1.49177142192389,1.62416286809161));
#10636=CARTESIAN_POINT('Ctrl Pts',(95.2187436538552,-1.54635547126111,1.57227192882445));
#10637=CARTESIAN_POINT('Ctrl Pts',(95.2228200542582,-1.59806652092165,1.51782719527269));
#10638=CARTESIAN_POINT('Ctrl Pts',(95.2268964546612,-1.6497775705822,1.46338246172093));
#10639=CARTESIAN_POINT('Ctrl Pts',(95.2309728550642,-1.698615337954,1.40638437361926));
#10640=CARTESIAN_POINT('Ctrl Pts',(95.2350492554671,-1.74433661151164,1.34718439188557));
#10641=CARTESIAN_POINT('Ctrl Pts',(95.2391223204031,-1.79002047417145,1.28803284984519));
#10642=CARTESIAN_POINT('Ctrl Pts',(95.2431953853391,-1.83278022606828,1.22644085164921));
#10643=CARTESIAN_POINT('Ctrl Pts',(95.2472684502751,-1.87234510209011,1.16272946925723));
#10644=CARTESIAN_POINT('Ctrl Pts',(95.2513355310802,-1.91185184955223,1.09911169137681));
#10645=CARTESIAN_POINT('Ctrl Pts',(95.2554026118852,-1.94817279064879,1.03338111369175));
#10646=CARTESIAN_POINT('Ctrl Pts',(95.2594696926903,-1.981078342687,0.965890573583024));
#10647=CARTESIAN_POINT('Ctrl Pts',(95.2635320150592,-2.0139453956205,0.89847899660389));
#10648=CARTESIAN_POINT('Ctrl Pts',(95.2675943374281,-2.04340479037228,0.829311975244283));
#10649=CARTESIAN_POINT('Ctrl Pts',(95.2716566597969,-2.0692719364077,0.758768510940943));
#10650=CARTESIAN_POINT('Ctrl Pts',(95.2757164039363,-2.09512266537068,0.688269818378645));
#10651=CARTESIAN_POINT('Ctrl Pts',(95.2797761480756,-2.11738550585129,0.616396863546591));
#10652=CARTESIAN_POINT('Ctrl Pts',(95.2838358922149,-2.1359237916369,0.543549037640074));
#10653=CARTESIAN_POINT('Ctrl Pts',(95.2878943716699,-2.15445630240879,0.470723905158345));
#10654=CARTESIAN_POINT('Ctrl Pts',(95.291952851125,-2.16926644447123,0.39692496697706));
#10655=CARTESIAN_POINT('Ctrl Pts',(95.29601133058,-2.18026773625882,0.322565649486823));
#10656=CARTESIAN_POINT('Ctrl Pts',(95.3000698572124,-2.19126915592969,0.248205467614994));
#10657=CARTESIAN_POINT('Ctrl Pts',(95.3041283838449,-2.19846156931004,0.173285366082212));
#10658=CARTESIAN_POINT('Ctrl Pts',(95.3081869104772,-2.20181007632792,0.0982262071996763));
#10659=CARTESIAN_POINT('Ctrl Pts',(95.3122495874623,-2.20516200761437,0.0230902909095669));
#10660=CARTESIAN_POINT('Ctrl Pts',(95.3163122644474,-2.20466216147588,-0.0521844886567871));
#10661=CARTESIAN_POINT('Ctrl Pts',(95.3203749414325,-2.20032778102013,-0.127175689780132));
#10662=CARTESIAN_POINT('Ctrl Pts',(95.3244397404096,-2.19599113665797,-0.202206059837059));
#10663=CARTESIAN_POINT('Ctrl Pts',(95.3285045393866,-2.18781602149744,-0.276952081418629));
#10664=CARTESIAN_POINT('Ctrl Pts',(95.3325693383637,-2.17587148944344,-0.350997523391801));
#10665=CARTESIAN_POINT('Ctrl Pts',(95.3366413986057,-2.16390561994752,-0.42517523846793));
#10666=CARTESIAN_POINT('Ctrl Pts',(95.3407134588477,-2.14815698392865,-0.49864940661286));
#10667=CARTESIAN_POINT('Ctrl Pts',(95.3447855190897,-2.12874547502596,-0.571015501152542));
#10668=CARTESIAN_POINT('Ctrl Pts',(95.3479236698886,-2.11378591191795,-0.626784744212076));
#10669=CARTESIAN_POINT('Ctrl Pts',(95.3510618206874,-2.09665198995791,-0.68189612088876));
#10670=CARTESIAN_POINT('Ctrl Pts',(95.3541999714863,-2.07741806422642,-0.736172660743221));
#10671=CARTESIAN_POINT('Ctrl Pts',(95.3582730364223,-2.05245399031801,-0.806619202511925));
#10672=CARTESIAN_POINT('Ctrl Pts',(95.3623461013583,-2.02385438390514,-0.875930335362855));
#10673=CARTESIAN_POINT('Ctrl Pts',(95.3664191662942,-1.99174239801431,-0.943704519408594));
#10674=CARTESIAN_POINT('Ctrl Pts',(95.3704862470993,-1.95967759092642,-1.01137912989062));
#10675=CARTESIAN_POINT('Ctrl Pts',(95.3745533279044,-1.92411085254978,-1.0775208468792));
#10676=CARTESIAN_POINT('Ctrl Pts',(95.3786204087094,-1.88521434804376,-1.14174553291439));
#10677=CARTESIAN_POINT('Ctrl Pts',(95.3826827310783,-1.8463633519856,-1.20589507683043));
#10678=CARTESIAN_POINT('Ctrl Pts',(95.3867450534472,-1.80419057593485,-1.26813163958155));
#10679=CARTESIAN_POINT('Ctrl Pts',(95.390807375816,-1.75891455346316,-1.32809472313367));
#10680=CARTESIAN_POINT('Ctrl Pts',(95.3948671199553,-1.71366726627367,-1.38801974998305));
#10681=CARTESIAN_POINT('Ctrl Pts',(95.3989268640946,-1.66532092797137,-1.44567378085091));
#10682=CARTESIAN_POINT('Ctrl Pts',(95.4029866082339,-1.61413717598334,-1.50072555022847));
#10683=CARTESIAN_POINT('Ctrl Pts',(95.407045087689,-1.56296936866645,-1.55576016997701));
#10684=CARTESIAN_POINT('Ctrl Pts',(95.411103567144,-1.50896622751712,-1.60819378830145));
#10685=CARTESIAN_POINT('Ctrl Pts',(95.4151620465991,-1.45242837753489,-1.65772971504144));
#10686=CARTESIAN_POINT('Ctrl Pts',(95.4192205732315,-1.39588987033482,-1.70726621760621));
#10687=CARTESIAN_POINT('Ctrl Pts',(95.4232790998638,-1.33681695610085,-1.75390464840955));
#10688=CARTESIAN_POINT('Ctrl Pts',(95.4273376264962,-1.27554445759278,-1.79738764230322));
#10689=CARTESIAN_POINT('Ctrl Pts',(95.4314003034813,-1.21420930026703,-1.84091510301403));
#10690=CARTESIAN_POINT('Ctrl Pts',(95.4354629804664,-1.15067045708161,-1.88128040607972));
#10691=CARTESIAN_POINT('Ctrl Pts',(95.4395256574515,-1.08529233052476,-1.91826915663682));
#10692=CARTESIAN_POINT('Ctrl Pts',(95.4435904564286,-1.01988005607513,-1.95527722692599));
#10693=CARTESIAN_POINT('Ctrl Pts',(95.4476552554056,-0.952627012595539,
-1.98890501889766));
#10694=CARTESIAN_POINT('Ctrl Pts',(95.4517200543827,-0.883920454766032,
-2.0189850493865));
#10695=CARTESIAN_POINT('Ctrl Pts',(95.4557921146247,-0.815091161095456,
-2.04911881416153));
#10696=CARTESIAN_POINT('Ctrl Pts',(95.4598641748667,-0.744803613989299,
-2.07569198941107));
#10697=CARTESIAN_POINT('Ctrl Pts',(95.4639362351087,-0.673462776609276,
-2.0985861641881));
#10698=CARTESIAN_POINT('Ctrl Pts',(95.4670743859076,-0.618483652404165,
-2.11622965878202));
#10699=CARTESIAN_POINT('Ctrl Pts',(95.4702125367064,-0.562879348821488,
-2.13168917184189));
#10700=CARTESIAN_POINT('Ctrl Pts',(95.4733506875053,-0.506838895599709,
-2.14493131216533));
#10701=CARTESIAN_POINT('Ctrl Pts',(95.4774237524413,-0.434102937500836,
-2.16211853511467));
#10702=CARTESIAN_POINT('Ctrl Pts',(95.4814968173773,-0.360351477878771,
-2.17563492618856));
#10703=CARTESIAN_POINT('Ctrl Pts',(95.4855698823133,-0.285988735521359,
-2.18536643223851));
#10704=CARTESIAN_POINT('Ctrl Pts',(95.4896369631183,-0.2117352466116,-2.19508364079818));
#10705=CARTESIAN_POINT('Ctrl Pts',(95.4937040439234,-0.136872727543854,
-2.20102694322759));
#10706=CARTESIAN_POINT('Ctrl Pts',(95.4977711247285,-0.0618173262461914,
-2.20313290978456));
#10707=CARTESIAN_POINT('Ctrl Pts',(95.5018334470973,0.0131502611242621,
-2.20523641238569));
#10708=CARTESIAN_POINT('Ctrl Pts',(95.5058957694662,0.0883098074955325,
-2.20351148567463));
#10709=CARTESIAN_POINT('Ctrl Pts',(95.5099580918351,0.163239910382419,-2.19794648061738));
#10710=CARTESIAN_POINT('Ctrl Pts',(95.5140178359744,0.238122457465352,-2.19238500749562));
#10711=CARTESIAN_POINT('Ctrl Pts',(95.5180775801137,0.31277537508975,-2.18298832761805));
#10712=CARTESIAN_POINT('Ctrl Pts',(95.522137324253,0.386778475984921,-2.16979685927388));
#10713=CARTESIAN_POINT('Ctrl Pts',(95.5261958037081,0.460758523566107,-2.1566095003124));
#10714=CARTESIAN_POINT('Ctrl Pts',(95.5302542831632,0.534088686589196,-2.13962978371868));
#10715=CARTESIAN_POINT('Ctrl Pts',(95.5343127626182,0.606356713896499,-2.11894963024434));
#10716=CARTESIAN_POINT('Ctrl Pts',(95.5383712892506,0.678625581275309,-2.0982692363759));
#10717=CARTESIAN_POINT('Ctrl Pts',(95.542429815883,0.749831829880887,-2.07388845329947));
#10718=CARTESIAN_POINT('Ctrl Pts',(95.5464883425154,0.819577731951936,-2.04594925188493));
#10719=CARTESIAN_POINT('Ctrl Pts',(95.5505510195005,0.8893949579589,-2.01798147913141));
#10720=CARTESIAN_POINT('Ctrl Pts',(95.5546136964856,0.957748411015381,-1.98644819924844));
#10721=CARTESIAN_POINT('Ctrl Pts',(95.5586763734707,1.02426045273147,-1.9515395268788));
#10722=CARTESIAN_POINT('Ctrl Pts',(95.5627411724478,1.09080723459977,-1.91661262123049));
#10723=CARTESIAN_POINT('Ctrl Pts',(95.5668059714248,1.15551027856716,-1.87830705568835));
#10724=CARTESIAN_POINT('Ctrl Pts',(95.5708707704018,1.21801899346771,-1.8368575697511));
#10725=CARTESIAN_POINT('Ctrl Pts',(95.5749428306438,1.28063937252291,-1.79533403938956));
#10726=CARTESIAN_POINT('Ctrl Pts',(95.5790148908859,1.34105720834959,-1.75065565496199));
#10727=CARTESIAN_POINT('Ctrl Pts',(95.5830869511279,1.39895355987823,-1.70309862817866));
#10728=CARTESIAN_POINT('Ctrl Pts',(95.5862251019268,1.44357163304115,-1.66644860025108));
#10729=CARTESIAN_POINT('Ctrl Pts',(95.5893632527256,1.48669281739357,-1.62808978664815));
#10730=CARTESIAN_POINT('Ctrl Pts',(95.5925014035245,1.52818662763047,-1.58816297373141));
#10731=CARTESIAN_POINT('Ctrl Pts',(95.5965744684605,1.58204222424386,-1.53634121240784));
#10732=CARTESIAN_POINT('Ctrl Pts',(95.6006475333965,1.63336272749686,-1.48167699586817));
#10733=CARTESIAN_POINT('Ctrl Pts',(95.6047205983325,1.68183326234142,-1.42444827132543));
#10734=CARTESIAN_POINT('Ctrl Pts',(95.6087876791376,1.73023258446756,-1.36730362699884));
#10735=CARTESIAN_POINT('Ctrl Pts',(95.6128547599426,1.77578994538915,-1.30760231653738));
#10736=CARTESIAN_POINT('Ctrl Pts',(95.6169218407477,1.81822655528487,-1.24565974232811));
#10737=CARTESIAN_POINT('Ctrl Pts',(95.6209841631166,1.86061351485146,-1.18378964019433));
#10738=CARTESIAN_POINT('Ctrl Pts',(95.6250464854854,1.89988670908004,-1.11968387603866));
#10739=CARTESIAN_POINT('Ctrl Pts',(95.6291088078543,1.93580802250771,-1.05369032452367));
#10740=CARTESIAN_POINT('Ctrl Pts',(95.6331685519936,1.97170653779581,-0.987738657061754));
#10741=CARTESIAN_POINT('Ctrl Pts',(95.6372282961329,2.00425716606191,-0.919901998078399));
#10742=CARTESIAN_POINT('Ctrl Pts',(95.6412880402722,2.03326621255493,-0.850555412000014));
#10743=CARTESIAN_POINT('Ctrl Pts',(95.6453465197272,2.06226622220153,-0.781230428646454));
#10744=CARTESIAN_POINT('Ctrl Pts',(95.6494049991823,2.08772665642617,-0.71039689228359));
#10745=CARTESIAN_POINT('Ctrl Pts',(95.6534634786373,2.10950140794812,-0.638451102172221));
#10746=CARTESIAN_POINT('Ctrl Pts',(95.6575220052697,2.13127641258827,-0.566504475734888));
#10747=CARTESIAN_POINT('Ctrl Pts',(95.6615805319021,2.14936551286382,-0.493446027386033));
#10748=CARTESIAN_POINT('Ctrl Pts',(95.6656390585345,2.16367253740287,-0.419686967737422));
#10749=CARTESIAN_POINT('Ctrl Pts',(95.6697017355196,2.17799419266959,-0.345852480195889));
#10750=CARTESIAN_POINT('Ctrl Pts',(95.6737644125047,2.18852595760925,-0.271316420384699));
#10751=CARTESIAN_POINT('Ctrl Pts',(95.6778270894898,2.19522301024608,-0.19649919919978));
#10752=CARTESIAN_POINT('Ctrl Pts',(95.6818918884669,2.20192356084541,-0.12164289995342));
#10753=CARTESIAN_POINT('Ctrl Pts',(95.6859566874439,2.20478539232686,-0.0465056244456972));
#10754=CARTESIAN_POINT('Ctrl Pts',(95.6900214864209,2.20381584438883,0.0284907707995336));
#10755=CARTESIAN_POINT('Ctrl Pts',(95.6940935466629,2.20284456447229,0.103621137909155));
#10756=CARTESIAN_POINT('Ctrl Pts',(95.698165606905,2.19802826484776,0.178609644888324));
#10757=CARTESIAN_POINT('Ctrl Pts',(95.702237667147,2.18942629103923,0.253038566440345));
#10758=CARTESIAN_POINT('Ctrl Pts',(95.7053758179458,2.18279714280103,0.310397536039677));
#10759=CARTESIAN_POINT('Ctrl Pts',(95.7085139687447,2.17392072501234,0.367424234420507));
#10760=CARTESIAN_POINT('Ctrl Pts',(95.7116521195436,2.16284466817774,0.423932708498817));
#10761=CARTESIAN_POINT('Ctrl Pts',(95.7157251844796,2.14846884572262,0.497276119668516));
#10762=CARTESIAN_POINT('Ctrl Pts',(95.7197982494156,2.13033039049547,0.570028900137833));
#10763=CARTESIAN_POINT('Ctrl Pts',(95.7238713143516,2.1084923097542,0.641775801746541));
#10764=CARTESIAN_POINT('Ctrl Pts',(95.7279383951566,2.08668631343496,0.713417293090574));
#10765=CARTESIAN_POINT('Ctrl Pts',(95.7320054759617,2.06119162111387,0.784055386697324));
#10766=CARTESIAN_POINT('Ctrl Pts',(95.7360725567667,2.03212227262231,0.853284869848483));
#10767=CARTESIAN_POINT('Ctrl Pts',(95.7401348791356,2.0030869349229,0.922433355327382));
#10768=CARTESIAN_POINT('Ctrl Pts',(95.7441972015045,1.97048543426028,0.990176066650771));
#10769=CARTESIAN_POINT('Ctrl Pts',(95.7482595238733,1.93448114142777,1.05612438351755));
#10770=CARTESIAN_POINT('Ctrl Pts',(95.7523192680126,1.89849969939927,1.12203084504027));
#10771=CARTESIAN_POINT('Ctrl Pts',(95.7563790121519,1.85911997899782,1.18614475401206));
#10772=CARTESIAN_POINT('Ctrl Pts',(95.7604387562913,1.81655227190928,1.24810009351063));
#10773=CARTESIAN_POINT('Ctrl Pts',(95.7644972357463,1.77399782543693,1.31003613279234));
#10774=CARTESIAN_POINT('Ctrl Pts',(95.7685557152014,1.72825763427084,1.36981454441949));
#10775=CARTESIAN_POINT('Ctrl Pts',(95.7726141946564,1.67958562172051,1.4270978029938));
#10776=CARTESIAN_POINT('Ctrl Pts',(95.7766727212888,1.63091304338781,1.48438172745096));
#10777=CARTESIAN_POINT('Ctrl Pts',(95.7807312479212,1.57930888652639,1.53917007857161));
#10778=CARTESIAN_POINT('Ctrl Pts',(95.7847897745536,1.52506666365048,1.59115922252363));
#10779=CARTESIAN_POINT('Ctrl Pts',(95.7888524515387,1.47076897129588,1.64320153189843));
#10780=CARTESIAN_POINT('Ctrl Pts',(95.7929151285238,1.41382817113154,1.6924385866597));
#10781=CARTESIAN_POINT('Ctrl Pts',(95.7969778055089,1.35457333061416,1.73860492694253));
#10782=CARTESIAN_POINT('Ctrl Pts',(95.8010426044859,1.29528754048039,1.78479538053847));
#10783=CARTESIAN_POINT('Ctrl Pts',(95.805107403463,1.2336856946048,1.82791165165345));
#10784=CARTESIAN_POINT('Ctrl Pts',(95.80917220244,1.17012633775186,1.86773133873676));
#10785=CARTESIAN_POINT('Ctrl Pts',(95.813244262682,1.1064534399011,1.90762215880864));
#10786=CARTESIAN_POINT('Ctrl Pts',(95.8173163229241,1.04081646405801,1.94420439935276));
#10787=CARTESIAN_POINT('Ctrl Pts',(95.8213883831661,0.973598660538437,1.97730160779729));
#10788=CARTESIAN_POINT('Ctrl Pts',(95.824526533965,0.921796970170994,2.00280811431936));
#10789=CARTESIAN_POINT('Ctrl Pts',(95.8276646847639,0.869056935062801,2.0262457724316));
#10790=CARTESIAN_POINT('Ctrl Pts',(95.8308028355628,0.815560654889221,2.04755386209903));
#10791=CARTESIAN_POINT('Ctrl Pts',(95.8353960033341,0.737260596757818,2.07874153821811));
#10792=CARTESIAN_POINT('Ctrl Pts',(95.8399891711054,0.657087046343997,2.10546688559112));
#10793=CARTESIAN_POINT('Ctrl Pts',(95.8445823388767,0.575530641081532,2.12752919631583));
#10794=CARTESIAN_POINT('Ctrl Pts',(95.8491582578205,0.494280506444697,2.14950865594274));
#10795=CARTESIAN_POINT('Ctrl Pts',(95.8537341767643,0.411658102933076,2.16685989473513));
#10796=CARTESIAN_POINT('Ctrl Pts',(95.8583100957081,0.328170611828205,2.17943112979794));
#10797=CARTESIAN_POINT('Ctrl Pts',(95.8628571209176,0.245210285958407,2.19192298628559));
#10798=CARTESIAN_POINT('Ctrl Pts',(95.8674041461271,0.161395999516733,2.19969489573444));
#10799=CARTESIAN_POINT('Ctrl Pts',(95.8719511713365,0.077243792355056,2.20264599891644));
#10800=CARTESIAN_POINT('Ctrl Pts',(95.8733169164828,0.0519678233012755,
2.20353239269289));
#10801=CARTESIAN_POINT('Ctrl Pts',(95.8746826616292,0.0266614814832344,
2.2039842087331));
#10802=CARTESIAN_POINT('Ctrl Pts',(95.8760484067755,0.00133902696002845,
2.20399959324107));
#10803=CARTESIAN_POINT('',(96.6260484068518,-0.0017560042200646,2.20399930046477));
#10804=CARTESIAN_POINT('Ctrl Pts',(95.8760484068025,0.00133902645877407,
2.20399959324137));
#10805=CARTESIAN_POINT('Ctrl Pts',(95.8801415572499,-0.0745525967635283,
2.20404570073241));
#10806=CARTESIAN_POINT('Ctrl Pts',(95.8842347076972,-0.150456680726987,
2.20016763868404));
#10807=CARTESIAN_POINT('Ctrl Pts',(95.8883278581446,-0.225943957588798,
2.19238804230207));
#10808=CARTESIAN_POINT('Ctrl Pts',(95.8924217124816,-0.301444215823037,
2.18460710808091));
#10809=CARTESIAN_POINT('Ctrl Pts',(95.8965155668186,-0.376527061147336,
2.17292335529049));
#10810=CARTESIAN_POINT('Ctrl Pts',(95.9006094211556,-0.450769289729901,
2.15741119108908));
#10811=CARTESIAN_POINT('Ctrl Pts',(95.9047214320244,-0.525340787817131,
2.14183022934858));
#10812=CARTESIAN_POINT('Ctrl Pts',(95.9088334428933,-0.599063731269043,
2.12238691207033));
#10813=CARTESIAN_POINT('Ctrl Pts',(95.9129454537622,-0.671522599166809,
2.0992078026742));
#10814=CARTESIAN_POINT('Ctrl Pts',(95.9170471156906,-0.743799105555967,
2.07608702951048));
#10815=CARTESIAN_POINT('Ctrl Pts',(95.9211487776191,-0.814817469942279,
2.04924945607877));
#10816=CARTESIAN_POINT('Ctrl Pts',(95.9252504395475,-0.884185175174658,
2.01886913295572));
#10817=CARTESIAN_POINT('Ctrl Pts',(95.9293676248866,-0.953815413836089,
1.98837383052956));
#10818=CARTESIAN_POINT('Ctrl Pts',(95.9334848102257,-1.02178205961179,1.95430913518859));
#10819=CARTESIAN_POINT('Ctrl Pts',(95.9376019955647,-1.08771450162772,1.91689675333565));
#10820=CARTESIAN_POINT('Ctrl Pts',(95.9417191809038,-1.15364694364365,1.87948437148271));
#10821=CARTESIAN_POINT('Ctrl Pts',(95.9458363662428,-1.21754482386606,1.83872461058378));
#10822=CARTESIAN_POINT('Ctrl Pts',(95.9499535515819,-1.27906965800229,1.79488072305039));
#10823=CARTESIAN_POINT('Ctrl Pts',(95.9540266165179,-1.33993518237773,1.75150667348419));
#10824=CARTESIAN_POINT('Ctrl Pts',(95.9580996814539,-1.398709319395,1.70494948884079));
#10825=CARTESIAN_POINT('Ctrl Pts',(95.9621727463899,-1.45503987674905,1.65543799553777));
#10826=CARTESIAN_POINT('Ctrl Pts',(95.9662398271949,-1.51128767347052,1.60599924432533));
#10827=CARTESIAN_POINT('Ctrl Pts',(95.970306908,-1.56509866269076,1.55361511462868));
#10828=CARTESIAN_POINT('Ctrl Pts',(95.9743739888051,-1.61615086168616,1.49855676978588));
#10829=CARTESIAN_POINT('Ctrl Pts',(95.9784363111739,-1.66714333021566,1.44356284255199));
#10830=CARTESIAN_POINT('Ctrl Pts',(95.9824986335428,-1.71538309831979,1.38590126473668));
#10831=CARTESIAN_POINT('Ctrl Pts',(95.9865609559117,-1.76058366238125,1.32588127966128));
#10832=CARTESIAN_POINT('Ctrl Pts',(95.990620700051,-1.80575553905165,1.26589938740218));
#10833=CARTESIAN_POINT('Ctrl Pts',(95.9946804441903,-1.84789175284692,1.20356243857123));
#10834=CARTESIAN_POINT('Ctrl Pts',(95.9987401883296,-1.88674575898031,1.1392130797045));
#10835=CARTESIAN_POINT('Ctrl Pts',(96.0027986677846,-1.925587661383,1.0748837668353));
#10836=CARTESIAN_POINT('Ctrl Pts',(96.0068571472397,-1.96114913955829,1.00854369708425));
#10837=CARTESIAN_POINT('Ctrl Pts',(96.0109156266947,-1.99322761242658,0.940563493369933));
#10838=CARTESIAN_POINT('Ctrl Pts',(96.0149741533271,-2.02530645818755,0.872582499427198));
#10839=CARTESIAN_POINT('Ctrl Pts',(96.0190326799595,-2.05390201611521,0.802961766231307));
#10840=CARTESIAN_POINT('Ctrl Pts',(96.0230912065919,-2.07885891820595,0.732093981805324));
#10841=CARTESIAN_POINT('Ctrl Pts',(96.027153883577,-2.10384134186037,0.661153726178143));
#10842=CARTESIAN_POINT('Ctrl Pts',(96.0312165605621,-2.1251775201404,0.588964324038188));
#10843=CARTESIAN_POINT('Ctrl Pts',(96.0352792375472,-2.14276153291415,0.515935086094572));
#10844=CARTESIAN_POINT('Ctrl Pts',(96.0393440365243,-2.1603547300591,0.442867703977705));
#10845=CARTESIAN_POINT('Ctrl Pts',(96.0434088355013,-2.17419177098629,0.368960082256197));
#10846=CARTESIAN_POINT('Ctrl Pts',(96.0474736344784,-2.18421812285109,0.294630602295251));
#10847=CARTESIAN_POINT('Ctrl Pts',(96.0515456947204,-2.19426238556412,0.220168341832275));
#10848=CARTESIAN_POINT('Ctrl Pts',(96.0556177549624,-2.20048232252395,0.145283194404663));
#10849=CARTESIAN_POINT('Ctrl Pts',(96.0596898152044,-2.20287545090114,0.0703970725036641));
#10850=CARTESIAN_POINT('Ctrl Pts',(96.0628279660033,-2.20471972561281,0.0126857594823805));
#10851=CARTESIAN_POINT('Ctrl Pts',(96.0659661168022,-2.20429229956221,-0.0450260454446914));
#10852=CARTESIAN_POINT('Ctrl Pts',(96.069104267601,-2.2016130511633,-0.102547418043673));
#10853=CARTESIAN_POINT('Ctrl Pts',(96.073177332537,-2.19813560428206,-0.177205489251421));
#10854=CARTESIAN_POINT('Ctrl Pts',(96.077250397473,-2.19084959419916,-0.251830449426423));
#10855=CARTESIAN_POINT('Ctrl Pts',(96.081323462409,-2.17975652317247,-0.326002300125415));
#10856=CARTESIAN_POINT('Ctrl Pts',(96.0853905432141,-2.16867975004198,-0.400065177833923));
#10857=CARTESIAN_POINT('Ctrl Pts',(96.0894576240191,-2.15380709102484,-0.473675799477012));
#10858=CARTESIAN_POINT('Ctrl Pts',(96.0935247048242,-2.13519200048681,-0.546416618577013));
#10859=CARTESIAN_POINT('Ctrl Pts',(96.097587027193,-2.11659868938336,-0.61907233178359));
#10860=CARTESIAN_POINT('Ctrl Pts',(96.1016493495619,-2.09427176381602,-0.69085980407235));
#10861=CARTESIAN_POINT('Ctrl Pts',(96.1057116719308,-2.06831590746407,-0.761370676432365));
#10862=CARTESIAN_POINT('Ctrl Pts',(96.1097714160701,-2.04237652448626,-0.831836797736386));
#10863=CARTESIAN_POINT('Ctrl Pts',(96.1138311602094,-2.0128129456352,-0.901027479970799));
#10864=CARTESIAN_POINT('Ctrl Pts',(96.1178909043487,-1.97977958031341,-0.968549850742891));
#10865=CARTESIAN_POINT('Ctrl Pts',(96.1219493838038,-1.94675650548668,-1.03605118706644));
#10866=CARTESIAN_POINT('Ctrl Pts',(96.1260078632588,-1.91026599995695,-1.10188481518128));
#10867=CARTESIAN_POINT('Ctrl Pts',(96.1300663427139,-1.87050980755325,-1.16567965575757));
#10868=CARTESIAN_POINT('Ctrl Pts',(96.1341248693463,-1.8307531530082,-1.22947523790977));
#10869=CARTESIAN_POINT('Ctrl Pts',(96.1381833959787,-1.78773099026223,-1.29123158119967));
#10870=CARTESIAN_POINT('Ctrl Pts',(96.142241922611,-1.74168918975071,-1.35060533328783));
#10871=CARTESIAN_POINT('Ctrl Pts',(96.1463045995961,-1.69560030572121,-1.41003980248724));
#10872=CARTESIAN_POINT('Ctrl Pts',(96.1503672765812,-1.64648591068597,-1.46708643678975));
#10873=CARTESIAN_POINT('Ctrl Pts',(96.1544299535663,-1.59463263822371,-1.5214344379932));
#10874=CARTESIAN_POINT('Ctrl Pts',(96.1584947525434,-1.54275228208562,-1.57581082590354));
#10875=CARTESIAN_POINT('Ctrl Pts',(96.1625595515204,-1.48813054687872,-1.62748544533259));
#10876=CARTESIAN_POINT('Ctrl Pts',(96.1666243504975,-1.43108953270281,-1.67618577412782));
#10877=CARTESIAN_POINT('Ctrl Pts',(96.1706964107395,-1.37394662174913,-1.72497310008906));
#10878=CARTESIAN_POINT('Ctrl Pts',(96.1747684709815,-1.31437617854984,-1.77077523124125));
#10879=CARTESIAN_POINT('Ctrl Pts',(96.1788405312235,-1.25273147286246,-1.81336147993164));
#10880=CARTESIAN_POINT('Ctrl Pts',(96.1819786820224,-1.20522471439048,-1.84618075627017));
#10881=CARTESIAN_POINT('Ctrl Pts',(96.1851168328213,-1.15648668836683,-1.87709094779876));
#10882=CARTESIAN_POINT('Ctrl Pts',(96.1882549836202,-1.10668863603713,-1.90600531553988));
#10883=CARTESIAN_POINT('Ctrl Pts',(96.1923280485562,-1.04205480744733,-1.94353381717664));
#10884=CARTESIAN_POINT('Ctrl Pts',(96.1964011134922,-0.975385250761897,
-1.97784330326168));
#10885=CARTESIAN_POINT('Ctrl Pts',(96.2004741784282,-0.907033786194218,
-2.00870747265553));
#10886=CARTESIAN_POINT('Ctrl Pts',(96.2045412592333,-0.838782743328431,
-2.03952629653357));
#10887=CARTESIAN_POINT('Ctrl Pts',(96.2086083400383,-0.768855130169087,
-2.06690965868656));
#10888=CARTESIAN_POINT('Ctrl Pts',(96.2126754208434,-0.697630854785237,
-2.09067625194616));
#10889=CARTESIAN_POINT('Ctrl Pts',(96.2167377432123,-0.626489910957011,
-2.11441503857412));
#10890=CARTESIAN_POINT('Ctrl Pts',(96.2208000655811,-0.554055769629776,
-2.13454531311469));
#10891=CARTESIAN_POINT('Ctrl Pts',(96.22486238795,-0.480728373953735,-2.15093380429891));
#10892=CARTESIAN_POINT('Ctrl Pts',(96.2289221320893,-0.407447516893365,
-2.16731189421789));
#10893=CARTESIAN_POINT('Ctrl Pts',(96.2329818762286,-0.333274995260967,
-2.1799528094234));
#10894=CARTESIAN_POINT('Ctrl Pts',(96.2370416203679,-0.258624678211475,
-2.18877346379657));
#10895=CARTESIAN_POINT('Ctrl Pts',(96.241100099823,-0.183997616095518,-2.19759137037522));
#10896=CARTESIAN_POINT('Ctrl Pts',(96.245158579278,-0.108893527934604,-2.20259132298585));
#10897=CARTESIAN_POINT('Ctrl Pts',(96.2492170587331,-0.0337336127045116,
-2.20374182774977));
#10898=CARTESIAN_POINT('Ctrl Pts',(96.2532755853654,0.0414271762135432,
-2.2048923458876));
#10899=CARTESIAN_POINT('Ctrl Pts',(96.2573341119978,0.116643316057064,-2.20219332181591));
#10900=CARTESIAN_POINT('Ctrl Pts',(96.2613926386302,0.191493003523942,-2.19566537286568));
#10901=CARTESIAN_POINT('Ctrl Pts',(96.2654553156153,0.266419234187636,-2.18913074826858));
#10902=CARTESIAN_POINT('Ctrl Pts',(96.2695179926004,0.340977787421396,-2.17875942122692));
#10903=CARTESIAN_POINT('Ctrl Pts',(96.2735806695855,0.414752135179091,-2.16462390875745));
#10904=CARTESIAN_POINT('Ctrl Pts',(96.2776454685626,0.48856501629114,-2.15048101311582));
#10905=CARTESIAN_POINT('Ctrl Pts',(96.2817102675396,0.561592412097398,-2.13257013061648));
#10906=CARTESIAN_POINT('Ctrl Pts',(96.2857750665166,0.633430748860622,-2.11101432643122));
#10907=CARTESIAN_POINT('Ctrl Pts',(96.2898471267586,0.705397416004021,-2.08942001544485));
#10908=CARTESIAN_POINT('Ctrl Pts',(96.2939191870007,0.776170331002954,-2.06416793783538));
#10909=CARTESIAN_POINT('Ctrl Pts',(96.2979912472427,0.84536419341451,-2.03543002348217));
#10910=CARTESIAN_POINT('Ctrl Pts',(96.3011293980416,0.898688742094799,-2.01328302576462));
#10911=CARTESIAN_POINT('Ctrl Pts',(96.3042675488404,0.951075842084046,-1.9890667734598));
#10912=CARTESIAN_POINT('Ctrl Pts',(96.3074056996393,1.00235980775178,-1.96287819688432));
#10913=CARTESIAN_POINT('Ctrl Pts',(96.3114787645753,1.06892223120658,-1.92888755086076));
#10914=CARTESIAN_POINT('Ctrl Pts',(96.3155518295113,1.1338820900052,-1.89144175845474));
#10915=CARTESIAN_POINT('Ctrl Pts',(96.3196248944473,1.19685747229546,-1.85071558890353));
#10916=CARTESIAN_POINT('Ctrl Pts',(96.3236919752523,1.25974033140259,-1.81004925407989));
#10917=CARTESIAN_POINT('Ctrl Pts',(96.3277590560574,1.32064410502822,-1.76611236794642));
#10918=CARTESIAN_POINT('Ctrl Pts',(96.3318261368624,1.37921056355657,-1.7191260050892));
#10919=CARTESIAN_POINT('Ctrl Pts',(96.3358884592313,1.4377085000247,-1.67219461571794));
#10920=CARTESIAN_POINT('Ctrl Pts',(96.3399507816002,1.49387418393377,-1.62222113541162));
#10921=CARTESIAN_POINT('Ctrl Pts',(96.3440131039691,1.54737890414502,-1.56946950496242));
#10922=CARTESIAN_POINT('Ctrl Pts',(96.3480728481084,1.60084966657576,-1.51675135433109));
#10923=CARTESIAN_POINT('Ctrl Pts',(96.3521325922477,1.65166247747263,-1.46125888681238));
#10924=CARTESIAN_POINT('Ctrl Pts',(96.356192336387,1.69952326062962,-1.40329493926931));
#10925=CARTESIAN_POINT('Ctrl Pts',(96.3602508158421,1.74736913428081,-1.3453490485518));
#10926=CARTESIAN_POINT('Ctrl Pts',(96.3643092952971,1.79226450223659,-1.28493357436921));
#10927=CARTESIAN_POINT('Ctrl Pts',(96.3683677747522,1.83395467982266,-1.22238546799141));
#10928=CARTESIAN_POINT('Ctrl Pts',(96.3724263013846,1.87564534203156,-1.15983663453009));
#10929=CARTESIAN_POINT('Ctrl Pts',(96.376484828017,1.9141304765749,-1.09515551794187));
#10930=CARTESIAN_POINT('Ctrl Pts',(96.3805433546494,1.94919887051189,-1.02870781235255));
#10931=CARTESIAN_POINT('Ctrl Pts',(96.3846060316345,1.98430312628168,-0.962192155647132));
#10932=CARTESIAN_POINT('Ctrl Pts',(96.3886687086196,2.01598344068688,-0.893906725545878));
#10933=CARTESIAN_POINT('Ctrl Pts',(96.3927313856047,2.04407508041402,-0.824240902667667));
#10934=CARTESIAN_POINT('Ctrl Pts',(96.3967961845817,2.07218139279014,-0.75453869237403));
#10935=CARTESIAN_POINT('Ctrl Pts',(96.4008609835588,2.09669514197037,-0.683455105300154));
#10936=CARTESIAN_POINT('Ctrl Pts',(96.4049257825358,2.11750109898325,-0.611396022071397));
#10937=CARTESIAN_POINT('Ctrl Pts',(96.4089978427778,2.13834422328721,-0.539208214125991));
#10938=CARTESIAN_POINT('Ctrl Pts',(96.4130699030198,2.15546621650982,-0.466041894899636));
#10939=CARTESIAN_POINT('Ctrl Pts',(96.4171419632619,2.16880282102937,-0.392314062321301));
#10940=CARTESIAN_POINT('Ctrl Pts',(96.4202801140607,2.1790807328577,-0.335495389965608));
#10941=CARTESIAN_POINT('Ctrl Pts',(96.4234182648596,2.18711151924388,-0.278343473191536));
#10942=CARTESIAN_POINT('Ctrl Pts',(96.4265564156584,2.19288687768179,-0.221050088647333));
#10943=CARTESIAN_POINT('Ctrl Pts',(96.4306294805944,2.20038282400623,-0.146687927422888));
#10944=CARTESIAN_POINT('Ctrl Pts',(96.4347025455304,2.20410643737698,-0.0718006432719025));
#10945=CARTESIAN_POINT('Ctrl Pts',(96.4387756104664,2.20399768264422,0.00319607554513029));
#10946=CARTESIAN_POINT('Ctrl Pts',(96.4428426912715,2.20388908769349,0.0780826094788758));
#10947=CARTESIAN_POINT('Ctrl Pts',(96.4469097720766,2.19995930416598,0.153077785366209));
#10948=CARTESIAN_POINT('Ctrl Pts',(96.4509768528816,2.19220004781124,0.227760730540615));
#10949=CARTESIAN_POINT('Ctrl Pts',(96.4550391752505,2.18444986969419,0.302356297557017));
#10950=CARTESIAN_POINT('Ctrl Pts',(96.4591014976194,2.17287916944965,0.376639887122612));
#10951=CARTESIAN_POINT('Ctrl Pts',(96.4631638199882,2.15753168534196,0.450192210889408));
#10952=CARTESIAN_POINT('Ctrl Pts',(96.4672235641276,2.14219394180472,0.523697853285732));
#10953=CARTESIAN_POINT('Ctrl Pts',(96.4712833082668,2.12308426828563,0.596472684653092));
#10954=CARTESIAN_POINT('Ctrl Pts',(96.4753430524062,2.10029786088887,0.668105452414248));
#10955=CARTESIAN_POINT('Ctrl Pts',(96.4794015318612,2.07751855187313,0.739715905263258));
#10956=CARTESIAN_POINT('Ctrl Pts',(96.4834600113163,2.05106492770177,0.810184546180891));
#10957=CARTESIAN_POINT('Ctrl Pts',(96.4875184907713,2.02108220058087,0.879114747058197));
#10958=CARTESIAN_POINT('Ctrl Pts',(96.4915770174037,1.99109912492907,0.948045749207003));
#10959=CARTESIAN_POINT('Ctrl Pts',(96.4956355440361,1.95758705696382,1.0154378386879));
#10960=CARTESIAN_POINT('Ctrl Pts',(96.4996940706685,1.92073892097277,1.08091535166282));
#10961=CARTESIAN_POINT('Ctrl Pts',(96.5037567476536,1.88385310313939,1.14645982361014));
#10962=CARTESIAN_POINT('Ctrl Pts',(96.5078194246387,1.84362463929627,1.21008539222633));
#10963=CARTESIAN_POINT('Ctrl Pts',(96.5118821016238,1.80029154570757,1.27144262570273));
#10964=CARTESIAN_POINT('Ctrl Pts',(96.5159469006008,1.75693581864943,1.33283190690418));
#10965=CARTESIAN_POINT('Ctrl Pts',(96.5200116995779,1.71047252791787,1.39195011784231));
#10966=CARTESIAN_POINT('Ctrl Pts',(96.5240764985549,1.66118038040572,1.44848049477897));
#10967=CARTESIAN_POINT('Ctrl Pts',(96.5281485587969,1.61180017851593,1.50511185630261));
#10968=CARTESIAN_POINT('Ctrl Pts',(96.532220619039,1.55958135835212,1.55914580620202));
#10969=CARTESIAN_POINT('Ctrl Pts',(96.536292679281,1.50483958816004,1.61030239828));
#10970=CARTESIAN_POINT('Ctrl Pts',(96.5394308300799,1.46265260671785,1.64972644673636));
#10971=CARTESIAN_POINT('Ctrl Pts',(96.5425689808787,1.41896799657714,1.68744235793924));
#10972=CARTESIAN_POINT('Ctrl Pts',(96.5457071316776,1.37394244643187,1.72333924515541));
#10973=CARTESIAN_POINT('Ctrl Pts',(96.549771968387,1.31562099509928,1.76983636854456));
#10974=CARTESIAN_POINT('Ctrl Pts',(96.5538368050965,1.25481867372989,1.8134635003033));
#10975=CARTESIAN_POINT('Ctrl Pts',(96.5579016418059,1.19184989068572,1.85394439994096));
#10976=CARTESIAN_POINT('Ctrl Pts',(96.5619606890479,1.12897079284792,1.89436764342484));
#10977=CARTESIAN_POINT('Ctrl Pts',(96.5660197362898,1.06393175466375,1.93165328948619));
#10978=CARTESIAN_POINT('Ctrl Pts',(96.5700787835318,0.997079888480288,1.96556549012953));
#10979=CARTESIAN_POINT('Ctrl Pts',(96.574133372363,0.930301451617452,1.99944044200188));
#10980=CARTESIAN_POINT('Ctrl Pts',(96.5781879611942,0.861714563893496,2.02994908790959));
#10981=CARTESIAN_POINT('Ctrl Pts',(96.5822425500254,0.791693557190234,2.05689992744019));
#10982=CARTESIAN_POINT('Ctrl Pts',(96.5862942938241,0.721721682975405,2.08383185604858));
#10983=CARTESIAN_POINT('Ctrl Pts',(96.5903460376228,0.650318132728327,2.10721076118897));
#10984=CARTESIAN_POINT('Ctrl Pts',(96.5943977814215,0.577878578333352,2.12689265095901));
#10985=CARTESIAN_POINT('Ctrl Pts',(96.5984478135306,0.505469626571626,2.14656622596704));
#10986=CARTESIAN_POINT('Ctrl Pts',(96.6024978456397,0.432026002467835,2.16254576459369));
#10987=CARTESIAN_POINT('Ctrl Pts',(96.6065478777489,0.357958330807542,2.17473718720343));
#10988=CARTESIAN_POINT('Ctrl Pts',(96.6105987786785,0.283874770010601,2.18693122514015));
#10989=CARTESIAN_POINT('Ctrl Pts',(96.6146496796082,0.209167366512248,2.19533544172223));
#10990=CARTESIAN_POINT('Ctrl Pts',(96.6187005805378,0.134255495671819,2.1999071484683));
#10991=CARTESIAN_POINT('Ctrl Pts',(96.6211498559594,0.0889619159919616,
2.20267131603551));
#10992=CARTESIAN_POINT('Ctrl Pts',(96.623599131381,0.043593721674534,2.20403543217708));
#10993=CARTESIAN_POINT('Ctrl Pts',(96.6260484068025,-0.00175600330752527,
2.20399930046549));
#10994=CARTESIAN_POINT('',(97.3760484067751,-0.000421831323932275,2.20399995963211));
#10995=CARTESIAN_POINT('Ctrl Pts',(96.6260484068518,-0.00175600422006416,
2.20399930046477));
#10996=CARTESIAN_POINT('Ctrl Pts',(96.6308098313547,-0.0899164821416865,
2.20392905989289));
#10997=CARTESIAN_POINT('Ctrl Pts',(96.6355712558577,-0.177854000831902,
2.19856523823089));
#10998=CARTESIAN_POINT('Ctrl Pts',(96.6403326803606,-0.264996210083368,
2.18801119938666));
#10999=CARTESIAN_POINT('Ctrl Pts',(96.6451473637233,-0.353113147528027,
2.17733910846065));
#11000=CARTESIAN_POINT('Ctrl Pts',(96.649962047086,-0.440416778753674,2.1613601370602));
#11001=CARTESIAN_POINT('Ctrl Pts',(96.6547767304487,-0.526336028431881,
2.14023045141745));
#11002=CARTESIAN_POINT('Ctrl Pts',(96.6581371028647,-0.586302729224979,
2.12548314459697));
#11003=CARTESIAN_POINT('Ctrl Pts',(96.6614974752808,-0.645595498506252,
2.10822782962978));
#11004=CARTESIAN_POINT('Ctrl Pts',(96.6648578476968,-0.704026432666069,
2.08853124997149));
#11005=CARTESIAN_POINT('Ctrl Pts',(96.6689309126328,-0.774849829492498,
2.06465727469931));
#11006=CARTESIAN_POINT('Ctrl Pts',(96.6730039775688,-0.844594055879215,
2.03713067829103));
#11007=CARTESIAN_POINT('Ctrl Pts',(96.6770770425048,-0.912855719265293,
2.00606840257371));
#11008=CARTESIAN_POINT('Ctrl Pts',(96.6811441233099,-0.981017092884918,
1.97505176342929));
#11009=CARTESIAN_POINT('Ctrl Pts',(96.685211204115,-1.04769979709705,1.94050995450216));
#11010=CARTESIAN_POINT('Ctrl Pts',(96.6892782849201,-1.11251708334427,1.9026091924689));
#11011=CARTESIAN_POINT('Ctrl Pts',(96.693340607289,-1.17725853413712,1.86475277387667));
#11012=CARTESIAN_POINT('Ctrl Pts',(96.6974029296579,-1.2401384930298,1.82354544986018));
#11013=CARTESIAN_POINT('Ctrl Pts',(96.7014652520268,-1.30079313252182,1.77920016478868));
#11014=CARTESIAN_POINT('Ctrl Pts',(96.7055249961661,-1.36140927640207,1.73488302428934));
#11015=CARTESIAN_POINT('Ctrl Pts',(96.7095847403054,-1.41980251906175,1.68743215586438));
#11016=CARTESIAN_POINT('Ctrl Pts',(96.7136444844448,-1.47563759686912,1.63710405371996));
#11017=CARTESIAN_POINT('Ctrl Pts',(96.7177029638998,-1.53145528103266,1.58679162969614));
#11018=CARTESIAN_POINT('Ctrl Pts',(96.7217614433549,-1.58471602816388,1.53360407100371));
#11019=CARTESIAN_POINT('Ctrl Pts',(96.72581992281,-1.63511854420886,1.47783738834294));
#11020=CARTESIAN_POINT('Ctrl Pts',(96.7298784494424,-1.68552164615227,1.4220700574286));
#11021=CARTESIAN_POINT('Ctrl Pts',(96.7339369760748,-1.73306613222038,1.3637238984421));
#11022=CARTESIAN_POINT('Ctrl Pts',(96.7379955027072,-1.77748950095122,1.30312972263247));
#11023=CARTESIAN_POINT('Ctrl Pts',(96.7420581796923,-1.82195829815037,1.24247358167534));
#11024=CARTESIAN_POINT('Ctrl Pts',(96.7461208566774,-1.8632993213725,1.17956521908401));
#11025=CARTESIAN_POINT('Ctrl Pts',(96.7501835336626,-1.90129257785128,1.11476568542794));
#11026=CARTESIAN_POINT('Ctrl Pts',(96.7542483326396,-1.93930567872936,1.04993230608611));
#11027=CARTESIAN_POINT('Ctrl Pts',(96.7583131316167,-1.97396731042543,0.983206212701497));
#11028=CARTESIAN_POINT('Ctrl Pts',(96.7623779305937,-2.00510403363176,0.914972029252061));
#11029=CARTESIAN_POINT('Ctrl Pts',(96.7664499908358,-2.03629637877627,0.846615953800434));
#11030=CARTESIAN_POINT('Ctrl Pts',(96.7705220510778,-2.06395106204914,0.776746851801219));
#11031=CARTESIAN_POINT('Ctrl Pts',(96.7745941113198,-2.08794343724145,0.705767810884249));
#11032=CARTESIAN_POINT('Ctrl Pts',(96.7777322621185,-2.10643326472366,0.651067506688116));
#11033=CARTESIAN_POINT('Ctrl Pts',(96.7808704129172,-2.12274901846192,0.595708394515493));
#11034=CARTESIAN_POINT('Ctrl Pts',(96.7840085637159,-2.13685439413681,0.539878966304667));
#11035=CARTESIAN_POINT('Ctrl Pts',(96.7880816286519,-2.15516202648322,0.4674169015322));
#11036=CARTESIAN_POINT('Ctrl Pts',(96.7921546935879,-2.16981493522022,0.393882808150005));
#11037=CARTESIAN_POINT('Ctrl Pts',(96.7962277585238,-2.18069284290564,0.319679096751906));
#11038=CARTESIAN_POINT('Ctrl Pts',(96.8002948393289,-2.19155476881201,0.245584405153781));
#11039=CARTESIAN_POINT('Ctrl Pts',(96.8043619201339,-2.19865263649152,0.170822517274372));
#11040=CARTESIAN_POINT('Ctrl Pts',(96.8084290009389,-2.20191660179042,0.0958085526439572));
#11041=CARTESIAN_POINT('Ctrl Pts',(96.8124913233078,-2.20517674828873,0.0208823534603541));
#11042=CARTESIAN_POINT('Ctrl Pts',(96.8165536456766,-2.20461188365891,-0.0542948619096966));
#11043=CARTESIAN_POINT('Ctrl Pts',(96.8206159680455,-2.20020385720147,-0.129301920928357));
#11044=CARTESIAN_POINT('Ctrl Pts',(96.8246757121848,-2.19579862838122,-0.20426137530135));
#11045=CARTESIAN_POINT('Ctrl Pts',(96.8287354563241,-2.1875551058737,-0.279050412192913));
#11046=CARTESIAN_POINT('Ctrl Pts',(96.8327952004633,-2.17550721885559,-0.35324827063585));
#11047=CARTESIAN_POINT('Ctrl Pts',(96.8368536799184,-2.16346308497376,-0.427423015094262));
#11048=CARTESIAN_POINT('Ctrl Pts',(96.8409121593734,-2.14761701607951,-0.501006475770795));
#11049=CARTESIAN_POINT('Ctrl Pts',(96.8449706388284,-2.1280545601486,-0.573585032083948));
#11050=CARTESIAN_POINT('Ctrl Pts',(96.8490291654608,-2.10849187681611,-0.646164432078399));
#11051=CARTESIAN_POINT('Ctrl Pts',(96.8530876920932,-2.08521284665938,-0.717738443973867));
#11052=CARTESIAN_POINT('Ctrl Pts',(96.8571462187255,-2.05835328593649,-0.787907196486008));
#11053=CARTESIAN_POINT('Ctrl Pts',(96.8612088957106,-2.03146625794269,-0.858147705351686));
#11054=CARTESIAN_POINT('Ctrl Pts',(96.8652715726957,-2.00099155855932,-0.926979638219817));
#11055=CARTESIAN_POINT('Ctrl Pts',(96.8693342496808,-1.96711345210214,-0.994022467834));
#11056=CARTESIAN_POINT('Ctrl Pts',(96.8733990486578,-1.933217650645,-1.06110031483822));
#11057=CARTESIAN_POINT('Ctrl Pts',(96.8774638476348,-1.89591513919266,-1.12638678272741));
#11058=CARTESIAN_POINT('Ctrl Pts',(96.8815286466119,-1.85543521899374,-1.18952769960084));
#11059=CARTESIAN_POINT('Ctrl Pts',(96.8856007068539,-1.81488298638082,-1.25278140998025));
#11060=CARTESIAN_POINT('Ctrl Pts',(96.8896727670959,-1.77114228589202,-1.31388152488797));
#11061=CARTESIAN_POINT('Ctrl Pts',(96.8937448273379,-1.72448437447102,-1.37250487875464));
#11062=CARTESIAN_POINT('Ctrl Pts',(96.8968829781369,-1.68852725367541,-1.41768321940962));
#11063=CARTESIAN_POINT('Ctrl Pts',(96.900021128936,-1.65083845080548,-1.46139121935922));
#11064=CARTESIAN_POINT('Ctrl Pts',(96.903159279735,-1.61155672181826,-1.50349623623154));
#11065=CARTESIAN_POINT('Ctrl Pts',(96.907232344671,-1.5605722270612,-1.55814512942743));
#11066=CARTESIAN_POINT('Ctrl Pts',(96.911305409607,-1.50670649418841,-1.6103030957032));
#11067=CARTESIAN_POINT('Ctrl Pts',(96.9153784745429,-1.45023257818622,-1.65965100824461));
#11068=CARTESIAN_POINT('Ctrl Pts',(96.9194455553479,-1.39384163343858,-1.70892641902764));
#11069=CARTESIAN_POINT('Ctrl Pts',(96.923512636153,-1.33485047006253,-1.75539966131159));
#11070=CARTESIAN_POINT('Ctrl Pts',(96.927579716958,-1.2735701506229,-1.79878711120643));
#11071=CARTESIAN_POINT('Ctrl Pts',(96.9316420393268,-1.21236152842848,-1.8421237983007));
#11072=CARTESIAN_POINT('Ctrl Pts',(96.9357043616957,-1.14886945903196,-1.88238159141643));
#11073=CARTESIAN_POINT('Ctrl Pts',(96.9397666840645,-1.08343810109065,-1.91931703506875));
#11074=CARTESIAN_POINT('Ctrl Pts',(96.9438264282038,-1.01804827039561,-1.95622903694463));
#11075=CARTESIAN_POINT('Ctrl Pts',(96.9478861723431,-0.950722008292447,
-1.98982263951525));
#11076=CARTESIAN_POINT('Ctrl Pts',(96.9519459164823,-0.881831345461783,
-2.01989838312749));
#11077=CARTESIAN_POINT('Ctrl Pts',(96.9560043959374,-0.812962143327503,
-2.04996475759774));
#11078=CARTESIAN_POINT('Ctrl Pts',(96.9600628753924,-0.742529945349692,
-2.07651525801702));
#11079=CARTESIAN_POINT('Ctrl Pts',(96.9641213548474,-0.670928748881124,
-2.09939767884144));
#11080=CARTESIAN_POINT('Ctrl Pts',(96.9681798814798,-0.599326720092509,
-2.12228036565998));
#11081=CARTESIAN_POINT('Ctrl Pts',(96.9722384081121,-0.526556121178033,
-2.14149474458408));
#11082=CARTESIAN_POINT('Ctrl Pts',(96.9762969347445,-0.45302662967315,-2.15693830992149));
#11083=CARTESIAN_POINT('Ctrl Pts',(96.9803596117295,-0.379421945037426,
-2.17239766824217));
#11084=CARTESIAN_POINT('Ctrl Pts',(96.9844222887146,-0.305057286361621,
-2.18407841414576));
#11085=CARTESIAN_POINT('Ctrl Pts',(96.9884849656997,-0.230352322789945,
-2.19192924324333));
#11086=CARTESIAN_POINT('Ctrl Pts',(96.9925497646767,-0.155608339790519,
-2.19978417293669));
#11087=CARTESIAN_POINT('Ctrl Pts',(96.9966145636537,-0.080524175152663,
-2.20380517662948));
#11088=CARTESIAN_POINT('Ctrl Pts',(97.0006793626307,-0.00552174843155068,
-2.20399308308676));
#11089=CARTESIAN_POINT('Ctrl Pts',(97.0047514228727,0.0696146609284717,
-2.20418132521588));
#11090=CARTESIAN_POINT('Ctrl Pts',(97.0088234831146,0.144668563116419,-2.20052281632401));
#11091=CARTESIAN_POINT('Ctrl Pts',(97.0128955433566,0.2192213667622,-2.19307044856177));
#11092=CARTESIAN_POINT('Ctrl Pts',(97.0160336941558,0.276675806637948,-2.18732724918376));
#11093=CARTESIAN_POINT('Ctrl Pts',(97.019171844955,0.33383269456276,-2.17933192027265));
#11094=CARTESIAN_POINT('Ctrl Pts',(97.0223099957542,0.390505364565229,-2.16912921704673));
#11095=CARTESIAN_POINT('Ctrl Pts',(97.0263830606903,0.464061888708159,-2.15588693666489));
#11096=CARTESIAN_POINT('Ctrl Pts',(97.0304561256265,0.537085917159001,-2.13887335699214));
#11097=CARTESIAN_POINT('Ctrl Pts',(97.0345291905626,0.609161278881517,-2.11814506970402));
#11098=CARTESIAN_POINT('Ctrl Pts',(97.0385962713678,0.681130747767004,-2.09744723633379));
#11099=CARTESIAN_POINT('Ctrl Pts',(97.0426633521731,0.752153862088602,-2.07304566184749));
#11100=CARTESIAN_POINT('Ctrl Pts',(97.0467304329783,0.821823697525992,-2.04504811928343));
#11101=CARTESIAN_POINT('Ctrl Pts',(97.0507927553473,0.891412020084187,-2.01708333351133));
#11102=CARTESIAN_POINT('Ctrl Pts',(97.0548550777163,0.959649768653953,-1.98553111562693));
#11103=CARTESIAN_POINT('Ctrl Pts',(97.0589174000853,1.02614584808455,-1.95054881980914));
#11104=CARTESIAN_POINT('Ctrl Pts',(97.0629771442248,1.0925997245233,-1.91558872616564));
#11105=CARTESIAN_POINT('Ctrl Pts',(97.0670368883643,1.15731370385263,-1.87720309627234));
#11106=CARTESIAN_POINT('Ctrl Pts',(97.0710966325037,1.21991856752921,-1.8355965484271));
#11107=CARTESIAN_POINT('Ctrl Pts',(97.0751551119589,1.28250392865033,-1.79400296177942));
#11108=CARTESIAN_POINT('Ctrl Pts',(97.0792135914141,1.34298108122692,-1.74919071344024));
#11109=CARTESIAN_POINT('Ctrl Pts',(97.0832720708693,1.40100862152683,-1.70140848781458));
#11110=CARTESIAN_POINT('Ctrl Pts',(97.0873305975019,1.45903683636136,-1.65362570674981));
#11111=CARTESIAN_POINT('Ctrl Pts',(97.0913891241344,1.51461501493786,-1.60287318473939));
#11112=CARTESIAN_POINT('Ctrl Pts',(97.095447650767,1.56743503011681,-1.54943971369096));
#11113=CARTESIAN_POINT('Ctrl Pts',(97.0995103277522,1.62030906038859,-1.4959516002141));
#11114=CARTESIAN_POINT('Ctrl Pts',(97.1035730047375,1.67041895834268,-1.43977740318065));
#11115=CARTESIAN_POINT('Ctrl Pts',(97.1076356817227,1.71749421757976,-1.38124205430478));
#11116=CARTESIAN_POINT('Ctrl Pts',(97.1117004806999,1.76459406487082,-1.32267613161283));
#11117=CARTESIAN_POINT('Ctrl Pts',(97.1157652796771,1.80865583695665,-1.26174698841172));
#11118=CARTESIAN_POINT('Ctrl Pts',(97.1198300786543,1.84945162573308,-1.19880969468605));
#11119=CARTESIAN_POINT('Ctrl Pts',(97.1239021388965,1.89032029118394,-1.13575997120228));
#11120=CARTESIAN_POINT('Ctrl Pts',(97.1279741991386,1.92791108059944,-1.07069534584733));
#11121=CARTESIAN_POINT('Ctrl Pts',(97.1320462593808,1.96204164812848,-1.00399630029662));
#11122=CARTESIAN_POINT('Ctrl Pts',(97.1351844101783,1.98834451727579,-0.952594393021613));
#11123=CARTESIAN_POINT('Ctrl Pts',(97.1383225609758,2.01259326484021,-0.900222326425294));
#11124=CARTESIAN_POINT('Ctrl Pts',(97.1414607117732,2.03472436786831,-0.847061241471294));
#11125=CARTESIAN_POINT('Ctrl Pts',(97.145533776709,2.06344874268377,-0.778062469567536));
#11126=CARTESIAN_POINT('Ctrl Pts',(97.1496068416448,2.08871484518926,-0.707467889834191));
#11127=CARTESIAN_POINT('Ctrl Pts',(97.1536799065806,2.1103447503495,-0.635657954148531));
#11128=CARTESIAN_POINT('Ctrl Pts',(97.1577469873855,2.13194287693844,-0.563953521337008));
#11129=CARTESIAN_POINT('Ctrl Pts',(97.1618140681903,2.14991527623945,-0.491037731086796));
#11130=CARTESIAN_POINT('Ctrl Pts',(97.1658811489952,2.16413205091675,-0.417310994577013));
#11131=CARTESIAN_POINT('Ctrl Pts',(97.1699434713639,2.17833219213671,-0.343670517472408));
#11132=CARTESIAN_POINT('Ctrl Pts',(97.1740057937325,2.18878534873056,-0.269221445620318));
#11133=CARTESIAN_POINT('Ctrl Pts',(97.1780681161012,2.19541187259309,-0.194377749954301));
#11134=CARTESIAN_POINT('Ctrl Pts',(97.1821278602403,2.20203419080719,-0.119581555252327));
#11135=CARTESIAN_POINT('Ctrl Pts',(97.1861876043794,2.20483465367082,-0.0443917081330866));
#11136=CARTESIAN_POINT('Ctrl Pts',(97.1902473485185,2.20378519149202,0.0307705989617547));
#11137=CARTESIAN_POINT('Ctrl Pts',(97.1943058279734,2.20273605623982,0.105909491628809));
#11138=CARTESIAN_POINT('Ctrl Pts',(97.1983643074282,2.19783938380886,0.181020384202449));
#11139=CARTESIAN_POINT('Ctrl Pts',(97.2024227868831,2.18911921245078,0.255681586507276));
#11140=CARTESIAN_POINT('Ctrl Pts',(97.2064813135153,2.18039893972605,0.330343656702817));
#11141=CARTESIAN_POINT('Ctrl Pts',(97.2105398401475,2.16785513699549,0.404555552221366));
#11142=CARTESIAN_POINT('Ctrl Pts',(97.2145983667797,2.1515635825754,0.477901820602631));
#11143=CARTESIAN_POINT('Ctrl Pts',(97.2186610437646,2.13525536799677,0.551323094746271));
#11144=CARTESIAN_POINT('Ctrl Pts',(97.2227237207495,2.11519185211197,0.623876506897386));
#11145=CARTESIAN_POINT('Ctrl Pts',(97.2267863977345,2.09149957222474,0.695158643320879));
#11146=CARTESIAN_POINT('Ctrl Pts',(97.2308511967113,2.06779491753456,0.766478011382557));
#11147=CARTESIAN_POINT('Ctrl Pts',(97.2349159956882,2.04045789817965,0.836524336214279));
#11148=CARTESIAN_POINT('Ctrl Pts',(97.238980794665,2.0096634631363,0.904913678167703));
#11149=CARTESIAN_POINT('Ctrl Pts',(97.2430528549069,1.97881401761057,0.973425189295053));
#11150=CARTESIAN_POINT('Ctrl Pts',(97.2471249151487,1.94449503820559,1.040273379795));
#11151=CARTESIAN_POINT('Ctrl Pts',(97.2511969753905,1.90692751884061,1.1050988362533));
#11152=CARTESIAN_POINT('Ctrl Pts',(97.2543351261912,1.87797594789814,1.15505685406376));
#11153=CARTESIAN_POINT('Ctrl Pts',(97.2574732769918,1.84709599841897,1.2038140468137));
#11154=CARTESIAN_POINT('Ctrl Pts',(97.2606114277925,1.81440550029416,1.25121887793555));
#11155=CARTESIAN_POINT('Ctrl Pts',(97.2646637681727,1.77219177825978,1.31243343503482));
#11156=CARTESIAN_POINT('Ctrl Pts',(97.2687161085529,1.72679109134377,1.37163325595954));
#11157=CARTESIAN_POINT('Ctrl Pts',(97.2727684489331,1.67842324522032,1.42846470376558));
#11158=CARTESIAN_POINT('Ctrl Pts',(97.2768148242482,1.63012659680576,1.48521249539917));
#11159=CARTESIAN_POINT('Ctrl Pts',(97.2808611995633,1.5788717685914,1.53959846900412));
#11160=CARTESIAN_POINT('Ctrl Pts',(97.2849075748784,1.52492150538961,1.59129833859032));
#11161=CARTESIAN_POINT('Ctrl Pts',(97.2889492578127,1.47103380563322,1.642938254401));
#11162=CARTESIAN_POINT('Ctrl Pts',(97.292990940747,1.41445722629823,1.69189792081092));
#11163=CARTESIAN_POINT('Ctrl Pts',(97.2970326236813,1.35549325620361,1.73788780776739));
#11164=CARTESIAN_POINT('Ctrl Pts',(97.3010718017673,1.29656582925137,1.78384919231833));
#11165=CARTESIAN_POINT('Ctrl Pts',(97.3051109798534,1.23525432669,1.82684415250284));
#11166=CARTESIAN_POINT('Ctrl Pts',(97.3091501579395,1.17189432754206,1.86662253417094));
#11167=CARTESIAN_POINT('Ctrl Pts',(97.3131881726005,1.1085525782978,1.90638945826891));
#11168=CARTESIAN_POINT('Ctrl Pts',(97.3172261872615,1.04316391258803,1.94294138651562));
#11169=CARTESIAN_POINT('Ctrl Pts',(97.3212642019225,0.976092579314091,1.9760716780036));
#11170=CARTESIAN_POINT('Ctrl Pts',(97.3253023929626,0.909018316386416,2.00920341661179));
#11171=CARTESIAN_POINT('Ctrl Pts',(97.3293405840028,0.840261674001143,2.03891301004312));
#11172=CARTESIAN_POINT('Ctrl Pts',(97.3333787750429,0.770209643490197,2.06504070300677));
#11173=CARTESIAN_POINT('Ctrl Pts',(97.3374210894093,0.700086084075982,2.09119507450078));
#11174=CARTESIAN_POINT('Ctrl Pts',(97.3414634037757,0.628664949918502,2.11376007679749));
#11175=CARTESIAN_POINT('Ctrl Pts',(97.3455057181421,0.556350434859627,2.13262518826715));
#11176=CARTESIAN_POINT('Ctrl Pts',(97.3495503257518,0.48399489509044,2.15150100209349));
#11177=CARTESIAN_POINT('Ctrl Pts',(97.3535949333615,0.41074543875725,2.16667265050363));
#11178=CARTESIAN_POINT('Ctrl Pts',(97.3576395409712,0.337015916512282,2.17808086902608));
#11179=CARTESIAN_POINT('Ctrl Pts',(97.3616909554316,0.263162311562423,2.18950828694883));
#11180=CARTESIAN_POINT('Ctrl Pts',(97.365742369892,0.188827508213047,2.1971595846685));
#11181=CARTESIAN_POINT('Ctrl Pts',(97.3697937843524,0.114429203377559,2.20102747766001));
#11182=CARTESIAN_POINT('Ctrl Pts',(97.3718786584933,0.0761435371257581,
2.20301791091649));
#11183=CARTESIAN_POINT('Ctrl Pts',(97.3739635326342,0.0378410376971126,
2.20400728289753));
#11184=CARTESIAN_POINT('Ctrl Pts',(97.3760484067751,-0.000421831323937878,
2.20399995963211));
#11185=CARTESIAN_POINT('',(98.1260484067631,0.00200370534590846,2.2039990891933));
#11186=CARTESIAN_POINT('Ctrl Pts',(97.3760484068025,-0.00042183182640112,
2.20399995963201));
#11187=CARTESIAN_POINT('Ctrl Pts',(97.3772863191389,-0.023140746438742,
2.20399561137365));
#11188=CARTESIAN_POINT('Ctrl Pts',(97.3785242314752,-0.0458559000617912,
2.20363999219748));
#11189=CARTESIAN_POINT('Ctrl Pts',(97.3797621438116,-0.0685600735653428,
2.20293338898677));
#11190=CARTESIAN_POINT('Ctrl Pts',(97.3838352087488,-0.143262918273813,
2.20060847414624));
#11191=CARTESIAN_POINT('Ctrl Pts',(97.387908273686,-0.217991429363417,2.19447493865576));
#11192=CARTESIAN_POINT('Ctrl Pts',(97.3919813386232,-0.292325635221059,
2.18452780320888));
#11193=CARTESIAN_POINT('Ctrl Pts',(97.3960484194294,-0.36655062955683,2.17459528205414));
#11194=CARTESIAN_POINT('Ctrl Pts',(97.4001155002357,-0.440381999516932,
2.16086034783918));
#11195=CARTESIAN_POINT('Ctrl Pts',(97.4041825810419,-0.513401423440742,
2.14337000501757));
#11196=CARTESIAN_POINT('Ctrl Pts',(97.408244903412,-0.586335415506716,2.12590012568912));
#11197=CARTESIAN_POINT('Ctrl Pts',(97.4123072257821,-0.658458886911531,
2.10468367785998));
#11198=CARTESIAN_POINT('Ctrl Pts',(97.4163695481522,-0.729361911800216,
2.07981903097725));
#11199=CARTESIAN_POINT('Ctrl Pts',(97.4204292922927,-0.800219936745927,
2.05497016491196));
#11200=CARTESIAN_POINT('Ctrl Pts',(97.4244890364332,-0.869858602827608,
2.02647785205489));
#11201=CARTESIAN_POINT('Ctrl Pts',(97.4285487805737,-0.93788270160062,1.99449042064341));
#11202=CARTESIAN_POINT('Ctrl Pts',(97.4326072600299,-1.00588560962769,1.96251295389952));
#11203=CARTESIAN_POINT('Ctrl Pts',(97.4366657394862,-1.07227451717383,1.9270427333978));
#11204=CARTESIAN_POINT('Ctrl Pts',(97.4407242189425,-1.13667527580074,1.88827575247455));
#11205=CARTESIAN_POINT('Ctrl Pts',(97.444782745576,-1.20107678304696,1.84950832090892));
#11206=CARTESIAN_POINT('Ctrl Pts',(97.4488412722096,-1.26348968734669,1.80744430060874));
#11207=CARTESIAN_POINT('Ctrl Pts',(97.4528997988432,-1.32356688299169,1.76232423414298));
#11208=CARTESIAN_POINT('Ctrl Pts',(97.4569624758295,-1.38370551510689,1.71715802674823));
#11209=CARTESIAN_POINT('Ctrl Pts',(97.4610251528158,-1.44150328613208,1.66892981972681));
#11210=CARTESIAN_POINT('Ctrl Pts',(97.4650878298021,-1.49664501156592,1.61792141631009));
#11211=CARTESIAN_POINT('Ctrl Pts',(97.4691526287803,-1.55181553827964,1.5668863705043));
#11212=CARTESIAN_POINT('Ctrl Pts',(97.4732174277585,-1.6043269229983,1.51306857857434));
#11213=CARTESIAN_POINT('Ctrl Pts',(97.4772822267367,-1.65390170539555,1.45678589672254));
#11214=CARTESIAN_POINT('Ctrl Pts',(97.4813542869799,-1.70356504706262,1.40040267276108));
#11215=CARTESIAN_POINT('Ctrl Pts',(97.485426347223,-1.7502810108955,1.34154613831157));
#11216=CARTESIAN_POINT('Ctrl Pts',(97.4894984074662,-1.79381348507808,1.28056596110939));
#11217=CARTESIAN_POINT('Ctrl Pts',(97.4926365582544,-1.82736197405157,1.23357132455627));
#11218=CARTESIAN_POINT('Ctrl Pts',(97.4957747090425,-1.85902060639208,1.18531610622014));
#11219=CARTESIAN_POINT('Ctrl Pts',(97.4989128598307,-1.88870001086929,1.13597018840388));
#11220=CARTESIAN_POINT('Ctrl Pts',(97.5029859247648,-1.9272214681866,1.07192319351211));
#11221=CARTESIAN_POINT('Ctrl Pts',(97.5070589896989,-1.96255570848192,1.00579103732401));
#11222=CARTESIAN_POINT('Ctrl Pts',(97.5111320546331,-1.99447099743568,0.937924005657145));
#11223=CARTESIAN_POINT('Ctrl Pts',(97.5151991354363,-2.02633939657287,0.870156683965339));
#11224=CARTESIAN_POINT('Ctrl Pts',(97.5192662162395,-2.05479861579184,0.800659975828997));
#11225=CARTESIAN_POINT('Ctrl Pts',(97.5233332970427,-2.07966150680036,0.729810946158569));
#11226=CARTESIAN_POINT('Ctrl Pts',(97.5273956194097,-2.10449530852207,0.659044809010307));
#11227=CARTESIAN_POINT('Ctrl Pts',(97.5314579417767,-2.12574098438867,0.586929942059288));
#11228=CARTESIAN_POINT('Ctrl Pts',(97.5355202641437,-2.14325910710736,0.513864184197897));
#11229=CARTESIAN_POINT('Ctrl Pts',(97.5395800082812,-2.16076611161887,0.440844798898597));
#11230=CARTESIAN_POINT('Ctrl Pts',(97.5436397524187,-2.17455014654319,0.366876183396631));
#11231=CARTESIAN_POINT('Ctrl Pts',(97.5476994965561,-2.18452174885648,0.292370875384411));
#11232=CARTESIAN_POINT('Ctrl Pts',(97.5517579760094,-2.19449024483403,0.217888777132598));
#11233=CARTESIAN_POINT('Ctrl Pts',(97.5558164554626,-2.20064860291723,0.142870791250414));
#11234=CARTESIAN_POINT('Ctrl Pts',(97.5598749349159,-2.20295883306561,0.0677375805460152));
#11235=CARTESIAN_POINT('Ctrl Pts',(97.5639334615465,-2.205269090069,-0.00739650353620468));
#11236=CARTESIAN_POINT('Ctrl Pts',(97.567991988177,-2.20373111743813,-0.0826453378098284));
#11237=CARTESIAN_POINT('Ctrl Pts',(97.5720505148076,-2.19835902081088,-0.157586851035928));
#11238=CARTESIAN_POINT('Ctrl Pts',(97.576113191791,-2.19298143054075,-0.232605001362973));
#11239=CARTESIAN_POINT('Ctrl Pts',(97.5801758687743,-2.18376192072935,-0.307314725757909));
#11240=CARTESIAN_POINT('Ctrl Pts',(97.5842385457576,-2.17076657192755,-0.381298426697426));
#11241=CARTESIAN_POINT('Ctrl Pts',(97.5883033447329,-2.15776443547665,-0.455320770339663));
#11242=CARTESIAN_POINT('Ctrl Pts',(97.5923681437082,-2.14098263930786,-0.52861586951254));
#11243=CARTESIAN_POINT('Ctrl Pts',(97.5964329426835,-2.12053800601775,-0.600778299403589));
#11244=CARTESIAN_POINT('Ctrl Pts',(97.6005050029238,-2.10005685089683,-0.67306963862836));
#11245=CARTESIAN_POINT('Ctrl Pts',(97.6045770631641,-2.0758999428233,-0.744223814250836));
#11246=CARTESIAN_POINT('Ctrl Pts',(97.6086491234044,-2.0482332452747,-0.813852918500303));
#11247=CARTESIAN_POINT('Ctrl Pts',(97.6117872742196,-2.02691178529126,-0.867512888481555));
#11248=CARTESIAN_POINT('Ctrl Pts',(97.6149254250347,-2.003506850464,-0.920267453980305));
#11249=CARTESIAN_POINT('Ctrl Pts',(97.6180635758498,-1.97811280272008,-0.971949453271568));
#11250=CARTESIAN_POINT('Ctrl Pts',(97.6221366407851,-1.94515339078515,-1.03902849169189));
#11251=CARTESIAN_POINT('Ctrl Pts',(97.6262097057203,-1.90871451324376,-1.10455847585856));
#11252=CARTESIAN_POINT('Ctrl Pts',(97.6302827706556,-1.86896502488545,-1.16815484237105));
#11253=CARTESIAN_POINT('Ctrl Pts',(97.6343498514599,-1.82927393631882,-1.23165777335243));
#11254=CARTESIAN_POINT('Ctrl Pts',(97.6384169322642,-1.78628214479456,-1.29323232543297));
#11255=CARTESIAN_POINT('Ctrl Pts',(97.6424840130685,-1.7402051703996,-1.35251690004764));
#11256=CARTESIAN_POINT('Ctrl Pts',(97.6465463354365,-1.69418210551725,-1.41173211241437));
#11257=CARTESIAN_POINT('Ctrl Pts',(97.6506086578046,-1.64508132079815,-1.46866229527368));
#11258=CARTESIAN_POINT('Ctrl Pts',(97.6546709801727,-1.59316165295788,-1.52297470351432));
#11259=CARTESIAN_POINT('Ctrl Pts',(97.6587307243112,-1.54127493691497,-1.57725264135973));
#11260=CARTESIAN_POINT('Ctrl Pts',(97.6627904684497,-1.48657321703343,-1.62891575723723));
#11261=CARTESIAN_POINT('Ctrl Pts',(97.6668502125881,-1.42935475595175,-1.67766533660266));
#11262=CARTESIAN_POINT('Ctrl Pts',(97.6709086920424,-1.37215411946322,-1.72639972958589));
#11263=CARTESIAN_POINT('Ctrl Pts',(97.6749671714966,-1.31243866159608,-1.77222207865274));
#11264=CARTESIAN_POINT('Ctrl Pts',(97.6790256509508,-1.25054136322061,-1.81487252964894));
#11265=CARTESIAN_POINT('Ctrl Pts',(97.6830841775824,-1.1886433453272,-1.85752347643034));
#11266=CARTESIAN_POINT('Ctrl Pts',(97.6871427042139,-1.12456383074711,-1.89700218249863));
#11267=CARTESIAN_POINT('Ctrl Pts',(97.6912012308455,-1.05866521063653,-1.93309181669881));
#11268=CARTESIAN_POINT('Ctrl Pts',(97.6952639078297,-0.99269920091883,-1.969218357078));
#11269=CARTESIAN_POINT('Ctrl Pts',(97.6993265848139,-0.924910790533539,
-2.00194867482967));
#11270=CARTESIAN_POINT('Ctrl Pts',(97.7033892617981,-0.855686771579625,
-2.03111204736313));
#11271=CARTESIAN_POINT('Ctrl Pts',(97.7074540607743,-0.786426595970732,
-2.06029065232623));
#11272=CARTESIAN_POINT('Ctrl Pts',(97.7115188597505,-0.715729767899791,
-2.08589843920142));
#11273=CARTESIAN_POINT('Ctrl Pts',(97.7155836587266,-0.644000341454866,
-2.10781392921814));
#11274=CARTESIAN_POINT('Ctrl Pts',(97.7196557189678,-0.572142779184829,
-2.12976856857057));
#11275=CARTESIAN_POINT('Ctrl Pts',(97.7237277792089,-0.499249397928626,
-2.14801762026816));
#11276=CARTESIAN_POINT('Ctrl Pts',(97.72779983945,-0.425736154340295,-2.16249039925904));
#11277=CARTESIAN_POINT('Ctrl Pts',(97.7309379902564,-0.369082855768432,
-2.17364390887598));
#11278=CARTESIAN_POINT('Ctrl Pts',(97.7340761410627,-0.312061674981444,
-2.18255570322988));
#11279=CARTESIAN_POINT('Ctrl Pts',(97.737214291869,-0.254864237668701,-2.18921452131982));
#11280=CARTESIAN_POINT('Ctrl Pts',(97.741287356814,-0.180626608172958,-2.19785712653895));
#11281=CARTESIAN_POINT('Ctrl Pts',(97.745360421759,-0.105805703914654,-2.20273595165285));
#11282=CARTESIAN_POINT('Ctrl Pts',(97.749433486704,-0.0308162371980697,
-2.20378455379036));
#11283=CARTESIAN_POINT('Ctrl Pts',(97.7535005675181,0.0440630552907173,
-2.20483161532574));
#11284=CARTESIAN_POINT('Ctrl Pts',(97.7575676483323,0.11910994509809,-2.20205961984711));
#11285=CARTESIAN_POINT('Ctrl Pts',(97.7616347291464,0.193903737515108,-2.19545378921481));
#11286=CARTESIAN_POINT('Ctrl Pts',(97.7656970515243,0.26861002208437,-2.1888556873258));
#11287=CARTESIAN_POINT('Ctrl Pts',(97.7697593739022,0.343063324368703,-2.17843270382538));
#11288=CARTESIAN_POINT('Ctrl Pts',(97.7738216962801,0.416843730981485,-2.16422210134298));
#11289=CARTESIAN_POINT('Ctrl Pts',(97.7778814404284,0.490577311466708,-2.15002051788766));
#11290=CARTESIAN_POINT('Ctrl Pts',(97.7819411845768,0.563638376091331,-2.13203617577166));
#11291=CARTESIAN_POINT('Ctrl Pts',(97.7860009287251,0.635614252189,-2.11035791334414));
#11292=CARTESIAN_POINT('Ctrl Pts',(97.7900594081892,0.707567706489905,-2.08868640409033));
#11293=CARTESIAN_POINT('Ctrl Pts',(97.7941178876532,0.778436186583184,-2.06332339684287));
#11294=CARTESIAN_POINT('Ctrl Pts',(97.7981763671173,0.847820870684519,-2.03440796578065));
#11295=CARTESIAN_POINT('Ctrl Pts',(97.8022348937587,0.917206361339779,-2.00549219859447));
#11296=CARTESIAN_POINT('Ctrl Pts',(97.8062934204001,0.985107581724493,-1.97302411092295));
#11297=CARTESIAN_POINT('Ctrl Pts',(97.8103519470415,1.05114593553944,-1.93719080686414));
#11298=CARTESIAN_POINT('Ctrl Pts',(97.8144146240354,1.11725182185513,-1.90132085875693));
#11299=CARTESIAN_POINT('Ctrl Pts',(97.8184773010294,1.1814906168022,-1.86207905029068));
#11300=CARTESIAN_POINT('Ctrl Pts',(97.8225399780234,1.24350925713102,-1.8196979769812));
#11301=CARTESIAN_POINT('Ctrl Pts',(97.8266047770093,1.30556029064606,-1.77729476745601));
#11302=CARTESIAN_POINT('Ctrl Pts',(97.8306695759951,1.36538848002121,-1.73174931730094));
#11303=CARTESIAN_POINT('Ctrl Pts',(97.834734374981,1.42267279825242,-1.68333541194636));
#11304=CARTESIAN_POINT('Ctrl Pts',(97.8388064352317,1.48005944789153,-1.63483502108843));
#11305=CARTESIAN_POINT('Ctrl Pts',(97.8428784954824,1.53489280054329,-1.58345626689899));
#11306=CARTESIAN_POINT('Ctrl Pts',(97.8469505557331,1.58688807197544,-1.52951045992569));
#11307=CARTESIAN_POINT('Ctrl Pts',(97.8500887064514,1.6269584511819,-1.48793689212848));
#11308=CARTESIAN_POINT('Ctrl Pts',(97.8532268571698,1.66534400792165,-1.44483951419821));
#11309=CARTESIAN_POINT('Ctrl Pts',(97.8563650078881,1.70193145066577,-1.4003732849618));
#11310=CARTESIAN_POINT('Ctrl Pts',(97.8604380728076,1.74941898167051,-1.34265972858413));
#11311=CARTESIAN_POINT('Ctrl Pts',(97.8645111377271,1.7940591075753,-1.28241663984275));
#11312=CARTESIAN_POINT('Ctrl Pts',(97.8685842026466,1.83557128389276,-1.21995658191113));
#11313=CARTESIAN_POINT('Ctrl Pts',(97.8726512834352,1.87702247068463,-1.15758829005009));
#11314=CARTESIAN_POINT('Ctrl Pts',(97.8767183642239,1.91535456988331,-1.09300989014078));
#11315=CARTESIAN_POINT('Ctrl Pts',(97.8807854450125,1.95032721951919,-1.02656696654556));
#11316=CARTESIAN_POINT('Ctrl Pts',(97.884847767365,1.98525895157162,-0.960201780379423));
#11317=CARTESIAN_POINT('Ctrl Pts',(97.8889100897175,2.01683882182788,-0.891976824994816));
#11318=CARTESIAN_POINT('Ctrl Pts',(97.8929724120701,2.04487063161971,-0.822265224814485));
#11319=CARTESIAN_POINT('Ctrl Pts',(97.8970321561931,2.07288465049487,-0.752597868415728));
#11320=CARTESIAN_POINT('Ctrl Pts',(97.9010919003162,2.09735489976669,-0.681446181414142));
#11321=CARTESIAN_POINT('Ctrl Pts',(97.9051516444392,2.11813245303143,-0.609205147232894));
#11322=CARTESIAN_POINT('Ctrl Pts',(97.9092101238781,2.13890353371035,-0.536986617448005));
#11323=CARTESIAN_POINT('Ctrl Pts',(97.9132686033171,2.15598407044871,-0.463679872810791));
#11324=CARTESIAN_POINT('Ctrl Pts',(97.9173270827559,2.16927486445895,-0.389695473962193));
#11325=CARTESIAN_POINT('Ctrl Pts',(97.9213856093723,2.18256581296693,-0.315710215087998));
#11326=CARTESIAN_POINT('Ctrl Pts',(97.9254441359887,2.1920668486204,-0.241047756616787));
#11327=CARTESIAN_POINT('Ctrl Pts',(97.929502662605,2.1977301000837,-0.166127683382604));
#11328=CARTESIAN_POINT('Ctrl Pts',(97.9335653395744,2.20339914293265,-0.0911309949673516));
#11329=CARTESIAN_POINT('Ctrl Pts',(97.9376280165438,2.20522252828817,-0.0158766428677534));
#11330=CARTESIAN_POINT('Ctrl Pts',(97.9416906935132,2.20320445441821,0.0592126002784699));
#11331=CARTESIAN_POINT('Ctrl Pts',(97.9457554924746,2.20118532648051,0.134341063569739));
#11332=CARTESIAN_POINT('Ctrl Pts',(97.9498202914361,2.19532078094752,0.209303769722548));
#11333=CARTESIAN_POINT('Ctrl Pts',(97.9538850903976,2.18566699386736,0.283682554836975));
#11334=CARTESIAN_POINT('Ctrl Pts',(97.9579571506244,2.17599596147924,0.358194208539071));
#11335=CARTESIAN_POINT('Ctrl Pts',(97.9620292108512,2.16252225269991,0.432119387265153));
#11336=CARTESIAN_POINT('Ctrl Pts',(97.9661012710781,2.14535322029897,0.505050057076367));
#11337=CARTESIAN_POINT('Ctrl Pts',(97.9692394220212,2.13212183072731,0.561254395297625));
#11338=CARTESIAN_POINT('Ctrl Pts',(97.9723775729642,2.11669681584981,0.616868281523678));
#11339=CARTESIAN_POINT('Ctrl Pts',(97.9755157239073,2.09914703400378,0.671712534967985));
#11340=CARTESIAN_POINT('Ctrl Pts',(97.9795887888431,2.07636884316304,0.742895919606782));
#11341=CARTESIAN_POINT('Ctrl Pts',(97.9836618537789,2.04992181246092,0.813056629302231));
#11342=CARTESIAN_POINT('Ctrl Pts',(97.9877349187148,2.01991664467316,0.881789514891353));
#11343=CARTESIAN_POINT('Ctrl Pts',(97.9918019995195,1.98995556036083,0.950421418393163));
#11344=CARTESIAN_POINT('Ctrl Pts',(97.9958690803242,1.95644690732366,1.01762922873601));
#11345=CARTESIAN_POINT('Ctrl Pts',(97.9999361611289,1.9195509141684,1.0830236783724));
#11346=CARTESIAN_POINT('Ctrl Pts',(98.0039984834971,1.88269808888879,1.14834161727606));
#11347=CARTESIAN_POINT('Ctrl Pts',(98.0080608058654,1.8424660308018,1.21184999687947));
#11348=CARTESIAN_POINT('Ctrl Pts',(98.0121231282336,1.79906204435868,1.27318174686412));
#11349=CARTESIAN_POINT('Ctrl Pts',(98.0161828723722,1.75568560507644,1.33447457149368));
#11350=CARTESIAN_POINT('Ctrl Pts',(98.0202426165107,1.7091415073808,1.39359311907142));
#11351=CARTESIAN_POINT('Ctrl Pts',(98.0243023606492,1.65968104116966,1.45019820768818));
#11352=CARTESIAN_POINT('Ctrl Pts',(98.0283608401034,1.61023598279663,1.50678566278652));
#11353=CARTESIAN_POINT('Ctrl Pts',(98.0324193195575,1.55787667365686,1.56086085420544));
#11354=CARTESIAN_POINT('Ctrl Pts',(98.0364777990116,1.50289443965292,1.61211795575272));
#11355=CARTESIAN_POINT('Ctrl Pts',(98.0405363256429,1.44791156651626,1.66337565313048));
#11356=CARTESIAN_POINT('Ctrl Pts',(98.0445948522743,1.39030605843857,1.71181487132733));
#11357=CARTESIAN_POINT('Ctrl Pts',(98.0486533789056,1.33040463637171,1.75716803508392));
#11358=CARTESIAN_POINT('Ctrl Pts',(98.0527160558894,1.27044195758822,1.80256757813844));
#11359=CARTESIAN_POINT('Ctrl Pts',(98.0567787328732,1.20817905778068,1.8448744757943));
#11360=CARTESIAN_POINT('Ctrl Pts',(98.060841409857,1.14397354961176,1.88386318977485));
#11361=CARTESIAN_POINT('Ctrl Pts',(98.0649062088326,1.07973450602679,1.92287226809457));
#11362=CARTESIAN_POINT('Ctrl Pts',(98.0689710078082,1.01355125415047,1.95855948455254));
#11363=CARTESIAN_POINT('Ctrl Pts',(98.0730358067838,0.945805695656618,1.99074548500392));
#11364=CARTESIAN_POINT('Ctrl Pts',(98.0771078670242,0.877939118032233,2.02298898179715));
#11365=CARTESIAN_POINT('Ctrl Pts',(98.0811799272646,0.808505101086245,2.05171858690034));
#11366=CARTESIAN_POINT('Ctrl Pts',(98.085251987505,0.737904760917371,2.07680344852744));
#11367=CARTESIAN_POINT('Ctrl Pts',(98.0883901383121,0.683496303919378,2.09613520545488));
#11368=CARTESIAN_POINT('Ctrl Pts',(98.0915282891192,0.628395567240788,2.11330331419059));
#11369=CARTESIAN_POINT('Ctrl Pts',(98.0946664399263,0.572790460130373,2.1282685659436));
#11370=CARTESIAN_POINT('Ctrl Pts',(98.0998967677324,0.480113926796354,2.15321101682651));
#11371=CARTESIAN_POINT('Ctrl Pts',(98.1051270955386,0.385747273566499,2.17211193581593));
#11372=CARTESIAN_POINT('Ctrl Pts',(98.1103574233447,0.290381856862663,2.18478703245991));
#11373=CARTESIAN_POINT('Ctrl Pts',(98.1155877511508,0.195016440158827,2.19746212910389));
#11374=CARTESIAN_POINT('Ctrl Pts',(98.120818078957,0.0986519424616607,2.20391122409829));
#11375=CARTESIAN_POINT('Ctrl Pts',(98.1260484067631,0.00200370534589378,
2.2039990891933));
#11376=CARTESIAN_POINT('',(98.8760484068365,-0.000689329991712772,2.20399989220149));
#11377=CARTESIAN_POINT('Ctrl Pts',(98.1260484068025,0.00200370461793977,
2.20399908919396));
#11378=CARTESIAN_POINT('Ctrl Pts',(98.1300685156377,-0.0722815880720076,
2.20406662360663));
#11379=CARTESIAN_POINT('Ctrl Pts',(98.1340886244729,-0.146655895447738,
2.20037424384966));
#11380=CARTESIAN_POINT('Ctrl Pts',(98.1381087333081,-0.220704688647699,
2.1929216676409));
#11381=CARTESIAN_POINT('Ctrl Pts',(98.1421265750994,-0.294711723807198,
2.1854732941337));
#11382=CARTESIAN_POINT('Ctrl Pts',(98.1461444168907,-0.36839312409481,2.17426897856647));
#11383=CARTESIAN_POINT('Ctrl Pts',(98.1501622586819,-0.441337082029862,
2.15936045625212));
#11384=CARTESIAN_POINT('Ctrl Pts',(98.1541791980949,-0.514264657277744,
2.14445528228442));
#11385=CARTESIAN_POINT('Ctrl Pts',(98.1581961375079,-0.58645464080003,2.12584765095944));
#11386=CARTESIAN_POINT('Ctrl Pts',(98.1622130769208,-0.657504793743489,
2.103640522096));
#11387=CARTESIAN_POINT('Ctrl Pts',(98.1662304772368,-0.728563098969988,
2.0814308451902));
#11388=CARTESIAN_POINT('Ctrl Pts',(98.1702478775528,-0.798480849007217,
2.05562099963288));
#11389=CARTESIAN_POINT('Ctrl Pts',(98.1742652778687,-0.866872050191152,
2.02636345421975));
#11390=CARTESIAN_POINT('Ctrl Pts',(98.1782870082842,-0.935336965888348,
1.99707437396467));
#11391=CARTESIAN_POINT('Ctrl Pts',(98.1823087386997,-1.00227160142837,1.9643303742205));
#11392=CARTESIAN_POINT('Ctrl Pts',(98.1863304691151,-1.06731191668464,1.92833121441908));
#11393=CARTESIAN_POINT('Ctrl Pts',(98.1903547887712,-1.13239410571263,1.89230887790651));
#11394=CARTESIAN_POINT('Ctrl Pts',(98.1943791084272,-1.19557913579793,1.85302747234195));
#11395=CARTESIAN_POINT('Ctrl Pts',(98.1984034280833,-1.25653177887033,1.8107302086973));
#11396=CARTESIAN_POINT('Ctrl Pts',(98.20243433856,-1.31758424700099,1.76836367280136));
#11397=CARTESIAN_POINT('Ctrl Pts',(98.2064652490368,-1.3763966527891,1.72297172740696));
#11398=CARTESIAN_POINT('Ctrl Pts',(98.2104961595136,-1.4326674162586,1.6748373277399));
#11399=CARTESIAN_POINT('Ctrl Pts',(98.2116031583243,-1.44812091456723,1.66161829856775));
#11400=CARTESIAN_POINT('Ctrl Pts',(98.2127101571349,-1.46338294330759,1.64819263968996));
#11401=CARTESIAN_POINT('Ctrl Pts',(98.2138171559455,-1.47844777324369,1.6345666648353));
#11402=CARTESIAN_POINT('Ctrl Pts',(98.2178902207403,-1.53387694612193,1.58443158073162));
#11403=CARTESIAN_POINT('Ctrl Pts',(98.221963285535,-1.5868599519597,1.53137716195861));
#11404=CARTESIAN_POINT('Ctrl Pts',(98.2260363503298,-1.63707348818888,1.47567150621982));
#11405=CARTESIAN_POINT('Ctrl Pts',(98.2301034309937,-1.68721325088763,1.42004769301192));
#11406=CARTESIAN_POINT('Ctrl Pts',(98.2341705116576,-1.73459130536596,1.36178072807496));
#11407=CARTESIAN_POINT('Ctrl Pts',(98.2382375923216,-1.77891926122074,1.30117726004487));
#11408=CARTESIAN_POINT('Ctrl Pts',(98.2422999145501,-1.82319535390158,1.24064469734175));
#11409=CARTESIAN_POINT('Ctrl Pts',(98.2463622367787,-1.86442815744766,1.17778144618194));
#11410=CARTESIAN_POINT('Ctrl Pts',(98.2504245590073,-1.90236893434033,1.11292786722987));
#11411=CARTESIAN_POINT('Ctrl Pts',(98.2544843030069,-1.94028563140743,1.0481154488179));
#11412=CARTESIAN_POINT('Ctrl Pts',(98.2585440470065,-1.97491420741665,0.981315620368102));
#11413=CARTESIAN_POINT('Ctrl Pts',(98.2626037910061,-2.00604948532256,0.912897290190472));
#11414=CARTESIAN_POINT('Ctrl Pts',(98.2666622703222,-2.03717506402784,0.844500273556684));
#11415=CARTESIAN_POINT('Ctrl Pts',(98.2707207496383,-2.06480930761938,0.774486190542105));
#11416=CARTESIAN_POINT('Ctrl Pts',(98.2747792289545,-2.08879394854574,0.70324664273547));
#11417=CARTESIAN_POINT('Ctrl Pts',(98.2788377554489,-2.11277886828451,0.632006266795926));
#11418=CARTESIAN_POINT('Ctrl Pts',(98.2828962819433,-2.13311395047349,0.559540850854564));
#11419=CARTESIAN_POINT('Ctrl Pts',(98.2869548084377,-2.14969037951925,0.486258441780054));
#11420=CARTESIAN_POINT('Ctrl Pts',(98.2910174852873,-2.16628376005417,0.412901092200628));
#11421=CARTESIAN_POINT('Ctrl Pts',(98.2950801621368,-2.17911070622868,0.338725547815187));
#11422=CARTESIAN_POINT('Ctrl Pts',(98.2991428389864,-2.18811344346597,0.26415063604598));
#11423=CARTESIAN_POINT('Ctrl Pts',(98.3032076378291,-2.19712088295916,0.189536772754672));
#11424=CARTESIAN_POINT('Ctrl Pts',(98.3072724366717,-2.20230010289387,0.114523603452549));
#11425=CARTESIAN_POINT('Ctrl Pts',(98.3113372355144,-2.20364542091123,0.0395330102187932));
#11426=CARTESIAN_POINT('Ctrl Pts',(98.3154092956254,-2.20499314217548,-0.0355915445818049));
#11427=CARTESIAN_POINT('Ctrl Pts',(98.3194813557364,-2.20249329748571,-0.110692964854589));
#11428=CARTESIAN_POINT('Ctrl Pts',(98.3235534158474,-2.19619231302927,-0.185351892871758));
#11429=CARTESIAN_POINT('Ctrl Pts',(98.3266915678865,-2.19133643009012,-0.242888142535564));
#11430=CARTESIAN_POINT('Ctrl Pts',(98.3298297199256,-2.18422409221878,-0.300161630191771));
#11431=CARTESIAN_POINT('Ctrl Pts',(98.3329678719647,-2.17489716874867,-0.35698502121098));
#11432=CARTESIAN_POINT('Ctrl Pts',(98.3370409369447,-2.16279158403393,-0.430737140649556));
#11433=CARTESIAN_POINT('Ctrl Pts',(98.3411140019247,-2.14690693162874,-0.504015026224418));
#11434=CARTESIAN_POINT('Ctrl Pts',(98.3451870669046,-2.12729337414513,-0.576401683132722));
#11435=CARTESIAN_POINT('Ctrl Pts',(98.3492541477523,-2.10770863282881,-0.648681989828063));
#11436=CARTESIAN_POINT('Ctrl Pts',(98.3533212286001,-2.08440598731108,-0.720073210512294));
#11437=CARTESIAN_POINT('Ctrl Pts',(98.3573883094478,-2.05748691816683,-0.790166806169656));
#11438=CARTESIAN_POINT('Ctrl Pts',(98.3614506318572,-2.03059934402735,-0.860178393117225));
#11439=CARTESIAN_POINT('Ctrl Pts',(98.3655129542665,-2.00010392295595,-0.928894927886572));
#11440=CARTESIAN_POINT('Ctrl Pts',(98.3695752766759,-1.96615195503874,-0.995922933613512));
#11441=CARTESIAN_POINT('Ctrl Pts',(98.3736350208544,-1.93222153538971,-1.06290839872994));
#11442=CARTESIAN_POINT('Ctrl Pts',(98.3776947650329,-1.89483913738575,-1.12820703653688));
#11443=CARTESIAN_POINT('Ctrl Pts',(98.3817545092114,-1.85420365720231,-1.19144651479518));
#11444=CARTESIAN_POINT('Ctrl Pts',(98.3858129887042,-1.81358083572474,-1.25466629278289));
#11445=CARTESIAN_POINT('Ctrl Pts',(98.3898714681971,-1.76970720206007,-1.3158277834051));
#11446=CARTESIAN_POINT('Ctrl Pts',(98.39392994769,-1.72282614248017,-1.37458578589584));
#11447=CARTESIAN_POINT('Ctrl Pts',(98.3979884743588,-1.67594453795309,-1.4333444713918));
#11448=CARTESIAN_POINT('Ctrl Pts',(98.4020470010275,-1.62605573728272,-1.48969924117991));
#11449=CARTESIAN_POINT('Ctrl Pts',(98.4061055276963,-1.57344374299025,-1.54333754818731));
#11450=CARTESIAN_POINT('Ctrl Pts',(98.4101682047153,-1.5207779463644,-1.597030707061));
#11451=CARTESIAN_POINT('Ctrl Pts',(98.4142308817344,-1.46538373010052,-1.64800151418336));
#11452=CARTESIAN_POINT('Ctrl Pts',(98.4182935587534,-1.40758181278408,-1.69597448103428));
#11453=CARTESIAN_POINT('Ctrl Pts',(98.4223583577632,-1.34974970475159,-1.7439725048087));
#11454=CARTESIAN_POINT('Ctrl Pts',(98.4264231567729,-1.28950777421597,-1.78896928415809));
#11455=CARTESIAN_POINT('Ctrl Pts',(98.4304879557826,-1.22720753181922,-1.83073145869245));
#11456=CARTESIAN_POINT('Ctrl Pts',(98.4345600160548,-1.16479599771715,-1.87256823620495));
#11457=CARTESIAN_POINT('Ctrl Pts',(98.438632076327,-1.10031921768597,-1.91115862178277));
#11458=CARTESIAN_POINT('Ctrl Pts',(98.4427041365992,-1.03415481414691,-1.94631441971146));
#11459=CARTESIAN_POINT('Ctrl Pts',(98.4458422870607,-0.983164936879575,
-1.97340738399038));
#11460=CARTESIAN_POINT('Ctrl Pts',(98.4489804375223,-0.931173316964451,
-1.99846144315086));
#11461=CARTESIAN_POINT('Ctrl Pts',(98.4521185879838,-0.878360093452682,
-2.02141028646581));
#11462=CARTESIAN_POINT('Ctrl Pts',(98.4561916533852,-0.809812802282947,
-2.0511960283713));
#11463=CARTESIAN_POINT('Ctrl Pts',(98.4602647187866,-0.739616525338188,
-2.07754853526234));
#11464=CARTESIAN_POINT('Ctrl Pts',(98.4643377841881,-0.668148923568016,
-2.10028403220491));
#11465=CARTESIAN_POINT('Ctrl Pts',(98.4684048654609,-0.5967863216628,-2.12298612626212));
#11466=CARTESIAN_POINT('Ctrl Pts',(98.4724719467337,-0.524156554541037,
-2.14208161747396));
#11467=CARTESIAN_POINT('Ctrl Pts',(98.4765390280066,-0.450657981229541,
-2.15743444487987));
#11468=CARTESIAN_POINT('Ctrl Pts',(98.4806013508446,-0.377245400341508,
-2.17276930966724));
#11469=CARTESIAN_POINT('Ctrl Pts',(98.4846636736825,-0.302966497826674,
-2.1843701133278));
#11470=CARTESIAN_POINT('Ctrl Pts',(98.4887259965205,-0.228233966287282,
-2.19215082889677));
#11471=CARTESIAN_POINT('Ctrl Pts',(98.4927857411294,-0.153548865143528,
-2.19992660628941));
#11472=CARTESIAN_POINT('Ctrl Pts',(98.4968454857384,-0.078411179979942,
-2.20388705741142));
#11473=CARTESIAN_POINT('Ctrl Pts',(98.5009052303474,-0.00324161999589336,
-2.20399761612843));
#11474=CARTESIAN_POINT('Ctrl Pts',(98.504963710272,0.0719045233018444,-2.20410814040439));
#11475=CARTESIAN_POINT('Ctrl Pts',(98.5090221901966,0.147082044556721,-2.20037115275537));
#11476=CARTESIAN_POINT('Ctrl Pts',(98.5130806701213,0.221868932772679,-2.19280418110471));
#11477=CARTESIAN_POINT('Ctrl Pts',(98.5171391972225,0.29665669032631,-2.18523712149407));
#11478=CARTESIAN_POINT('Ctrl Pts',(98.5211977243237,0.371053330970389,-2.17384003933285));
#11479=CARTESIAN_POINT('Ctrl Pts',(98.5252562514249,0.444642282234361,-2.15868229270762));
#11480=CARTESIAN_POINT('Ctrl Pts',(98.5293189288743,0.51830648734473,-2.14350904540305));
#11481=CARTESIAN_POINT('Ctrl Pts',(98.5333816063238,0.591160884992382,-2.1245675504363));
#11482=CARTESIAN_POINT('Ctrl Pts',(98.5374442837732,0.66280015669062,-2.10197810461738));
#11483=CARTESIAN_POINT('Ctrl Pts',(98.5415090832129,0.7344768465289,-2.07937686003186));
#11484=CARTESIAN_POINT('Ctrl Pts',(98.5455738826526,0.804936698691908,-2.0531240370874));
#11485=CARTESIAN_POINT('Ctrl Pts',(98.5496386820922,0.873793119374038,-2.02338863902479));
#11486=CARTESIAN_POINT('Ctrl Pts',(98.5537107427888,0.942772543457405,-1.99360012238496));
#11487=CARTESIAN_POINT('Ctrl Pts',(98.5577828034853,1.01014238607789,-1.96031681608829));
#11488=CARTESIAN_POINT('Ctrl Pts',(98.5618548641818,1.0755398661799,-1.92375414132308));
#11489=CARTESIAN_POINT('Ctrl Pts',(98.5649930107888,1.12593864350324,-1.89557699900869));
#11490=CARTESIAN_POINT('Ctrl Pts',(98.5681311573959,1.17516650040913,-1.86545318199277));
#11491=CARTESIAN_POINT('Ctrl Pts',(98.5712693040029,1.2230701006524,-1.83349816713574));
#11492=CARTESIAN_POINT('Ctrl Pts',(98.5753423677599,1.28524514930769,-1.792023109031));
#11493=CARTESIAN_POINT('Ctrl Pts',(98.5794154315169,1.34542804035084,-1.74730189288413));
#11494=CARTESIAN_POINT('Ctrl Pts',(98.5834884952739,1.40325968770601,-1.69955236720121));
#11495=CARTESIAN_POINT('Ctrl Pts',(98.5875555749001,1.4610063690102,-1.65187299495191));
#11496=CARTESIAN_POINT('Ctrl Pts',(98.5916226545262,1.51640829997285,-1.60117444807728));
#11497=CARTESIAN_POINT('Ctrl Pts',(98.5956897341524,1.56913528317269,-1.54771782412124));
#11498=CARTESIAN_POINT('Ctrl Pts',(98.5997520553481,1.62180057648512,-1.49432374372283));
#11499=CARTESIAN_POINT('Ctrl Pts',(98.6038143765438,1.67179680634006,-1.43817833560501));
#11500=CARTESIAN_POINT('Ctrl Pts',(98.6078766977395,1.71882806235913,-1.37958185405824));
#11501=CARTESIAN_POINT('Ctrl Pts',(98.6119364407097,1.76582946914223,-1.32102256182668));
#11502=CARTESIAN_POINT('Ctrl Pts',(98.6159961836799,1.8098693381602,-1.26001565453461));
#11503=CARTESIAN_POINT('Ctrl Pts',(98.6200559266501,1.85069066799873,-1.19689600692058));
#11504=CARTESIAN_POINT('Ctrl Pts',(98.6241144049417,1.89149928130278,-1.13379602214405));
#11505=CARTESIAN_POINT('Ctrl Pts',(98.6281728832333,1.92909108698606,-1.06858500444347));
#11506=CARTESIAN_POINT('Ctrl Pts',(98.6322313615249,1.96325216304356,-1.00162714834652));
#11507=CARTESIAN_POINT('Ctrl Pts',(98.6362898870011,1.99741363626414,-0.934668513784985));
#11508=CARTESIAN_POINT('Ctrl Pts',(98.6403484124774,2.02814408527399,-0.865963426624388));
#11509=CARTESIAN_POINT('Ctrl Pts',(98.6444069379536,2.05527609772403,-0.795899592991663));
#11510=CARTESIAN_POINT('Ctrl Pts',(98.6484696138018,2.08243585619754,-0.725764109945683));
#11511=CARTESIAN_POINT('Ctrl Pts',(98.6525322896499,2.10598965681717,-0.654267551915746));
#11512=CARTESIAN_POINT('Ctrl Pts',(98.6565949654981,2.12581899857559,-0.581815765767015));
#11513=CARTESIAN_POINT('Ctrl Pts',(98.6606597633471,2.14565869751758,-0.509326136887162));
#11514=CARTESIAN_POINT('Ctrl Pts',(98.6647245611961,2.16176996123382,-0.43588075312185));
#11515=CARTESIAN_POINT('Ctrl Pts',(98.6687893590451,2.17408537160911,-0.361896113484658));
#11516=CARTESIAN_POINT('Ctrl Pts',(98.6728614181864,2.18642278204383,-0.287779308826521));
#11517=CARTESIAN_POINT('Ctrl Pts',(98.6769334773277,2.19495074064123,-0.213121799223034));
#11518=CARTESIAN_POINT('Ctrl Pts',(98.6810055364689,2.19965374554041,-0.138345219397123));
#11519=CARTESIAN_POINT('Ctrl Pts',(98.6841436976533,2.20327814953667,-0.0807181191586382));
#11520=CARTESIAN_POINT('Ctrl Pts',(98.6872818588377,2.20463193494392,-0.02302042152449));
#11521=CARTESIAN_POINT('Ctrl Pts',(98.6904200200221,2.20372907897158,0.0345564248014581));
#11522=CARTESIAN_POINT('Ctrl Pts',(98.6944930856565,2.20255724890371,0.109286261901794));
#11523=CARTESIAN_POINT('Ctrl Pts',(98.6985661512908,2.19757764677268,0.184100536604629));
#11524=CARTESIAN_POINT('Ctrl Pts',(98.7026392169252,2.1887788129006,0.258579404047292));
#11525=CARTESIAN_POINT('Ctrl Pts',(98.7067062984189,2.17999290625919,0.332948847273765));
#11526=CARTESIAN_POINT('Ctrl Pts',(98.7107733799127,2.16739896396685,0.40698339138202));
#11527=CARTESIAN_POINT('Ctrl Pts',(98.7148404614064,2.15103752937728,0.48026403905611));
#11528=CARTESIAN_POINT('Ctrl Pts',(98.7189027844465,2.13469523753883,0.553458948942818));
#11529=CARTESIAN_POINT('Ctrl Pts',(98.7229651074865,2.11459431448589,0.625901251187874));
#11530=CARTESIAN_POINT('Ctrl Pts',(98.7270274305266,2.09082679201224,0.697179550620779));
#11531=CARTESIAN_POINT('Ctrl Pts',(98.7310871753261,2.0670743541073,0.768412611749784));
#11532=CARTESIAN_POINT('Ctrl Pts',(98.7351469201255,2.03966008528233,0.838482684259335));
#11533=CARTESIAN_POINT('Ctrl Pts',(98.739206664925,2.00872619729104,0.90699231767236));
#11534=CARTESIAN_POINT('Ctrl Pts',(98.7432651450284,1.97780194585806,0.975480608890158));
#11535=CARTESIAN_POINT('Ctrl Pts',(98.7473236251317,1.94336044854155,1.04240899128766));
#11536=CARTESIAN_POINT('Ctrl Pts',(98.7513821052351,1.90559190151686,1.10740033631625));
#11537=CARTESIAN_POINT('Ctrl Pts',(98.7554406325031,1.86782291557415,1.17239243662603));
#11538=CARTESIAN_POINT('Ctrl Pts',(98.7594991597712,1.82672704460385,1.23544704295642));
#11539=CARTESIAN_POINT('Ctrl Pts',(98.7635576870392,1.7825394460346,1.29621337878093));
#11540=CARTESIAN_POINT('Ctrl Pts',(98.767620364636,1.73830666036864,1.35704185544093));
#11541=CARTESIAN_POINT('Ctrl Pts',(98.7716830422329,1.69097611487498,1.41557700167304));
#11542=CARTESIAN_POINT('Ctrl Pts',(98.7757457198297,1.6408247153413,1.47149932161899));
#11543=CARTESIAN_POINT('Ctrl Pts',(98.7798105194062,1.59064712119879,1.52745085038681));
#11544=CARTESIAN_POINT('Ctrl Pts',(98.7838753189827,1.53764607582393,1.58078649619607));
#11545=CARTESIAN_POINT('Ctrl Pts',(98.7879401185593,1.48213511584823,1.63122392649494));
#11546=CARTESIAN_POINT('Ctrl Pts',(98.792012179374,1.42652499272933,1.68175145673308));
#11547=CARTESIAN_POINT('Ctrl Pts',(98.7960842401887,1.36839636919061,1.72937012721333));
#11548=CARTESIAN_POINT('Ctrl Pts',(98.8001563010034,1.3080952277046,1.77383845804979));
#11549=CARTESIAN_POINT('Ctrl Pts',(98.803294446016,1.26162398500473,1.80810810110852));
#11550=CARTESIAN_POINT('Ctrl Pts',(98.8064325910286,1.21386315119932,1.84050757261451));
#11551=CARTESIAN_POINT('Ctrl Pts',(98.8095707360412,1.16498120820677,1.87094489083059));
#11552=CARTESIAN_POINT('Ctrl Pts',(98.813757197885,1.09976994857186,1.91154998423045));
#11553=CARTESIAN_POINT('Ctrl Pts',(98.8179436597288,1.03232269390181,1.94881103154898));
#11554=CARTESIAN_POINT('Ctrl Pts',(98.8221301215726,0.963005805721677,1.98248223652732));
#11555=CARTESIAN_POINT('Ctrl Pts',(98.8263092907943,0.893809664342735,2.01609478782976));
#11556=CARTESIAN_POINT('Ctrl Pts',(98.8304884600159,0.82275075711108,2.04612973507325));
#11557=CARTESIAN_POINT('Ctrl Pts',(98.8346676292375,0.750222616012183,2.07238558825906));
#11558=CARTESIAN_POINT('Ctrl Pts',(98.8388389852493,0.677830070664218,2.0985923545377));
#11559=CARTESIAN_POINT('Ctrl Pts',(98.843010341261,0.603974171398295,2.12103393939962));
#11560=CARTESIAN_POINT('Ctrl Pts',(98.8471816972727,0.529069616147168,2.13955634215832));
#11561=CARTESIAN_POINT('Ctrl Pts',(98.8513484326716,0.454248032705071,2.15805822764328));
#11562=CARTESIAN_POINT('Ctrl Pts',(98.8555151680704,0.378380528606072,2.17264945329948));
#11563=CARTESIAN_POINT('Ctrl Pts',(98.8596819034693,0.301897734824081,2.18322553981674));
#11564=CARTESIAN_POINT('Ctrl Pts',(98.8638443463035,0.225493733501853,2.19379073086549));
#11565=CARTESIAN_POINT('Ctrl Pts',(98.8680067891378,0.148476140120422,2.20034895303591));
#11566=CARTESIAN_POINT('Ctrl Pts',(98.8721692319721,0.0712852104429588,
2.20284688954364));
#11567=CARTESIAN_POINT('Ctrl Pts',(98.8734622902489,0.0473059332520479,
2.20362287076546));
#11568=CARTESIAN_POINT('Ctrl Pts',(98.8747553485257,0.0233099826406988,
2.20400739829569));
#11569=CARTESIAN_POINT('Ctrl Pts',(98.8760484068025,-0.00068932936029577,
2.20399989220168));
#11570=CARTESIAN_POINT('',(99.6260484068026,-0.00167252030352725,2.20399936539824));
#11571=CARTESIAN_POINT('Ctrl Pts',(98.8760484068365,-0.000689329991730441,
2.20399989220149));
#11572=CARTESIAN_POINT('Ctrl Pts',(98.8804378272718,-0.0821574837625145,
2.2039744119635));
#11573=CARTESIAN_POINT('Ctrl Pts',(98.8848272477072,-0.163495403890133,
2.19942758819312));
#11574=CARTESIAN_POINT('Ctrl Pts',(98.8892166681425,-0.244213885737787,
2.19042817230167));
#11575=CARTESIAN_POINT('Ctrl Pts',(98.893604022686,-0.324894377228526,2.181432992008));
#11576=CARTESIAN_POINT('Ctrl Pts',(98.8979913772296,-0.404955679669053,
2.1679895597763));
#11577=CARTESIAN_POINT('Ctrl Pts',(98.9023787317731,-0.483923865789736,
2.15021712673839));
#11578=CARTESIAN_POINT('Ctrl Pts',(98.9067839458555,-0.563213506530593,
2.13237234772178));
#11579=CARTESIAN_POINT('Ctrl Pts',(98.9111891599379,-0.641400782654518,
2.11016339615855));
#11580=CARTESIAN_POINT('Ctrl Pts',(98.9155943740203,-0.718025682717486,
2.08375985155634));
#11581=CARTESIAN_POINT('Ctrl Pts',(98.9199700667003,-0.794137083444975,
2.05753324947015));
#11582=CARTESIAN_POINT('Ctrl Pts',(98.9243457593804,-0.868706716711618,
2.02716833620499));
#11583=CARTESIAN_POINT('Ctrl Pts',(98.9287214520604,-0.941307554494785,
1.99287633531312));
#11584=CARTESIAN_POINT('Ctrl Pts',(98.9327945073845,-1.00888707858082,1.96095608244838));
#11585=CARTESIAN_POINT('Ctrl Pts',(98.9368675627086,-1.07497143834343,1.9255328876901));
#11586=CARTESIAN_POINT('Ctrl Pts',(98.9409406180326,-1.13917351153671,1.88676964958977));
#11587=CARTESIAN_POINT('Ctrl Pts',(98.9450076892201,-1.20328125898522,1.84806336247438));
#11588=CARTESIAN_POINT('Ctrl Pts',(98.9490747604075,-1.26551180507766,1.80602701953534));
#11589=CARTESIAN_POINT('Ctrl Pts',(98.953141831595,-1.32550026940888,1.76087053351375));
#11590=CARTESIAN_POINT('Ctrl Pts',(98.957204144383,-1.38541854832619,1.71576687976078));
#11591=CARTESIAN_POINT('Ctrl Pts',(98.961266457171,-1.44309957762212,1.66755062136221));
#11592=CARTESIAN_POINT('Ctrl Pts',(98.965328769959,-1.49820665835499,1.61647542785554));
#11593=CARTESIAN_POINT('Ctrl Pts',(98.9693885045446,-1.55327876462395,1.56543264992032));
#11594=CARTESIAN_POINT('Ctrl Pts',(98.9734482391301,-1.60577981471814,1.51153486122198));
#11595=CARTESIAN_POINT('Ctrl Pts',(98.9775079737156,-1.65540652773743,1.45507567773099));
#11596=CARTESIAN_POINT('Ctrl Pts',(98.9815664436573,-1.70501778158834,1.39863408178452));
#11597=CARTESIAN_POINT('Ctrl Pts',(98.9856249135989,-1.7517561610921,1.33963303362135));
#11598=CARTESIAN_POINT('Ctrl Pts',(98.9896833835405,-1.79535670531577,1.27840146303018));
#11599=CARTESIAN_POINT('Ctrl Pts',(98.9937419007131,-1.8389577569464,1.2171691798487));
#11600=CARTESIAN_POINT('Ctrl Pts',(98.9978004178857,-1.87942062530542,1.15370671267549));
#11601=CARTESIAN_POINT('Ctrl Pts',(99.0018589350582,-1.91652291347563,1.08837306201638));
#11602=CARTESIAN_POINT('Ctrl Pts',(99.0059216027317,-1.95366314483411,1.02297259696035));
#11603=CARTESIAN_POINT('Ctrl Pts',(99.0099842704053,-1.98743569671596,0.955697543191284));
#11604=CARTESIAN_POINT('Ctrl Pts',(99.0140469380788,-2.01766389872753,0.886932010794298));
#11605=CARTESIAN_POINT('Ctrl Pts',(99.0181117278117,-2.04790788988244,0.818130559990831));
#11606=CARTESIAN_POINT('Ctrl Pts',(99.0221765175447,-2.07460367475865,0.747837526978033));
#11607=CARTESIAN_POINT('Ctrl Pts',(99.0262413072777,-2.09762355455813,0.676455041642015));
#11608=CARTESIAN_POINT('Ctrl Pts',(99.030313358491,-2.12068455786344,0.604945036176564));
#11609=CARTESIAN_POINT('Ctrl Pts',(99.0343854097043,-2.14005641622013,0.532342152943204));
#11610=CARTESIAN_POINT('Ctrl Pts',(99.0384574609176,-2.15566203483824,0.459061206765558));
#11611=CARTESIAN_POINT('Ctrl Pts',(99.0415956966382,-2.16768892429142,0.402585275867206));
#11612=CARTESIAN_POINT('Ctrl Pts',(99.0447339323588,-2.17747992202309,0.345706889448446));
#11613=CARTESIAN_POINT('Ctrl Pts',(99.0478721680795,-2.18502081063902,0.288617492668778));
#11614=CARTESIAN_POINT('Ctrl Pts',(99.0519452411864,-2.1948080265649,0.214521947459351));
#11615=CARTESIAN_POINT('Ctrl Pts',(99.0560183142934,-2.2008408984806,0.139785114427793));
#11616=CARTESIAN_POINT('Ctrl Pts',(99.0600913874004,-2.20304659179242,0.0648206324546741));
#11617=CARTESIAN_POINT('Ctrl Pts',(99.0641584763078,-2.20524904447765,-0.0100337109549575));
#11618=CARTESIAN_POINT('Ctrl Pts',(99.0682255652152,-2.20363546844268,-0.0851145659680157));
#11619=CARTESIAN_POINT('Ctrl Pts',(99.0722926541226,-2.19818459535836,-0.160001514771584));
#11620=CARTESIAN_POINT('Ctrl Pts',(99.0763549844544,-2.19274009990489,-0.234800844343007));
#11621=CARTESIAN_POINT('Ctrl Pts',(99.0804173147862,-2.18346726192895,-0.309406244646234));
#11622=CARTESIAN_POINT('Ctrl Pts',(99.084479645118,-2.17039685972843,-0.383397276047933));
#11623=CARTESIAN_POINT('Ctrl Pts',(99.0885393971312,-2.15733475317543,-0.45734134611617));
#11624=CARTESIAN_POINT('Ctrl Pts',(99.0925991491445,-2.14047994817327,-0.530671352076355));
#11625=CARTESIAN_POINT('Ctrl Pts',(99.0966589011577,-2.11991490433368,-0.602973298234623));
#11626=CARTESIAN_POINT('Ctrl Pts',(99.1007173883874,-2.09935626737051,-0.675252719294549));
#11627=CARTESIAN_POINT('Ctrl Pts',(99.1047758756171,-2.07508981708984,-0.746504257519102));
#11628=CARTESIAN_POINT('Ctrl Pts',(99.1088343628468,-2.04724845670253,-0.816326991180082));
#11629=CARTESIAN_POINT('Ctrl Pts',(99.1128928971441,-2.0194067734298,-0.886150534598268));
#11630=CARTESIAN_POINT('Ctrl Pts',(99.1169514314414,-1.98799027623994,-0.954544797714794));
#11631=CARTESIAN_POINT('Ctrl Pts',(99.1210099657387,-1.95318020468243,-1.02112834062947));
#11632=CARTESIAN_POINT('Ctrl Pts',(99.1250726501671,-1.91833453742703,-1.08777996980689));
#11633=CARTESIAN_POINT('Ctrl Pts',(99.1291353345954,-1.88008858778585,-1.15261675720722));
#11634=CARTESIAN_POINT('Ctrl Pts',(99.1331980190238,-1.83866947535711,-1.21528209087027));
#11635=CARTESIAN_POINT('Ctrl Pts',(99.137262825333,-1.79722873033025,-1.27798015372281));
#11636=CARTESIAN_POINT('Ctrl Pts',(99.1413276316422,-1.75261180574522,-1.33850411967357));
#11637=CARTESIAN_POINT('Ctrl Pts',(99.1453924379514,-1.70508750065945,-1.39652877345758));
#11638=CARTESIAN_POINT('Ctrl Pts',(99.1494645052614,-1.65747830247203,-1.45465707721232));
#11639=CARTESIAN_POINT('Ctrl Pts',(99.1535365725714,-1.60695167173138,-1.51027679728771));
#11640=CARTESIAN_POINT('Ctrl Pts',(99.1576086398813,-1.55381448750771,-1.56309837771369));
#11641=CARTESIAN_POINT('Ctrl Pts',(99.1607467212871,-1.51286506376914,-1.60380458582399));
#11642=CARTESIAN_POINT('Ctrl Pts',(99.1638848026929,-1.47036607962651,-1.64284976010869));
#11643=CARTESIAN_POINT('Ctrl Pts',(99.1670228840986,-1.42647071631425,-1.68011823854689));
#11644=CARTESIAN_POINT('Ctrl Pts',(99.1710959695303,-1.36949655226152,-1.72849101061917));
#11645=CARTESIAN_POINT('Ctrl Pts',(99.1751690549619,-1.30994919752869,-1.7740557142029));
#11646=CARTESIAN_POINT('Ctrl Pts',(99.1792421403935,-1.24813685368431,-1.81652701451837));
#11647=CARTESIAN_POINT('Ctrl Pts',(99.1833092418649,-1.18641532124411,-1.85893591826094));
#11648=CARTESIAN_POINT('Ctrl Pts',(99.1873763433363,-1.12243579659121,-1.89826017360842));
#11649=CARTESIAN_POINT('Ctrl Pts',(99.1914434448077,-1.05654011831091,-1.93425411422583));
#11650=CARTESIAN_POINT('Ctrl Pts',(99.195505787998,-0.990721534286376,-1.97020594394712));
#11651=CARTESIAN_POINT('Ctrl Pts',(99.1995681311883,-0.92299166748019,-2.0028349722339));
#11652=CARTESIAN_POINT('Ctrl Pts',(99.2036304743786,-0.853720574479981,
-2.03193926599925));
#11653=CARTESIAN_POINT('Ctrl Pts',(99.2076902394239,-0.784493444018035,
-2.0610250888762));
#11654=CARTESIAN_POINT('Ctrl Pts',(99.2117500044693,-0.713727467424388,
-2.08659043175383));
#11655=CARTESIAN_POINT('Ctrl Pts',(99.2158097695146,-0.641815286916337,
-2.10848029098697));
#11656=CARTESIAN_POINT('Ctrl Pts',(99.21986826993,-0.569925507284941,-2.13036333145821));
#11657=CARTESIAN_POINT('Ctrl Pts',(99.2239267703454,-0.496890689104043,
-2.14857302253901));
#11658=CARTESIAN_POINT('Ctrl Pts',(99.2279852707609,-0.42311981713259,-2.16300384196369));
#11659=CARTESIAN_POINT('Ctrl Pts',(99.2320438183777,-0.349348087186561,
-2.17743482922259));
#11660=CARTESIAN_POINT('Ctrl Pts',(99.2361023659946,-0.27484075537111,-2.18808676766113));
#11661=CARTESIAN_POINT('Ctrl Pts',(99.2401609136114,-0.200016621497414,
-2.19490531712071));
#11662=CARTESIAN_POINT('Ctrl Pts',(99.2442236114712,-0.125115972977261,
-2.20173083918223));
#11663=CARTESIAN_POINT('Ctrl Pts',(99.248286309331,-0.0498983520112227,
-2.20471510082763));
#11664=CARTESIAN_POINT('Ctrl Pts',(99.2523490071908,0.0252134507354692,
-2.20385577611195));
#11665=CARTESIAN_POINT('Ctrl Pts',(99.2564138270146,0.100364484688543,-2.20299600256741));
#11666=CARTESIAN_POINT('Ctrl Pts',(99.2604786468384,0.175409113396773,-2.19828867479555));
#11667=CARTESIAN_POINT('Ctrl Pts',(99.2645434666621,0.249928352263751,-2.18978350955859));
#11668=CARTESIAN_POINT('Ctrl Pts',(99.2686155474668,0.324580704722417,-2.18126315155919));
#11669=CARTESIAN_POINT('Ctrl Pts',(99.2726876282714,0.398705321071872,-2.16893148390978));
#11670=CARTESIAN_POINT('Ctrl Pts',(99.276759709076,0.471892555701658,-2.15288955031914));
#11671=CARTESIAN_POINT('Ctrl Pts',(99.2798976727566,0.528290966040015,-2.14052756454605));
#11672=CARTESIAN_POINT('Ctrl Pts',(99.2830356364372,0.584132908470223,-2.12596336727211));
#11673=CARTESIAN_POINT('Ctrl Pts',(99.2861736001177,0.639238193960531,-2.10926303039286));
#11674=CARTESIAN_POINT('Ctrl Pts',(99.2902465884069,0.710763299193751,-2.08758646448652));
#11675=CARTESIAN_POINT('Ctrl Pts',(99.294319576696,0.781322536814027,-2.06222583963422));
#11676=CARTESIAN_POINT('Ctrl Pts',(99.2983925649851,0.850509108205028,-2.03328558172734));
#11677=CARTESIAN_POINT('Ctrl Pts',(99.3024595690473,0.91959402741384,-2.00438784421583));
#11678=CARTESIAN_POINT('Ctrl Pts',(99.3065265731094,0.987309847693555,-1.97192109835214));
#11679=CARTESIAN_POINT('Ctrl Pts',(99.3105935771715,1.0532648847763,-1.93603953536522));
#11680=CARTESIAN_POINT('Ctrl Pts',(99.3146558230158,1.11914275733449,-1.90019995224626));
#11681=CARTESIAN_POINT('Ctrl Pts',(99.3187180688601,1.18326352219853,-1.86095371655459));
#11682=CARTESIAN_POINT('Ctrl Pts',(99.3227803147044,1.24525696235485,-1.81850243269202));
#11683=CARTESIAN_POINT('Ctrl Pts',(99.3268399824895,1.30721105906302,-1.77607809006518));
#11684=CARTESIAN_POINT('Ctrl Pts',(99.3308996502746,1.36704011718689,-1.73045300470282));
#11685=CARTESIAN_POINT('Ctrl Pts',(99.3349593180597,1.42440112548946,-1.68187319192155));
#11686=CARTESIAN_POINT('Ctrl Pts',(99.3390177214372,1.48174426836611,-1.63330850961082));
#11687=CARTESIAN_POINT('Ctrl Pts',(99.3430761248147,1.53662052349016,-1.58179123541503));
#11688=CARTESIAN_POINT('Ctrl Pts',(99.3471345281923,1.58871961326095,-1.52760793086445));
#11689=CARTESIAN_POINT('Ctrl Pts',(99.3511929791303,1.64081931358217,-1.47342399133849));
#11690=CARTESIAN_POINT('Ctrl Pts',(99.3552514300683,1.69014145427682,-1.41657430485035));
#11691=CARTESIAN_POINT('Ctrl Pts',(99.3593098810064,1.73641345784783,-1.3573814141224));
#11692=CARTESIAN_POINT('Ctrl Pts',(99.3633724834128,1.78273279395095,-1.29812797383567));
#11693=CARTESIAN_POINT('Ctrl Pts',(99.3674350858192,1.82599546766183,-1.23652691983741));
#11694=CARTESIAN_POINT('Ctrl Pts',(99.3714976882256,1.86597045674903,-1.17293233161159));
#11695=CARTESIAN_POINT('Ctrl Pts',(99.375562413125,1.90596633063594,-1.10930451860528));
#11696=CARTESIAN_POINT('Ctrl Pts',(99.3796271380245,1.94267086609419,-1.04368151441209));
#11697=CARTESIAN_POINT('Ctrl Pts',(99.383691862924,1.97589884494488,-0.976442396941821));
#11698=CARTESIAN_POINT('Ctrl Pts',(99.3877638507495,2.00918619616578,-0.909083135366692));
#11699=CARTESIAN_POINT('Ctrl Pts',(99.3918358385749,2.03898439321521,-0.840102431539732));
#11700=CARTESIAN_POINT('Ctrl Pts',(99.3959078264004,2.06515641817133,-0.769899323603909));
#11701=CARTESIAN_POINT('Ctrl Pts',(99.3990466563126,2.08533072573685,-0.715784325092066));
#11702=CARTESIAN_POINT('Ctrl Pts',(99.4021854862248,2.1033513993086,-0.660943415302023));
#11703=CARTESIAN_POINT('Ctrl Pts',(99.4053243161369,2.11917631141579,-0.605564002508532));
#11704=CARTESIAN_POINT('Ctrl Pts',(99.4093974652079,2.13971174272361,-0.533700088220429));
#11705=CARTESIAN_POINT('Ctrl Pts',(99.4134706142789,2.15662713355787,-0.460651852012233));
#11706=CARTESIAN_POINT('Ctrl Pts',(99.41754376335,2.16978984641977,-0.386817815481237));
#11707=CARTESIAN_POINT('Ctrl Pts',(99.4216109278203,2.18293321955733,-0.313092261899616));
#11708=CARTESIAN_POINT('Ctrl Pts',(99.4256780922906,2.19233477865686,-0.238583666401459));
#11709=CARTESIAN_POINT('Ctrl Pts',(99.429745256761,2.19791190347919,-0.163704809167205));
#11710=CARTESIAN_POINT('Ctrl Pts',(99.4338076617085,2.20348250177602,-0.0889135775083088));
#11711=CARTESIAN_POINT('Ctrl Pts',(99.4378700666561,2.20523752226794,-0.0137534186954298));
#11712=CARTESIAN_POINT('Ctrl Pts',(99.4419324716036,2.20314582682219,0.0613552422859288));
#11713=CARTESIAN_POINT('Ctrl Pts',(99.445992297618,2.20105545924574,0.136416222098011));
#11714=CARTESIAN_POINT('Ctrl Pts',(99.4500521236324,2.19512323489591,0.211425292907891));
#11715=CARTESIAN_POINT('Ctrl Pts',(99.4541119496467,2.18537008339007,0.285960834072956));
#11716=CARTESIAN_POINT('Ctrl Pts',(99.4581705101639,2.17561997206034,0.360473141601971));
#11717=CARTESIAN_POINT('Ctrl Pts',(99.4622290706811,2.16205136022153,0.434511739454726));
#11718=CARTESIAN_POINT('Ctrl Pts',(99.4662876311982,2.14473699205026,0.507660550891255));
#11719=CARTESIAN_POINT('Ctrl Pts',(99.4703462379696,2.127422426552,0.580810195984218));
#11720=CARTESIAN_POINT('Ctrl Pts',(99.4744048447411,2.10636213167654,0.653069570337208));
#11721=CARTESIAN_POINT('Ctrl Pts',(99.4784634515125,2.081679520328,0.724034788285061));
#11722=CARTESIAN_POINT('Ctrl Pts',(99.482526206663,2.05697168041345,0.795072541130457));
#11723=CARTESIAN_POINT('Ctrl Pts',(99.4865889618135,2.0286342876539,0.864813044104926));
#11724=CARTESIAN_POINT('Ctrl Pts',(99.4906517169641,1.9968397770103,0.93287025086528));
#11725=CARTESIAN_POINT('Ctrl Pts',(99.4947165931353,1.96502866757765,1.00096298788527));
#11726=CARTESIAN_POINT('Ctrl Pts',(99.4987814693065,1.92975707025435,1.06737025661494));
#11727=CARTESIAN_POINT('Ctrl Pts',(99.5028463454778,1.89124324927213,1.1317309627657));
#11728=CARTESIAN_POINT('Ctrl Pts',(99.5069184804549,1.85266065267633,1.19620660030846));
#11729=CARTESIAN_POINT('Ctrl Pts',(99.5109906154321,1.81082453401622,1.2586279782448));
#11730=CARTESIAN_POINT('Ctrl Pts',(99.5150627504093,1.76599605057846,1.31866369834817));
#11731=CARTESIAN_POINT('Ctrl Pts',(99.5182001776582,1.73145738566371,1.36491896867078));
#11732=CARTESIAN_POINT('Ctrl Pts',(99.5213376049071,1.69514330785048,1.40975868348756));
#11733=CARTESIAN_POINT('Ctrl Pts',(99.524475032156,1.65718831331425,1.45304607436057));
#11734=CARTESIAN_POINT('Ctrl Pts',(99.5284883777273,1.60863690569746,1.50841859607012));
#11735=CARTESIAN_POINT('Ctrl Pts',(99.5325017232986,1.55720003307881,1.56147683584796));
#11736=CARTESIAN_POINT('Ctrl Pts',(99.5365150688698,1.50313021226308,1.61189812487699));
#11737=CARTESIAN_POINT('Ctrl Pts',(99.5405215924509,1.44915230074844,1.66223370647506));
#11738=CARTESIAN_POINT('Ctrl Pts',(99.544528116032,1.39255068593022,1.70994090581197));
#11739=CARTESIAN_POINT('Ctrl Pts',(99.5485346396131,1.33361720663063,1.75473107517326));
#11740=CARTESIAN_POINT('Ctrl Pts',(99.5525373552304,1.2747397401197,1.79947867412602));
#11741=CARTESIAN_POINT('Ctrl Pts',(99.5565400708476,1.21353519271828,1.84131444273081));
#11742=CARTESIAN_POINT('Ctrl Pts',(99.5605427864649,1.15033023490278,1.8799883910994));
#11743=CARTESIAN_POINT('Ctrl Pts',(99.5645430802893,1.08716351845349,1.91863894028107));
#11744=CARTESIAN_POINT('Ctrl Pts',(99.5685433741137,1.02199921149075,1.95413120698742));
#11745=CARTESIAN_POINT('Ctrl Pts',(99.5725436679381,0.955193379403557,1.98625819266872));
#11746=CARTESIAN_POINT('Ctrl Pts',(99.5765429227281,0.888404899432113,2.01837683370171));
#11747=CARTESIAN_POINT('Ctrl Pts',(99.580542177518,0.819976185039759,2.0471317165054));
#11748=CARTESIAN_POINT('Ctrl Pts',(99.584541432308,0.750286714981923,2.0723623827221));
#11749=CARTESIAN_POINT('Ctrl Pts',(99.5885430400031,0.680556244106896,2.09760789304557));
#11750=CARTESIAN_POINT('Ctrl Pts',(99.5925446476982,0.609563999543172,2.11932487609767));
#11751=CARTESIAN_POINT('Ctrl Pts',(99.5965462553934,0.53770706366451,2.13740195416896));
#11752=CARTESIAN_POINT('Ctrl Pts',(99.6005491822716,0.465826439193568,2.15548499158888));
#11753=CARTESIAN_POINT('Ctrl Pts',(99.6045521091498,0.393081039035946,2.16992563667628));
#11754=CARTESIAN_POINT('Ctrl Pts',(99.608555036028,0.319878123329642,2.18066365728764));
#11755=CARTESIAN_POINT('Ctrl Pts',(99.6125632404791,0.246578694811779,2.19141583521158));
#11756=CARTESIAN_POINT('Ctrl Pts',(99.6165714449303,0.172821037268198,2.19845559879149));
#11757=CARTESIAN_POINT('Ctrl Pts',(99.6205796493814,0.0990164677374564,
2.20177467946127));
#11758=CARTESIAN_POINT('Ctrl Pts',(99.6224025685218,0.0654503749680512,
2.20328418721099));
#11759=CARTESIAN_POINT('Ctrl Pts',(99.6242254876622,0.0318745667734997,
2.20402482283944));
#11760=CARTESIAN_POINT('Ctrl Pts',(99.6260484068026,-0.00167252030352725,
2.20399936539824));
#11761=CARTESIAN_POINT('',(100.349820515151,0.480300475185355,2.15472339387338));
#11762=CARTESIAN_POINT('Ctrl Pts',(99.6260484068026,-0.00167396307086296,
2.20590060288082));
#11763=CARTESIAN_POINT('Ctrl Pts',(99.6319075205934,-0.109592698905016,
2.20681139051173));
#11764=CARTESIAN_POINT('Ctrl Pts',(99.6774835397241,-0.948102371469299,
2.15053535437817));
#11765=CARTESIAN_POINT('Ctrl Pts',(99.7627764641942,-2.37345450507347,1.07511981627215));
#11766=CARTESIAN_POINT('Ctrl Pts',(99.8819271802135,-2.18961305998529,-1.41221794055659));
#11767=CARTESIAN_POINT('Ctrl Pts',(100.001077896233,0.000573147000856311,
-2.6057943353733));
#11768=CARTESIAN_POINT('Ctrl Pts',(100.120228612252,2.19048665599282,-1.41085615541611));
#11769=CARTESIAN_POINT('Ctrl Pts',(100.236476151891,2.36818650235432,1.01501035828337));
#11770=CARTESIAN_POINT('Ctrl Pts',(100.313006786191,1.14036460413367,2.00378250651846));
#11771=CARTESIAN_POINT('Ctrl Pts',(100.349820515151,0.480300475185355,2.15472339387338));
#11772=CARTESIAN_POINT('',(100.349869898682,1.9893770426062,0.948680653513814));
#11773=CARTESIAN_POINT('Origin',(100.349869898682,0.,0.));
#11774=CARTESIAN_POINT('',(99.7342548474101,-0.00178926204916046,2.20399927371615));
#11775=CARTESIAN_POINT('Ctrl Pts',(100.349869898682,1.9893770426062,0.948680653513813));
#11776=CARTESIAN_POINT('Ctrl Pts',(100.310152993343,2.30503304407864,0.286752110579726));
#11777=CARTESIAN_POINT('Ctrl Pts',(100.230719182663,2.21766422752178,-1.36580521532166));
#11778=CARTESIAN_POINT('Ctrl Pts',(100.111568466644,0.0501856098512207,
-2.6066853763117));
#11779=CARTESIAN_POINT('Ctrl Pts',(99.9924177506253,-2.1620698968013,-1.45316896147941));
#11780=CARTESIAN_POINT('Ctrl Pts',(99.8732670346058,-2.39365166732773,1.02916391750694));
#11781=CARTESIAN_POINT('Ctrl Pts',(99.7872127335343,-0.976535127098266,
2.14187097997843));
#11782=CARTESIAN_POINT('Ctrl Pts',(99.7408753378023,-0.12379021475703,2.20663616064201));
#11783=CARTESIAN_POINT('Ctrl Pts',(99.7342548474101,-0.00179052749946479,
2.20555804569826));
#11784=CARTESIAN_POINT('',(98.9842548474577,-0.000466138566021928,2.20399995070663));
#11785=CARTESIAN_POINT('Ctrl Pts',(99.7342548474101,-0.00178926204916046,
2.20399927371615));
#11786=CARTESIAN_POINT('Ctrl Pts',(99.7301177955417,0.0743921602789955,
2.20406111971104));
#11787=CARTESIAN_POINT('Ctrl Pts',(99.7259807436732,0.150715896488296,2.20016833951562));
#11788=CARTESIAN_POINT('Ctrl Pts',(99.7218436918048,0.226730373341687,2.19230685302134));
#11789=CARTESIAN_POINT('Ctrl Pts',(99.7178416649022,0.300263892144504,2.1847019494704));
#11790=CARTESIAN_POINT('Ctrl Pts',(99.7138396379996,0.373507490498452,2.17338344944699));
#11791=CARTESIAN_POINT('Ctrl Pts',(99.7098376110969,0.446051984251043,2.15839144442006));
#11792=CARTESIAN_POINT('Ctrl Pts',(99.7058380234803,0.51855226121741,2.14340857720976));
#11793=CARTESIAN_POINT('Ctrl Pts',(99.7018384358637,0.590353796805677,2.1247567438145));
#11794=CARTESIAN_POINT('Ctrl Pts',(99.6978388482471,0.661055196870396,2.10252753292095));
#11795=CARTESIAN_POINT('Ctrl Pts',(99.6938403161961,0.731737937518075,2.08030418873041));
#11796=CARTESIAN_POINT('Ctrl Pts',(99.6898417841452,0.801320648756876,2.05450548855933));
#11797=CARTESIAN_POINT('Ctrl Pts',(99.6858432520943,0.869416528199261,2.02527304344228));
#11798=CARTESIAN_POINT('Ctrl Pts',(99.6818443935192,0.937517968420832,1.99603821117385));
#11799=CARTESIAN_POINT('Ctrl Pts',(99.6778455349441,1.0041318842539,1.96336927512572));
#11800=CARTESIAN_POINT('Ctrl Pts',(99.6738466763689,1.06889260099549,1.92745547485204));
#11801=CARTESIAN_POINT('Ctrl Pts',(99.6698436806361,1.13372031817998,1.89150451871219));
#11802=CARTESIAN_POINT('Ctrl Pts',(99.6658406849033,1.1966905809756,1.85230224284687));
#11803=CARTESIAN_POINT('Ctrl Pts',(99.6618376891705,1.25746437939013,1.81008268721763));
#11804=CARTESIAN_POINT('Ctrl Pts',(99.6578321875143,1.31827622293191,1.76783670163982));
#11805=CARTESIAN_POINT('Ctrl Pts',(99.6538266858582,1.37688847994479,1.72256998339863));
#11806=CARTESIAN_POINT('Ctrl Pts',(99.649821184202,1.4329952624189,1.67455683029421));
#11807=CARTESIAN_POINT('Ctrl Pts',(99.6458092838468,1.48919167421968,1.62646697725452));
#11808=CARTESIAN_POINT('Ctrl Pts',(99.6417973834915,1.54287427675369,1.5756222814579));
#11809=CARTESIAN_POINT('Ctrl Pts',(99.6377854831363,1.59377480585921,1.52233303459146));
#11810=CARTESIAN_POINT('Ctrl Pts',(99.6368455229467,1.6057004437741,1.50984773681451));
#11811=CARTESIAN_POINT('Ctrl Pts',(99.6359055627572,1.61747354506083,1.49722838528258));
#11812=CARTESIAN_POINT('Ctrl Pts',(99.6349656025676,1.6290909969087,1.48447920961899));
#11813=CARTESIAN_POINT('Ctrl Pts',(99.630891816437,1.67944101676689,1.429224300346));
#11814=CARTESIAN_POINT('Ctrl Pts',(99.6268180303064,1.72707337135986,1.37129874505747));
#11815=CARTESIAN_POINT('Ctrl Pts',(99.6227442441758,1.77169212129934,1.31100077319804));
#11816=CARTESIAN_POINT('Ctrl Pts',(99.6186764265708,1.81624550007225,1.25079114421615));
#11817=CARTESIAN_POINT('Ctrl Pts',(99.6146086089659,1.85779375883192,1.18821638020305));
#11818=CARTESIAN_POINT('Ctrl Pts',(99.6105407913609,1.89607943995466,1.12360969975398));
#11819=CARTESIAN_POINT('Ctrl Pts',(99.6064777123138,1.93432052249017,1.0590782789474));
#11820=CARTESIAN_POINT('Ctrl Pts',(99.6024146332668,1.96930633614992,0.9925200528759));
#11821=CARTESIAN_POINT('Ctrl Pts',(99.5983515542198,2.00082215241775,0.924297957584244));
#11822=CARTESIAN_POINT('Ctrl Pts',(99.5942910415887,2.0323180619365,0.856118954310918));
#11823=CARTESIAN_POINT('Ctrl Pts',(99.5902305289577,2.06034812386471,0.786278599563272));
#11824=CARTESIAN_POINT('Ctrl Pts',(99.5861700163267,2.08474372803297,0.715164029036125));
#11825=CARTESIAN_POINT('Ctrl Pts',(99.5821107576639,2.10913179834626,0.64407142012377));
#11826=CARTESIAN_POINT('Ctrl Pts',(99.5780514990011,2.12988748463402,0.571705827876288));
#11827=CARTESIAN_POINT('Ctrl Pts',(99.5739922403383,2.14689106090511,0.498472439163638));
#11828=CARTESIAN_POINT('Ctrl Pts',(99.5699329248685,2.16389487513162,0.425238025591169));
#11829=CARTESIAN_POINT('Ctrl Pts',(99.5658736093987,2.17714636888608,0.351136256741012));
#11830=CARTESIAN_POINT('Ctrl Pts',(99.5618142939289,2.18657662602126,0.276583908674142));
#11831=CARTESIAN_POINT('Ctrl Pts',(99.5577508185871,2.19601654701804,0.201955161463279));
#11832=CARTESIAN_POINT('Ctrl Pts',(99.5536873432452,2.20162735158575,0.12687538750957));
#11833=CARTESIAN_POINT('Ctrl Pts',(99.5496238679034,2.20339196712703,0.0517671633382531));
#11834=CARTESIAN_POINT('Ctrl Pts',(99.5455582640324,2.205157507009,-0.0233804040138641));
#11835=CARTESIAN_POINT('Ctrl Pts',(99.5414926601615,2.20307285899171,-0.0985559737415544));
#11836=CARTESIAN_POINT('Ctrl Pts',(99.5374270562905,2.19717309413235,-0.173338958174133));
#11837=CARTESIAN_POINT('Ctrl Pts',(99.5333541895044,2.19126278975843,-0.248255537143437));
#11838=CARTESIAN_POINT('Ctrl Pts',(99.5292813227183,2.18152381717142,-0.322777656036424));
#11839=CARTESIAN_POINT('Ctrl Pts',(99.5252084559323,2.16804286873909,-0.396492268915249));
#11840=CARTESIAN_POINT('Ctrl Pts',(99.5220772661377,2.15767881551315,-0.45316351687983));
#11841=CARTESIAN_POINT('Ctrl Pts',(99.518946076343,2.14510416478066,-0.509357638457879));
#11842=CARTESIAN_POINT('Ctrl Pts',(99.5158148865484,2.1303782225379,-0.564893466891131));
#11843=CARTESIAN_POINT('Ctrl Pts',(99.5117423865472,2.11122531142885,-0.637124687672423));
#11844=CARTESIAN_POINT('Ctrl Pts',(99.507669886546,2.08835766175706,-0.708520398955298));
#11845=CARTESIAN_POINT('Ctrl Pts',(99.5035973865447,2.06186525068677,-0.778670461755417));
#11846=CARTESIAN_POINT('Ctrl Pts',(99.4995308792193,2.03541182314764,-0.848717298875088));
#11847=CARTESIAN_POINT('Ctrl Pts',(99.4954643718939,2.00534439126511,-0.917521683578741));
#11848=CARTESIAN_POINT('Ctrl Pts',(99.4913978645685,1.97180320036611,-0.984686822815248));
#11849=CARTESIAN_POINT('Ctrl Pts',(99.4873361257298,1.93830134069428,-1.05177320255399));
#11850=CARTESIAN_POINT('Ctrl Pts',(99.483274386891,1.90133402720749,-1.11722373067191));
#11851=CARTESIAN_POINT('Ctrl Pts',(99.4792126480523,1.86108964626999,-1.18066139453556));
#11852=CARTESIAN_POINT('Ctrl Pts',(99.4751534933172,1.82087086905829,-1.24405869896235));
#11853=CARTESIAN_POINT('Ctrl Pts',(99.471094338582,1.77737941679389,-1.30544527803626));
#11854=CARTESIAN_POINT('Ctrl Pts',(99.4670351838469,1.73084901870324,-1.36446974112804));
#11855=CARTESIAN_POINT('Ctrl Pts',(99.4629772988251,1.68433317543317,-1.42347574122564));
#11856=CARTESIAN_POINT('Ctrl Pts',(99.4589194138033,1.63478056916153,-1.48012071749539));
#11857=CARTESIAN_POINT('Ctrl Pts',(99.4548615287815,1.58246660369059,-1.53408456357659));
#11858=CARTESIAN_POINT('Ctrl Pts',(99.4508036007722,1.53015208402688,-1.58804898132871));
#11859=CARTESIAN_POINT('Ctrl Pts',(99.4467456727628,1.47507648081182,-1.63933187082003));
#11860=CARTESIAN_POINT('Ctrl Pts',(99.4426877447535,1.41755248405717,-1.68764953557999));
#11861=CARTESIAN_POINT('Ctrl Pts',(99.4386256687448,1.3599696864823,-1.73601659048109));
#11862=CARTESIAN_POINT('Ctrl Pts',(99.4345635927362,1.29993386406711,-1.78141205995232));
#11863=CARTESIAN_POINT('Ctrl Pts',(99.4305015167276,1.23779068576521,-1.82359266784907));
#11864=CARTESIAN_POINT('Ctrl Pts',(99.4264373209815,1.17561507891557,-1.86579528710563));
#11865=CARTESIAN_POINT('Ctrl Pts',(99.4223731252354,1.11133033503176,-1.90477945608713));
#11866=CARTESIAN_POINT('Ctrl Pts',(99.4183089294893,1.04530871568077,-1.94034679604493));
#11867=CARTESIAN_POINT('Ctrl Pts',(99.4142374693345,0.979169088228575,-1.97597770963655));
#11868=CARTESIAN_POINT('Ctrl Pts',(99.4101660091798,0.911286816445657,-2.00817939036449));
#11869=CARTESIAN_POINT('Ctrl Pts',(99.406094549025,0.842055802925244,-2.03680092909443));
#11870=CARTESIAN_POINT('Ctrl Pts',(99.4029510895265,0.788604490921365,-2.05889881151578));
#11871=CARTESIAN_POINT('Ctrl Pts',(99.3998076300279,0.734349660433825,-2.07886356027579));
#11872=CARTESIAN_POINT('Ctrl Pts',(99.3966641705294,0.679477986987283,-2.09664628995921));
#11873=CARTESIAN_POINT('Ctrl Pts',(99.3925909798832,0.608377090942739,-2.11968856177621));
#11874=CARTESIAN_POINT('Ctrl Pts',(99.3885177892369,0.535965708987452,-2.1391544187786));
#11875=CARTESIAN_POINT('Ctrl Pts',(99.3844445985907,0.462637481712026,-2.15489734338208));
#11876=CARTESIAN_POINT('Ctrl Pts',(99.3803773913427,0.389416971464416,-2.17061714208834));
#11877=CARTESIAN_POINT('Ctrl Pts',(99.3763101840948,0.315282752805154,-2.18262476699012));
#11878=CARTESIAN_POINT('Ctrl Pts',(99.3722429768469,0.240644467779498,-2.19082318778288));
#11879=CARTESIAN_POINT('Ctrl Pts',(99.3681805275575,0.166093497179889,-2.19901201778177));
#11880=CARTESIAN_POINT('Ctrl Pts',(99.3641180782681,0.0910401039530714,
-2.20340044515141));
#11881=CARTESIAN_POINT('Ctrl Pts',(99.3600556289787,0.0159033734873056,
-2.20394262237285));
#11882=CARTESIAN_POINT('Ctrl Pts',(99.3559957576903,-0.0591856757522623,
-2.20448445553255));
#11883=CARTESIAN_POINT('Ctrl Pts',(99.3519358864019,-0.134357481080633,
-2.20118487862807));
#11884=CARTESIAN_POINT('Ctrl Pts',(99.3478760151135,-0.209189938435319,
-2.19405003809335));
#11885=CARTESIAN_POINT('Ctrl Pts',(99.343817408466,-0.28399908564479,-2.1869174200457));
#11886=CARTESIAN_POINT('Ctrl Pts',(99.3397588018185,-0.358468619794764,
-2.17595195563659));
#11887=CARTESIAN_POINT('Ctrl Pts',(99.335700195171,-0.432180162262118,-2.16121176827887));
#11888=CARTESIAN_POINT('Ctrl Pts',(99.331641541488,-0.505892558978118,-2.14647141009601));
#11889=CARTESIAN_POINT('Ctrl Pts',(99.3275828878051,-0.57884647876335,-2.12795633748231));
#11890=CARTESIAN_POINT('Ctrl Pts',(99.3235242341221,-0.650633951486543,
-2.10577573857546));
#11891=CARTESIAN_POINT('Ctrl Pts',(99.3194614312018,-0.722494813881127,
-2.08357246402892));
#11892=CARTESIAN_POINT('Ctrl Pts',(99.3153986282815,-0.793186390734587,
-2.0576963212229));
#11893=CARTESIAN_POINT('Ctrl Pts',(99.3113358253612,-0.862316822649757,
-2.02830611530292));
#11894=CARTESIAN_POINT('Ctrl Pts',(99.3072709008695,-0.931483354063812,
-1.99890056199286));
#11895=CARTESIAN_POINT('Ctrl Pts',(99.3032059763777,-0.999086687470405,
-1.96597750051935));
#11896=CARTESIAN_POINT('Ctrl Pts',(99.299141051886,-1.06475829435055,-1.92974241146629));
#11897=CARTESIAN_POINT('Ctrl Pts',(99.2950688682582,-1.13054717748865,-1.89344261384505));
#11898=CARTESIAN_POINT('Ctrl Pts',(99.2909966846303,-1.19439703737409,-1.85381922677039));
#11899=CARTESIAN_POINT('Ctrl Pts',(99.2869245010025,-1.25596752021542,-1.81112163814691));
#11900=CARTESIAN_POINT('Ctrl Pts',(99.2837874855051,-1.3033984753269,-1.77822945806464));
#11901=CARTESIAN_POINT('Ctrl Pts',(99.2806504700076,-1.34947732050749,-1.74351382884607));
#11902=CARTESIAN_POINT('Ctrl Pts',(99.2775134545102,-1.39406271455528,-1.70710431663878));
#11903=CARTESIAN_POINT('Ctrl Pts',(99.2734403154914,-1.45195293164663,-1.65982976381973));
#11904=CARTESIAN_POINT('Ctrl Pts',(99.2693671764726,-1.50754729424262,-1.60951604503001));
#11905=CARTESIAN_POINT('Ctrl Pts',(99.2652940374537,-1.56050937957516,-1.55641462221927));
#11906=CARTESIAN_POINT('Ctrl Pts',(99.2612268808056,-1.61339367752509,-1.50339119144127));
#11907=CARTESIAN_POINT('Ctrl Pts',(99.2571597241573,-1.66365303969438,-1.44758852095762));
#11908=CARTESIAN_POINT('Ctrl Pts',(99.2530925675092,-1.71098396732507,-1.38929833497221));
#11909=CARTESIAN_POINT('Ctrl Pts',(99.2490301670178,-1.75825954589085,-1.33107631387285));
#11910=CARTESIAN_POINT('Ctrl Pts',(99.2449677665265,-1.80261319423376,-1.27037292540568));
#11911=CARTESIAN_POINT('Ctrl Pts',(99.2409053660352,-1.84377931595503,-1.20751556265599));
#11912=CARTESIAN_POINT('Ctrl Pts',(99.2368455424143,-1.88491932509632,-1.14469807171942));
#11913=CARTESIAN_POINT('Ctrl Pts',(99.2327857187933,-1.92287555898522,-1.07972971620207));
#11914=CARTESIAN_POINT('Ctrl Pts',(99.2287258951723,-1.95742448661696,-1.01296859733771));
#11915=CARTESIAN_POINT('Ctrl Pts',(99.2246673349892,-1.99196266244554,-0.946228254875343));
#11916=CARTESIAN_POINT('Ctrl Pts',(99.2206087748061,-2.023095418051,-0.877696680538174));
#11917=CARTESIAN_POINT('Ctrl Pts',(99.2165502146231,-2.05064492767362,-0.807757005916043));
#11918=CARTESIAN_POINT('Ctrl Pts',(99.2124916061278,-2.07819476523911,-0.737816498748508));
#11919=CARTESIAN_POINT('Ctrl Pts',(99.2084329976326,-2.10216109881843,-0.666468302891899));
#11920=CARTESIAN_POINT('Ctrl Pts',(99.2043743891374,-2.12241466213535,-0.5941144687288));
#11921=CARTESIAN_POINT('Ctrl Pts',(99.2003116290888,-2.14268894283582,-0.521686623780005));
#11922=CARTESIAN_POINT('Ctrl Pts',(99.1962488690402,-2.1592427403123,-0.448251547122586));
#11923=CARTESIAN_POINT('Ctrl Pts',(99.1921861089916,-2.17199722044688,-0.374224630898386));
#11924=CARTESIAN_POINT('Ctrl Pts',(99.1881212261541,-2.18475836478738,-0.300159035668188));
#11925=CARTESIAN_POINT('Ctrl Pts',(99.1840563433165,-2.1937161816409,-0.225501459539191));
#11926=CARTESIAN_POINT('Ctrl Pts',(99.179991460479,-2.19884370864308,-0.150672973557745));
#11927=CARTESIAN_POINT('Ctrl Pts',(99.1759193160121,-2.20398039561424,-0.075710811710773));
#11928=CARTESIAN_POINT('Ctrl Pts',(99.1718471715452,-2.20527311705613,-0.000577608238949548));
#11929=CARTESIAN_POINT('Ctrl Pts',(99.1677750270782,-2.20274708011188,0.0743054577980183));
#11930=CARTESIAN_POINT('Ctrl Pts',(99.1646375975492,-2.20080086652228,0.131999958697744));
#11931=CARTESIAN_POINT('Ctrl Pts',(99.1615001680201,-2.19658887303926,0.189545959249616));
#11932=CARTESIAN_POINT('Ctrl Pts',(99.1583627384911,-2.19014343654103,0.24675438674162));
#11933=CARTESIAN_POINT('Ctrl Pts',(99.1542897455551,-2.18177600801924,0.321022037662551));
#11934=CARTESIAN_POINT('Ctrl Pts',(99.1502167526192,-2.1696105373008,0.395006868667691));
#11935=CARTESIAN_POINT('Ctrl Pts',(99.1461437596832,-2.15367606013578,0.468289897390542));
#11936=CARTESIAN_POINT('Ctrl Pts',(99.1420767520201,-2.13776499872324,0.541465236526569));
#11937=CARTESIAN_POINT('Ctrl Pts',(99.1380097443571,-2.11809602776835,0.613940358226609));
#11938=CARTESIAN_POINT('Ctrl Pts',(99.133942736694,-2.09474986256318,0.685302132852038));
#11939=CARTESIAN_POINT('Ctrl Pts',(99.1298804888272,-2.07143102039191,0.75658038968468));
#11940=CARTESIAN_POINT('Ctrl Pts',(99.1258182409603,-2.04444368191489,0.826747436671027));
#11941=CARTESIAN_POINT('Ctrl Pts',(99.1217559930934,-2.01391907905545,0.895402670878566));
#11942=CARTESIAN_POINT('Ctrl Pts',(99.117696324253,-1.98341385555471,0.964014317478532));
#11943=CARTESIAN_POINT('Ctrl Pts',(99.1136366554126,-1.94937601755784,1.03111562075139));
#11944=CARTESIAN_POINT('Ctrl Pts',(99.1095769865722,-1.91198540020253,1.09632469160025));
#11945=CARTESIAN_POINT('Ctrl Pts',(99.105518583105,-1.87460643726626,1.16151343719398));
#11946=CARTESIAN_POINT('Ctrl Pts',(99.1014601796377,-1.83387700720655,1.22481070743143));
#11947=CARTESIAN_POINT('Ctrl Pts',(99.0974017761704,-1.79002274859216,1.28585946336392));
#11948=CARTESIAN_POINT('Ctrl Pts',(99.0933433261073,-1.74616798647374,1.34690892021569));
#11949=CARTESIAN_POINT('Ctrl Pts',(99.0892848760443,-1.69918860459373,1.40570942475502));
#11950=CARTESIAN_POINT('Ctrl Pts',(99.0852264259812,-1.64935245476583,1.46193449920232));
#11951=CARTESIAN_POINT('Ctrl Pts',(99.0811638259375,-1.59946534482858,1.51821706677362));
#11952=CARTESIAN_POINT('Ctrl Pts',(99.0771012258938,-1.54671595089979,1.57191858716061));
#11953=CARTESIAN_POINT('Ctrl Pts',(99.07303862585,-1.49141066508986,1.62274774011743));
#11954=CARTESIAN_POINT('Ctrl Pts',(99.0689739041421,-1.43607649648385,1.67360343824147));
#11955=CARTESIAN_POINT('Ctrl Pts',(99.064909182434,-1.37818414585655,1.72158347671752));
#11956=CARTESIAN_POINT('Ctrl Pts',(99.060844460726,-1.31807288491114,1.76643705522219));
#11957=CARTESIAN_POINT('Ctrl Pts',(99.0567724774148,-1.25785423552448,1.81137076440128));
#11958=CARTESIAN_POINT('Ctrl Pts',(99.0527004941035,-1.19540915528624,1.8531665912189));
#11959=CARTESIAN_POINT('Ctrl Pts',(99.0486285107923,-1.13110527439736,1.89161752429778));
#11960=CARTESIAN_POINT('Ctrl Pts',(99.0454896813522,-1.08153755787727,1.92125686992423));
#11961=CARTESIAN_POINT('Ctrl Pts',(99.0423508519121,-1.03086596171574,1.94890961628639));
#11962=CARTESIAN_POINT('Ctrl Pts',(99.039212022472,-0.97926716831074,1.97450039581375));
#11963=CARTESIAN_POINT('Ctrl Pts',(99.0346322578875,-0.90398103660152,2.01183907509093));
#11964=CARTESIAN_POINT('Ctrl Pts',(99.0300524933029,-0.826449303819452,
2.04492059732323));
#11965=CARTESIAN_POINT('Ctrl Pts',(99.0254727287184,-0.74716224320077,2.07349091686826));
#11966=CARTESIAN_POINT('Ctrl Pts',(99.0211239147306,-0.671873509051896,
2.10062047843846));
#11967=CARTESIAN_POINT('Ctrl Pts',(99.0167751007428,-0.595002578912433,
2.12368253475061));
#11968=CARTESIAN_POINT('Ctrl Pts',(99.012426286755,-0.516994574433637,2.14250615168456));
#11969=CARTESIAN_POINT('Ctrl Pts',(99.0080869948121,-0.439157374160702,
2.16128855293861));
#11970=CARTESIAN_POINT('Ctrl Pts',(99.0037477028693,-0.360188413294784,
2.17585089502794));
#11971=CARTESIAN_POINT('Ctrl Pts',(98.9994084109264,-0.28054952401915,2.18607135395271));
#11972=CARTESIAN_POINT('Ctrl Pts',(98.99508172104,-0.201141919892249,2.19626213089191));
#11973=CARTESIAN_POINT('Ctrl Pts',(98.9907550311536,-0.121068629902613,
2.20213609041139));
#11974=CARTESIAN_POINT('Ctrl Pts',(98.9864283412672,-0.0408017934233111,
2.20362229378209));
#11975=CARTESIAN_POINT('Ctrl Pts',(98.9857038433307,-0.0273612282512411,
2.20387115637764));
#11976=CARTESIAN_POINT('Ctrl Pts',(98.9849793453942,-0.0139152616418334,
2.2039971062624));
#11977=CARTESIAN_POINT('Ctrl Pts',(98.9842548474577,-0.000466138566033943,
2.20399995070663));
#11978=CARTESIAN_POINT('',(98.2342548473827,0.00202208611722839,2.20399907240628));
#11979=CARTESIAN_POINT('Ctrl Pts',(98.9842548474101,-0.000466137681637975,
2.20399995070682));
#11980=CARTESIAN_POINT('Ctrl Pts',(98.9800659211421,0.0772944494749427,
2.20401639677789));
#11981=CARTESIAN_POINT('Ctrl Pts',(98.975876994874,0.155004589942922,2.1999132369169));
#11982=CARTESIAN_POINT('Ctrl Pts',(98.971688068606,0.232216947609706,2.19173248578444));
#11983=CARTESIAN_POINT('Ctrl Pts',(98.9673858384265,0.311517778926223,2.18333045811424));
#11984=CARTESIAN_POINT('Ctrl Pts',(98.9630836082471,0.390293025390627,2.17062713283996));
#11985=CARTESIAN_POINT('Ctrl Pts',(98.9587813780677,0.468068877566995,2.15372410625251));
#11986=CARTESIAN_POINT('Ctrl Pts',(98.9545794155905,0.544032087074628,2.13721502131104));
#11987=CARTESIAN_POINT('Ctrl Pts',(98.9503774531134,0.619041586376206,2.11670007151106));
#11988=CARTESIAN_POINT('Ctrl Pts',(98.9461754906363,0.692672418946442,2.0923242865366));
#11989=CARTESIAN_POINT('Ctrl Pts',(98.9418231266057,0.768938732357677,2.06707601496865));
#11990=CARTESIAN_POINT('Ctrl Pts',(98.9374707625751,0.843725343475413,2.03768550765046));
#11991=CARTESIAN_POINT('Ctrl Pts',(98.9331183985445,0.916585256674168,2.00436709892364));
#11992=CARTESIAN_POINT('Ctrl Pts',(98.9287660345139,0.989445169872913,1.97104869019682));
#11993=CARTESIAN_POINT('Ctrl Pts',(98.9244136704833,1.06037797311012,1.93380268451775));
#11994=CARTESIAN_POINT('Ctrl Pts',(98.9200613064528,1.12896878897367,1.89289341314384));
#11995=CARTESIAN_POINT('Ctrl Pts',(98.9159882345174,1.19315811807277,1.85460929812984));
#11996=CARTESIAN_POINT('Ctrl Pts',(98.911915162582,1.2555216575691,1.81298260017475));
#11997=CARTESIAN_POINT('Ctrl Pts',(98.9078420906466,1.31568978311253,1.76821276847932));
#11998=CARTESIAN_POINT('Ctrl Pts',(98.9037750026509,1.37576951286062,1.72350871022863));
#11999=CARTESIAN_POINT('Ctrl Pts',(98.8997079146552,1.43365985248843,1.6756709689612));
#12000=CARTESIAN_POINT('Ctrl Pts',(98.8956408266595,1.4890178468179,1.62494364574831));
#12001=CARTESIAN_POINT('Ctrl Pts',(98.8915784968471,1.5443110765083,1.57427566964179));
#12002=CARTESIAN_POINT('Ctrl Pts',(98.8875161670347,1.59707749676501,1.52072514900194));
#12003=CARTESIAN_POINT('Ctrl Pts',(98.8834538372224,1.64700641957879,1.46457702216929));
#12004=CARTESIAN_POINT('Ctrl Pts',(98.8793940854881,1.69690365597848,1.40846452864689));
#12005=CARTESIAN_POINT('Ctrl Pts',(98.8753343337539,1.74396665188229,1.34975805613334));
#12006=CARTESIAN_POINT('Ctrl Pts',(98.8712745820197,1.78792183141841,1.28877908298413));
#12007=CARTESIAN_POINT('Ctrl Pts',(98.867216094829,1.83186331966421,1.22781910374723));
#12008=CARTESIAN_POINT('Ctrl Pts',(98.8631576076384,1.87269863451879,1.16458841634131));
#12009=CARTESIAN_POINT('Ctrl Pts',(98.8590991204477,1.91019574487544,1.09943995573191));
#12010=CARTESIAN_POINT('Ctrl Pts',(98.8550405859496,1.94769329231425,1.03429073572453));
#12011=CARTESIAN_POINT('Ctrl Pts',(98.8509820514515,1.98185232137401,0.967224112833762));
#12012=CARTESIAN_POINT('Ctrl Pts',(98.8469235169534,2.01248606470643,0.898618850994355));
#12013=CARTESIAN_POINT('Ctrl Pts',(98.8428608319543,2.04315113594403,0.829943429295143));
#12014=CARTESIAN_POINT('Ctrl Pts',(98.8387981469551,2.07028352703557,0.75972666338779));
#12015=CARTESIAN_POINT('Ctrl Pts',(98.8347354619559,2.09374440406664,0.688367903406034));
#12016=CARTESIAN_POINT('Ctrl Pts',(98.8306706548699,2.11721753555982,0.616971870170623));
#12017=CARTESIAN_POINT('Ctrl Pts',(98.8266058477839,2.13701520812239,0.544433116020145));
#12018=CARTESIAN_POINT('Ctrl Pts',(98.8225410406978,2.15304906800389,0.471164207859177));
#12019=CARTESIAN_POINT('Ctrl Pts',(98.818468972282,2.16911157060874,0.397764412869827));
#12020=CARTESIAN_POINT('Ctrl Pts',(98.8143969038661,2.18139675241525,0.323632330286333));
#12021=CARTESIAN_POINT('Ctrl Pts',(98.8103248354503,2.18986785055103,0.249188276455825));
#12022=CARTESIAN_POINT('Ctrl Pts',(98.8071867537781,2.19639598197921,0.19181902400911));
#12023=CARTESIAN_POINT('Ctrl Pts',(98.8040486721059,2.20066006838065,0.134264671864022));
#12024=CARTESIAN_POINT('Ctrl Pts',(98.8009105904337,2.20266440573115,0.0767171149422006));
#12025=CARTESIAN_POINT('Ctrl Pts',(98.796837534475,2.20526592444271,0.00202357789872107));
#12026=CARTESIAN_POINT('Ctrl Pts',(98.7927644785163,2.20406880647379,-0.0729464854661871));
#12027=CARTESIAN_POINT('Ctrl Pts',(98.7886914225577,2.19904041407215,-0.147774345802607));
#12028=CARTESIAN_POINT('Ctrl Pts',(98.7846243508788,2.19401940956488,-0.222492266364284));
#12029=CARTESIAN_POINT('Ctrl Pts',(98.7805572792,2.18517833832298,-0.297067926274521));
#12030=CARTESIAN_POINT('Ctrl Pts',(98.7764902075211,2.17253654210778,-0.371080817621158));
#12031=CARTESIAN_POINT('Ctrl Pts',(98.7724278944578,2.15990953723449,-0.445007111306859));
#12032=CARTESIAN_POINT('Ctrl Pts',(98.7683655813945,2.14349072250751,-0.5183714763544));
#12033=CARTESIAN_POINT('Ctrl Pts',(98.7643032683311,2.12335124622355,-0.5907583982991));
#12034=CARTESIAN_POINT('Ctrl Pts',(98.7602435336027,2.10322455238986,-0.663099376535162));
#12035=CARTESIAN_POINT('Ctrl Pts',(98.7561837988743,2.07938201077449,-0.734463683918276));
#12036=CARTESIAN_POINT('Ctrl Pts',(98.7521240641459,2.05194558955012,-0.804447199961441));
#12037=CARTESIAN_POINT('Ctrl Pts',(98.7480655941936,2.02451771591133,-0.874408913230569));
#12038=CARTESIAN_POINT('Ctrl Pts',(98.7440071242412,1.99349835982372,-0.942990245018632));
#12039=CARTESIAN_POINT('Ctrl Pts',(98.7399486542889,1.95905843849026,-1.00980494877977));
#12040=CARTESIAN_POINT('Ctrl Pts',(98.7358901372377,1.92461811747864,-1.07662042793112));
#12041=CARTESIAN_POINT('Ctrl Pts',(98.7318316201865,1.88675737275609,-1.14166881476953));
#12042=CARTESIAN_POINT('Ctrl Pts',(98.7277731031353,1.84569335560361,-1.20458791172778));
#12043=CARTESIAN_POINT('Ctrl Pts',(98.7237104357869,1.80458734580317,-1.26757135064941));
#12044=CARTESIAN_POINT('Ctrl Pts',(98.7196477684384,1.76027178369827,-1.32842075073339));
#12045=CARTESIAN_POINT('Ctrl Pts',(98.71558510109,1.71300709461038,-1.386803047954));
#12046=CARTESIAN_POINT('Ctrl Pts',(98.7115203117955,1.66571771900266,-1.4452158384618));
#12047=CARTESIAN_POINT('Ctrl Pts',(98.7074555225011,1.6154764683021,-1.50115860446677));
#12048=CARTESIAN_POINT('Ctrl Pts',(98.7033907332066,1.56258222777984,-1.55433354896129));
#12049=CARTESIAN_POINT('Ctrl Pts',(98.6993186826129,1.50959349751127,-1.60760348464892));
#12050=CARTESIAN_POINT('Ctrl Pts',(98.6952466320192,1.45394266522222,-1.65809540144811));
#12051=CARTESIAN_POINT('Ctrl Pts',(98.6911745814255,1.39596308267522,-1.70555066527146));
#12052=CARTESIAN_POINT('Ctrl Pts',(98.6880363457552,1.35127955286296,-1.74212334487086));
#12053=CARTESIAN_POINT('Ctrl Pts',(98.6848981100848,1.30521359901653,-1.7768932234169));
#12054=CARTESIAN_POINT('Ctrl Pts',(98.6817598744145,1.25792886057399,-1.8097599237841));
#12055=CARTESIAN_POINT('Ctrl Pts',(98.6776868063584,1.19655872208867,-1.85241711127264));
#12056=CARTESIAN_POINT('Ctrl Pts',(98.6736137383024,1.13289797794599,-1.89203136868507));
#12057=CARTESIAN_POINT('Ctrl Pts',(98.6695406702463,1.06728088726471,-1.92834838856454));
#12058=CARTESIAN_POINT('Ctrl Pts',(98.6654735862884,1.00176020035204,-1.96461205195495));
#12059=CARTESIAN_POINT('Ctrl Pts',(98.6614065023305,0.934289287714346,-1.99758786635259));
#12060=CARTESIAN_POINT('Ctrl Pts',(98.6573394183727,0.865232066629473,-2.02706424932119));
#12061=CARTESIAN_POINT('Ctrl Pts',(98.6532770928171,0.796255641035015,-2.05650614554416));
#12062=CARTESIAN_POINT('Ctrl Pts',(98.6492147672615,0.725697031260407,-2.0824565582041));
#12063=CARTESIAN_POINT('Ctrl Pts',(98.645152441706,0.653944027213801,-2.10475015364565));
#12064=CARTESIAN_POINT('Ctrl Pts',(98.6410926943609,0.582236562191627,-2.12702960015225));
#12065=CARTESIAN_POINT('Ctrl Pts',(98.6370329470157,0.509336661946798,-2.14565669360773));
#12066=CARTESIAN_POINT('Ctrl Pts',(98.6329731996706,0.435650074823647,-2.16051498775319));
#12067=CARTESIAN_POINT('Ctrl Pts',(98.6289147169952,0.361986442133028,-2.17536865332614));
#12068=CARTESIAN_POINT('Ctrl Pts',(98.6248562343198,0.287537076862959,-2.18645575627118));
#12069=CARTESIAN_POINT('Ctrl Pts',(98.6207977516444,0.212719225792712,-2.19371067622377));
#12070=CARTESIAN_POINT('Ctrl Pts',(98.6167392217818,0.13790050482908,-2.20096568052798));
#12071=CARTESIAN_POINT('Ctrl Pts',(98.6126806919192,0.062713764962516,-2.20438836907451));
#12072=CARTESIAN_POINT('Ctrl Pts',(98.6086221620565,-0.0124189096529951,
-2.20396501122024));
#12073=CARTESIAN_POINT('Ctrl Pts',(98.6045594818485,-0.0876284166600681,
-2.20354122043054));
#12074=CARTESIAN_POINT('Ctrl Pts',(98.6004968016404,-0.162783269495413,
-2.19926353185));
#12075=CARTESIAN_POINT('Ctrl Pts',(98.5964341214323,-0.237462423946303,
-2.19117037156255));
#12076=CARTESIAN_POINT('Ctrl Pts',(98.5923693192312,-0.312180584333164,
-2.18307298410763));
#12077=CARTESIAN_POINT('Ctrl Pts',(98.58830451703,-0.386422079680152,-2.17115623207429));
#12078=CARTESIAN_POINT('Ctrl Pts',(98.5842397148289,-0.459774669191026,
-2.15550997528898));
#12079=CARTESIAN_POINT('Ctrl Pts',(98.5801676513979,-0.533258293373165,
-2.13983576854133));
#12080=CARTESIAN_POINT('Ctrl Pts',(98.5760955879668,-0.605849378058541,
-2.1204188732418));
#12081=CARTESIAN_POINT('Ctrl Pts',(98.5720235245358,-0.677149924069375,
-2.09739933735396));
#12082=CARTESIAN_POINT('Ctrl Pts',(98.568885402489,-0.732097451084112,-2.07965940910893));
#12083=CARTESIAN_POINT('Ctrl Pts',(98.5657472804422,-0.786278811957624,
-2.05978092427929));
#12084=CARTESIAN_POINT('Ctrl Pts',(98.5626091583954,-0.839520996472622,
-2.03784702479887));
#12085=CARTESIAN_POINT('Ctrl Pts',(98.5585360928936,-0.908625671738396,
-2.00937833939999));
#12086=CARTESIAN_POINT('Ctrl Pts',(98.5544630273918,-0.976413882151996,
-1.97733569537347));
#12087=CARTESIAN_POINT('Ctrl Pts',(98.5503899618901,-1.04249077563177,-1.94186224607274));
#12088=CARTESIAN_POINT('Ctrl Pts',(98.5463228804995,-1.10847058953349,-1.90644091404492));
#12089=CARTESIAN_POINT('Ctrl Pts',(98.542255799109,-1.17274366113594,-1.86759900817242));
#12090=CARTESIAN_POINT('Ctrl Pts',(98.5381887177184,-1.23493497904427,-1.82552775863117));
#12091=CARTESIAN_POINT('Ctrl Pts',(98.5341263947373,-1.29705353427032,-1.78350573166738));
#12092=CARTESIAN_POINT('Ctrl Pts',(98.5300640717561,-1.35709478132595,-1.73826213378279));
#12093=CARTESIAN_POINT('Ctrl Pts',(98.5260017487749,-1.41470964593181,-1.69003331851993));
#12094=CARTESIAN_POINT('Ctrl Pts',(98.5219420040072,-1.47228794441086,-1.64183511238871));
#12095=CARTESIAN_POINT('Ctrl Pts',(98.5178822592395,-1.52744255109358,-1.59065575422982));
#12096=CARTESIAN_POINT('Ctrl Pts',(98.5138225144717,-1.57985575099939,-1.53677317976147));
#12097=CARTESIAN_POINT('Ctrl Pts',(98.509764034373,-1.63225262343827,-1.48290739049138));
#12098=CARTESIAN_POINT('Ctrl Pts',(98.5057055542742,-1.68190945195677,-1.42634039887376));
#12099=CARTESIAN_POINT('Ctrl Pts',(98.5016470741755,-1.72854501034008,-1.36738734352355));
#12100=CARTESIAN_POINT('Ctrl Pts',(98.497588546885,-1.77518111099854,-1.30843360267119));
#12101=CARTESIAN_POINT('Ctrl Pts',(98.4935300195945,-1.81879557695176,-1.24709411857095));
#12102=CARTESIAN_POINT('Ctrl Pts',(98.489471492304,-1.85914817399835,-1.1837162105499));
#12103=CARTESIAN_POINT('Ctrl Pts',(98.4854088146429,-1.89954203680996,-1.12027349039651));
#12104=CARTESIAN_POINT('Ctrl Pts',(98.4813461369818,-1.93666711254185,-1.05478858723801));
#12105=CARTESIAN_POINT('Ctrl Pts',(98.4772834593207,-1.97032756787706,-0.987636205929935));
#12106=CARTESIAN_POINT('Ctrl Pts',(98.4732186596566,-2.00400560461829,-0.920448749835463));
#12107=CARTESIAN_POINT('Ctrl Pts',(98.4691538599926,-2.03421522525858,-0.85159251881448));
#12108=CARTESIAN_POINT('Ctrl Pts',(98.4650890603285,-2.06080859611859,-0.781462686354086));
#12109=CARTESIAN_POINT('Ctrl Pts',(98.4610169993891,-2.08744947283495,-0.711207575388574));
#12110=CARTESIAN_POINT('Ctrl Pts',(98.4569449384496,-2.11046104999968,-0.639674773772419));
#12111=CARTESIAN_POINT('Ctrl Pts',(98.4528728775102,-2.12974539317599,-0.567274677952076));
#12112=CARTESIAN_POINT('Ctrl Pts',(98.4497347324655,-2.14460692567234,-0.511479343522763));
#12113=CARTESIAN_POINT('Ctrl Pts',(98.4465965874209,-2.15725585695442,-0.455169245346742));
#12114=CARTESIAN_POINT('Ctrl Pts',(98.4434584423762,-2.16766832644021,-0.398534849853682));
#12115=CARTESIAN_POINT('Ctrl Pts',(98.4393853785347,-2.18118288754535,-0.325027887880069));
#12116=CARTESIAN_POINT('Ctrl Pts',(98.4353123146932,-2.19098027329576,-0.25069096209894));
#12117=CARTESIAN_POINT('Ctrl Pts',(98.4312392508518,-2.19696686395659,-0.175933506407276));
#12118=CARTESIAN_POINT('Ctrl Pts',(98.4271721711602,-2.20294465911178,-0.101285884452472));
#12119=CARTESIAN_POINT('Ctrl Pts',(98.4231050914687,-2.2051227373313,-0.0262194312439857));
#12120=CARTESIAN_POINT('Ctrl Pts',(98.4190380117771,-2.20345863725056,0.0488470462354287));
#12121=CARTESIAN_POINT('Ctrl Pts',(98.4149756905449,-2.20179648415711,0.123825696377855));
#12122=CARTESIAN_POINT('Ctrl Pts',(98.4109133693126,-2.19630109447879,0.198803895789822));
#12123=CARTESIAN_POINT('Ctrl Pts',(98.4068510480804,-2.1869819860372,0.273360188668321));
#12124=CARTESIAN_POINT('Ctrl Pts',(98.4027913050913,-2.17766879217654,0.347869162725441));
#12125=CARTESIAN_POINT('Ctrl Pts',(98.3987315621023,-2.16453675436123,0.421956289040943));
#12126=CARTESIAN_POINT('Ctrl Pts',(98.3946718191132,-2.14764733110511,0.495203938995964));
#12127=CARTESIAN_POINT('Ctrl Pts',(98.3906133408203,-2.13076316926325,0.568428770751416));
#12128=CARTESIAN_POINT('Ctrl Pts',(98.3865548625275,-2.11012405317688,0.640814180423116));
#12129=CARTESIAN_POINT('Ctrl Pts',(98.3824963842346,-2.08584248054946,0.711953050653816));
#12130=CARTESIAN_POINT('Ctrl Pts',(98.3784378587748,-2.0615606257254,0.78309274764936));
#12131=CARTESIAN_POINT('Ctrl Pts',(98.3743793333149,-2.03363638623842,0.852985425154341));
#12132=CARTESIAN_POINT('Ctrl Pts',(98.370320807855,-2.00223151782014,0.921240983156772));
#12133=CARTESIAN_POINT('Ctrl Pts',(98.3662581320504,-1.97079453403554,0.98956634091825));
#12134=CARTESIAN_POINT('Ctrl Pts',(98.3621954562458,-1.93587001346819,1.05625080126569));
#12135=CARTESIAN_POINT('Ctrl Pts',(98.3581327804411,-1.89766678655087,1.12092674480614));
#12136=CARTESIAN_POINT('Ctrl Pts',(98.3540679826508,-1.85944360561686,1.18563646938975));
#12137=CARTESIAN_POINT('Ctrl Pts',(98.3500031848605,-1.8179385718371,1.24833518953764));
#12138=CARTESIAN_POINT('Ctrl Pts',(98.3459383870701,-1.77340372661367,1.30868453892936));
#12139=CARTESIAN_POINT('Ctrl Pts',(98.3418663280117,-1.728789325292,1.36914169511248));
#12140=CARTESIAN_POINT('Ctrl Pts',(98.3377942689532,-1.68113460494581,1.42724072791491));
#12141=CARTESIAN_POINT('Ctrl Pts',(98.3337222098947,-1.63073143823414,1.48267696291364));
#12142=CARTESIAN_POINT('Ctrl Pts',(98.3305840487155,-1.59188788051238,1.52539929038897));
#12143=CARTESIAN_POINT('Ctrl Pts',(98.3274458875363,-1.55141281655021,1.56654083295959));
#12144=CARTESIAN_POINT('Ctrl Pts',(98.3243077263571,-1.50945340650252,1.60597833534514));
#12145=CARTESIAN_POINT('Ctrl Pts',(98.3202847758764,-1.45566374460082,1.65653504996899));
#12146=CARTESIAN_POINT('Ctrl Pts',(98.3162618253957,-1.39921494262276,1.70449547284695));
#12147=CARTESIAN_POINT('Ctrl Pts',(98.3122388749149,-1.34039097563458,1.74956224022965));
#12148=CARTESIAN_POINT('Ctrl Pts',(98.3082213064714,-1.28164570530911,1.79456871578958));
#12149=CARTESIAN_POINT('Ctrl Pts',(98.3042037380278,-1.22053195433016,1.83668891555991));
#12150=CARTESIAN_POINT('Ctrl Pts',(98.3001861695843,-1.15736980930053,1.87566284937343));
#12151=CARTESIAN_POINT('Ctrl Pts',(98.2961726017163,-1.09427055926356,1.91459797409837));
#12152=CARTESIAN_POINT('Ctrl Pts',(98.2921590338484,-1.02912737514308,1.95039279055704));
#12153=CARTESIAN_POINT('Ctrl Pts',(98.2881454659804,-0.96229122060861,1.98282919252758));
#12154=CARTESIAN_POINT('Ctrl Pts',(98.2841345225613,-0.895498769848787,
2.0152443845226));
#12155=CARTESIAN_POINT('Ctrl Pts',(98.2801235791422,-0.827015985307934,
2.04430530678105));
#12156=CARTESIAN_POINT('Ctrl Pts',(98.276112635723,-0.757218903963501,2.06983949413483));
#12157=CARTESIAN_POINT('Ctrl Pts',(98.2721017199381,-0.687422303500887,
2.09537350556539));
#12158=CARTESIAN_POINT('Ctrl Pts',(98.2680908041532,-0.616311878717547,
2.11738064673258));
#12159=CARTESIAN_POINT('Ctrl Pts',(98.2640798883684,-0.544282841101875,
2.13573691939857));
#12160=CARTESIAN_POINT('Ctrl Pts',(98.2600690287855,-0.47225481277564,2.15409293485173));
#12161=CARTESIAN_POINT('Ctrl Pts',(98.2560581692025,-0.399308674593535,
2.16879807161835));
#12162=CARTESIAN_POINT('Ctrl Pts',(98.2520473096196,-0.325851804889479,
2.17977902578456));
#12163=CARTESIAN_POINT('Ctrl Pts',(98.2480331976153,-0.252335368727682,
2.19076888444867));
#12164=CARTESIAN_POINT('Ctrl Pts',(98.2440190856109,-0.178307861136477,
2.198028472553));
#12165=CARTESIAN_POINT('Ctrl Pts',(98.2400049736066,-0.104182596936714,
2.20153627871437));
#12166=CARTESIAN_POINT('Ctrl Pts',(98.2380882648744,-0.06878833264788,2.20321123015893));
#12167=CARTESIAN_POINT('Ctrl Pts',(98.2361715561422,-0.0333718065489038,
2.20403154496129));
#12168=CARTESIAN_POINT('Ctrl Pts',(98.23425484741,0.00202208561227388,2.20399907240674));
#12169=CARTESIAN_POINT('',(97.484254847371,-0.00067182755121702,2.20399989760611));
#12170=CARTESIAN_POINT('Ctrl Pts',(98.2342548473827,0.00202208611721571,
2.20399907240628));
#12171=CARTESIAN_POINT('Ctrl Pts',(98.2289277772449,0.100391620738078,2.20390882206416));
#12172=CARTESIAN_POINT('Ctrl Pts',(98.2236007071072,0.198467672311368,2.19722915975478));
#12173=CARTESIAN_POINT('Ctrl Pts',(98.2182736369695,0.295508944404814,2.18409946288551));
#12174=CARTESIAN_POINT('Ctrl Pts',(98.2139014280923,0.375155861064196,2.17332322459276));
#12175=CARTESIAN_POINT('Ctrl Pts',(98.2095292192152,0.454106399944636,2.15820294185027));
#12176=CARTESIAN_POINT('Ctrl Pts',(98.205157010338,0.531962637762755,2.138838879398));
#12177=CARTESIAN_POINT('Ctrl Pts',(98.2010839453725,0.604491998439037,2.12079969449621));
#12178=CARTESIAN_POINT('Ctrl Pts',(98.197010880407,0.676242606939927,2.0990322666232));
#12179=CARTESIAN_POINT('Ctrl Pts',(98.1929378154415,0.746802901210407,2.07362036707391));
#12180=CARTESIAN_POINT('Ctrl Pts',(98.188870734605,0.817259528608114,2.04824580257522));
#12181=CARTESIAN_POINT('Ctrl Pts',(98.1848036537686,0.88652886837879,2.01923755759146));
#12182=CARTESIAN_POINT('Ctrl Pts',(98.1807365729321,0.954211942849043,1.98672986792977));
#12183=CARTESIAN_POINT('Ctrl Pts',(98.1766742505292,1.02181582897173,1.95426021185696));
#12184=CARTESIAN_POINT('Ctrl Pts',(98.1726119281263,1.08783670883466,1.91829945123413));
#12185=CARTESIAN_POINT('Ctrl Pts',(98.1685496057233,1.15189465244276,1.87903025778559));
#12186=CARTESIAN_POINT('Ctrl Pts',(98.1644898615484,1.21591194049374,1.839785987256));
#12187=CARTESIAN_POINT('Ctrl Pts',(98.1604301173734,1.27796835844299,1.79723769955032));
#12188=CARTESIAN_POINT('Ctrl Pts',(98.1563703731984,1.33770890638433,1.75161379355726));
#12189=CARTESIAN_POINT('Ctrl Pts',(98.1523118937061,1.39743084408001,1.70600410022423));
#12190=CARTESIAN_POINT('Ctrl Pts',(98.1482534142138,1.45483796493468,1.65732098049386));
#12191=CARTESIAN_POINT('Ctrl Pts',(98.1441949347215,1.50960591474826,1.60583497974015));
#12192=CARTESIAN_POINT('Ctrl Pts',(98.1401364080503,1.56437450122625,1.55434838047393));
#12193=CARTESIAN_POINT('Ctrl Pts',(98.1360778813792,1.61650350909749,1.50005916382788));
#12194=CARTESIAN_POINT('Ctrl Pts',(98.132019354708,1.66570442019289,1.44327571328207));
#12195=CARTESIAN_POINT('Ctrl Pts',(98.127956677682,1.71495564541824,1.38643419450447));
#12196=CARTESIAN_POINT('Ctrl Pts',(98.123894000656,1.76127248096927,1.32709370993731));
#12197=CARTESIAN_POINT('Ctrl Pts',(98.11983132363,1.80440631920992,1.26559623703428));
#12198=CARTESIAN_POINT('Ctrl Pts',(98.1157665246109,1.84756268685913,1.20406664313878));
#12199=CARTESIAN_POINT('Ctrl Pts',(98.1117017255917,1.8875324924024,1.14037822213482));
#12200=CARTESIAN_POINT('Ctrl Pts',(98.1076369265725,1.92411161185864,1.07490023030547));
#12201=CARTESIAN_POINT('Ctrl Pts',(98.1035648662868,1.96075607544003,1.00930527004832));
#12202=CARTESIAN_POINT('Ctrl Pts',(98.0994928060011,1.99399754292445,0.941914782343538));
#12203=CARTESIAN_POINT('Ctrl Pts',(98.0954207457154,2.02367902148731,0.873120391465089));
#12204=CARTESIAN_POINT('Ctrl Pts',(98.0922825952499,2.04655317835997,0.820103703446003));
#12205=CARTESIAN_POINT('Ctrl Pts',(98.0891444447844,2.0673139948512,0.76625369991621));
#12206=CARTESIAN_POINT('Ctrl Pts',(98.0860062943188,2.08590996800986,0.711755298791019));
#12207=CARTESIAN_POINT('Ctrl Pts',(98.0819332295131,2.11004603306881,0.641020793855812));
#12208=CARTESIAN_POINT('Ctrl Pts',(98.0778601647074,2.13062658797387,0.568920787013463));
#12209=CARTESIAN_POINT('Ctrl Pts',(98.0737870999016,2.14749904921425,0.495846582749047));
#12210=CARTESIAN_POINT('Ctrl Pts',(98.0697200192292,2.16434672149054,0.42287973886312));
#12211=CARTESIAN_POINT('Ctrl Pts',(98.0656529385568,2.17749700991872,0.348942000603794));
#12212=CARTESIAN_POINT('Ctrl Pts',(98.0615858578843,2.18684656459241,0.274441438070829));
#12213=CARTESIAN_POINT('Ctrl Pts',(98.057523535651,2.19618518039122,0.200028040366577));
#12214=CARTESIAN_POINT('Ctrl Pts',(98.0534612134177,2.20173183808983,0.125053598038256));
#12215=CARTESIAN_POINT('Ctrl Pts',(98.0493988911844,2.20343421831169,0.0499364153015492));
#12216=CARTESIAN_POINT('Ctrl Pts',(98.0453391471823,2.20513551808505,-0.0251330928639777));
#12217=CARTESIAN_POINT('Ctrl Pts',(98.0412794031803,2.20299737119982,-0.100344685537534));
#12218=CARTESIAN_POINT('Ctrl Pts',(98.0372196591782,2.19701939932981,-0.175276236177271));
#12219=CARTESIAN_POINT('Ctrl Pts',(98.0331611798619,2.19104328970924,-0.250184444245087));
#12220=CARTESIAN_POINT('Ctrl Pts',(98.0291027005457,2.18122976800794,-0.324812307849021));
#12221=CARTESIAN_POINT('Ctrl Pts',(98.0250442212294,2.16763048424939,-0.39874062215023));
#12222=CARTESIAN_POINT('Ctrl Pts',(98.0209856947371,2.15403104241195,-0.472669795798605));
#12223=CARTESIAN_POINT('Ctrl Pts',(98.0169271682449,2.13664583928596,-0.545898934741146));
#12224=CARTESIAN_POINT('Ctrl Pts',(98.0128686417526,2.11557774430185,-0.618018452649033));
#12225=CARTESIAN_POINT('Ctrl Pts',(98.0088059649087,2.09448810455213,-0.690211721795935));
#12226=CARTESIAN_POINT('Ctrl Pts',(98.0047432880648,2.06970818620269,-0.761292644600529));
#12227=CARTESIAN_POINT('Ctrl Pts',(98.000680611221,2.04139071857128,-0.830866977398324));
#12228=CARTESIAN_POINT('Ctrl Pts',(97.996615812386,2.01305846034317,-0.900477649812031));
#12229=CARTESIAN_POINT('Ctrl Pts',(97.992551013551,1.98118517587959,-0.968579732315303));
#12230=CARTESIAN_POINT('Ctrl Pts',(97.988486214716,1.94597062435514,-1.03480158926573));
#12231=CARTESIAN_POINT('Ctrl Pts',(97.9844141546157,1.91069316634791,-1.1011417434519));
#12232=CARTESIAN_POINT('Ctrl Pts',(97.9803420945155,1.8720627649595,-1.16559455301516));
#12233=CARTESIAN_POINT('Ctrl Pts',(97.9762700344153,1.83032351616074,-1.22781587633855));
#12234=CARTESIAN_POINT('Ctrl Pts',(97.9731318823768,1.79815697011727,-1.27576702829188));
#12235=CARTESIAN_POINT('Ctrl Pts',(97.9699937303382,1.76414497408377,-1.32239343605571));
#12236=CARTESIAN_POINT('Ctrl Pts',(97.9668555782997,1.72841504534132,-1.36755161914926));
#12237=CARTESIAN_POINT('Ctrl Pts',(97.9627825133003,1.68204051650868,-1.42616325196266));
#12238=CARTESIAN_POINT('Ctrl Pts',(97.9587094483009,1.63259184260637,-1.48252635568421));
#12239=CARTESIAN_POINT('Ctrl Pts',(97.9546363833014,1.58031523996454,-1.53630066794746));
#12240=CARTESIAN_POINT('Ctrl Pts',(97.9505693024321,1.52811544188933,-1.58999597521537));
#12241=CARTESIAN_POINT('Ctrl Pts',(97.9465022215628,1.47309629406208,-1.64110970290096));
#12242=CARTESIAN_POINT('Ctrl Pts',(97.9424351406935,1.41554477998905,-1.6893338852476));
#12243=CARTESIAN_POINT('Ctrl Pts',(97.9383728182595,1.35806060048928,-1.73750164588594));
#12244=CARTESIAN_POINT('Ctrl Pts',(97.9343104958254,1.29805030535379,-1.78278627281644));
#12245=CARTESIAN_POINT('Ctrl Pts',(97.9302481733914,1.23583712918931,-1.82491714609654));
#12246=CARTESIAN_POINT('Ctrl Pts',(97.9261884291864,1.17366343778255,-1.86702128022864));
#12247=CARTESIAN_POINT('Ctrl Pts',(97.9221286849814,1.10929003406122,-1.90597536560161));
#12248=CARTESIAN_POINT('Ctrl Pts',(97.9180689407764,1.0430715079989,-1.94155036741283));
#12249=CARTESIAN_POINT('Ctrl Pts',(97.9140104612552,0.976873610206266,-1.97711428696694));
#12250=CARTESIAN_POINT('Ctrl Pts',(97.909951981734,0.908832151622473,-2.00930098712529));
#12251=CARTESIAN_POINT('Ctrl Pts',(97.9058935022128,0.839327456571355,-2.03792674565242));
#12252=CARTESIAN_POINT('Ctrl Pts',(97.901834975514,0.769821953564913,-2.06655283693885));
#12253=CARTESIAN_POINT('Ctrl Pts',(97.8977764488151,0.698853622484897,-2.09161772423588));
#12254=CARTESIAN_POINT('Ctrl Pts',(97.8937179221163,0.626822455076543,-2.11298594643027));
#12255=CARTESIAN_POINT('Ctrl Pts',(97.8896552450646,0.554717626761799,-2.13437602031291));
#12256=CARTESIAN_POINT('Ctrl Pts',(97.885592568013,0.481548250435302,-2.15206174394929));
#12257=CARTESIAN_POINT('Ctrl Pts',(97.8815298909614,0.40772843753002,-2.16595787614379));
#12258=CARTESIAN_POINT('Ctrl Pts',(97.8774650919177,0.333870067521403,-2.17986126647922));
#12259=CARTESIAN_POINT('Ctrl Pts',(97.8734002928739,0.259361057956396,-2.18997105942271));
#12260=CARTESIAN_POINT('Ctrl Pts',(97.8693354938302,0.184622000096624,-2.19625379159156));
#12261=CARTESIAN_POINT('Ctrl Pts',(97.8652634335221,0.109749430086021,-2.20254774709008));
#12262=CARTESIAN_POINT('Ctrl Pts',(97.8611913732139,0.0346464688482193,
-2.20500097067697));
#12263=CARTESIAN_POINT('Ctrl Pts',(97.8571193129057,-0.0402653783392436,
-2.20363216061738));
#12264=CARTESIAN_POINT('Ctrl Pts',(97.8539811626974,-0.0979965048629268,
-2.20257728145334));
#12265=CARTESIAN_POINT('Ctrl Pts',(97.850843012489,-0.155614094320053,-2.19925354133635));
#12266=CARTESIAN_POINT('Ctrl Pts',(97.8477048622806,-0.21292846106124,-2.19369037707469));
#12267=CARTESIAN_POINT('Ctrl Pts',(97.8436317973462,-0.287317869440097,
-2.18646984020636));
#12268=CARTESIAN_POINT('Ctrl Pts',(97.8395587324119,-0.36148303709724,-2.17544720311697));
#12269=CARTESIAN_POINT('Ctrl Pts',(97.8354856674776,-0.435004570433692,
-2.16064504805898));
#12270=CARTESIAN_POINT('Ctrl Pts',(97.8314185866741,-0.508418086226198,
-2.14586464026825));
#12271=CARTESIAN_POINT('Ctrl Pts',(97.8273515058705,-0.581189380966512,
-2.12731583264171));
#12272=CARTESIAN_POINT('Ctrl Pts',(97.823284425067,-0.65290411767467,-2.10507297097356));
#12273=CARTESIAN_POINT('Ctrl Pts',(97.8192221026994,-0.724534948997614,
-2.08285613318785));
#12274=CARTESIAN_POINT('Ctrl Pts',(97.8151597803318,-0.795111224518574,
-2.05695396891655));
#12275=CARTESIAN_POINT('Ctrl Pts',(97.8110974579642,-0.864230354606361,
-2.02749152752286));
#12276=CARTESIAN_POINT('Ctrl Pts',(97.807037713826,-0.933305616936154,-1.99804778502262));
#12277=CARTESIAN_POINT('Ctrl Pts',(97.8029779696879,-1.00092513089808,-1.96504843607286));
#12278=CARTESIAN_POINT('Ctrl Pts',(97.7989182255497,-1.06670426994776,-1.92866741572393));
#12279=CARTESIAN_POINT('Ctrl Pts',(97.7948597460956,-1.13246291759979,-1.89229772872422));
#12280=CARTESIAN_POINT('Ctrl Pts',(97.7908012666416,-1.19638191108074,-1.85254869284278));
#12281=CARTESIAN_POINT('Ctrl Pts',(97.7867427871875,-1.25810076539643,-1.80964042398177));
#12282=CARTESIAN_POINT('Ctrl Pts',(97.7826842605559,-1.31982033715831,-1.76673165633681));
#12283=CARTESIAN_POINT('Ctrl Pts',(97.7786257339244,-1.37933932796847,-1.72066385681412));
#12284=CARTESIAN_POINT('Ctrl Pts',(97.7745672072928,-1.43632715981332,-1.67169982053675));
#12285=CARTESIAN_POINT('Ctrl Pts',(97.7705045303083,-1.49337326886991,-1.62268571238584));
#12286=CARTESIAN_POINT('Ctrl Pts',(97.7664418533238,-1.54788268706758,-1.57076976485147));
#12287=CARTESIAN_POINT('Ctrl Pts',(97.7623791763393,-1.59955939560565,-1.51625385075511));
#12288=CARTESIAN_POINT('Ctrl Pts',(97.7583143773627,-1.6512630955995,-1.46170946224685));
#12289=CARTESIAN_POINT('Ctrl Pts',(97.7542495783862,-1.7001308289334,-1.40456276606914));
#12290=CARTESIAN_POINT('Ctrl Pts',(97.7501847794096,-1.74590658485429,-1.34514913558401));
#12291=CARTESIAN_POINT('Ctrl Pts',(97.7461127191678,-1.7917641135529,-1.28562936992972));
#12292=CARTESIAN_POINT('Ctrl Pts',(97.742040658926,-1.83451836013391,-1.2238349744318));
#12293=CARTESIAN_POINT('Ctrl Pts',(97.7379685986842,-1.87395666017458,-1.16013035292907));
#12294=CARTESIAN_POINT('Ctrl Pts',(97.7348304478766,-1.90434995638714,-1.11103611130495));
#12295=CARTESIAN_POINT('Ctrl Pts',(97.731692297069,-1.93277477065016,-1.06080798103647));
#12296=CARTESIAN_POINT('Ctrl Pts',(97.7285541462614,-1.95915306880777,-1.00962134138553));
#12297=CARTESIAN_POINT('Ctrl Pts',(97.7244810813405,-1.99338995781841,-0.943185239629218));
#12298=CARTESIAN_POINT('Ctrl Pts',(97.7204080164196,-2.02430970542024,-0.874877554951377));
#12299=CARTESIAN_POINT('Ctrl Pts',(97.7163349514987,-2.05170405580196,-0.805063020766566));
#12300=CARTESIAN_POINT('Ctrl Pts',(97.712267870709,-2.07905815851011,-0.7353510578252));
#12301=CARTESIAN_POINT('Ctrl Pts',(97.7082007899193,-2.10289697446296,-0.664137081565813));
#12302=CARTESIAN_POINT('Ctrl Pts',(97.7041337091296,-2.12305849458596,-0.591809621894051));
#12303=CARTESIAN_POINT('Ctrl Pts',(97.7000713867765,-2.14319642596823,-0.519566784496978));
#12304=CARTESIAN_POINT('Ctrl Pts',(97.6960090644233,-2.15966548183138,-0.446213509594031));
#12305=CARTESIAN_POINT('Ctrl Pts',(97.6919467420702,-2.17235263411151,-0.372155925747258));
#12306=CARTESIAN_POINT('Ctrl Pts',(97.6878869979468,-2.18503173425028,-0.298145343947892));
#12307=CARTESIAN_POINT('Ctrl Pts',(97.6838272538235,-2.19393361343885,-0.223431809645988));
#12308=CARTESIAN_POINT('Ctrl Pts',(97.6797675097001,-2.19899606451928,-0.148432840802502));
#12309=CARTESIAN_POINT('Ctrl Pts',(97.6757090302612,-2.20405693855375,-0.0734572355075946));
#12310=CARTESIAN_POINT('Ctrl Pts',(97.6716505508223,-2.20528072705553,0.00180315171998274));
#12311=CARTESIAN_POINT('Ctrl Pts',(97.6675920713834,-2.20265711799268,0.0769260720184203));
#12312=CARTESIAN_POINT('Ctrl Pts',(97.6635335447673,-2.20003347843209,0.152049865571672));
#12313=CARTESIAN_POINT('Ctrl Pts',(97.6594750181512,-2.19356237096343,0.227035711915739));
#12314=CARTESIAN_POINT('Ctrl Pts',(97.6554164915351,-2.18328555940878,0.301463374354331));
#12315=CARTESIAN_POINT('Ctrl Pts',(97.6513538145665,-2.1729982385252,0.375967148413867));
#12316=CARTESIAN_POINT('Ctrl Pts',(97.6472911375978,-2.1588975072858,0.449911124662818));
#12317=CARTESIAN_POINT('Ctrl Pts',(97.6432284606292,-2.14107669898293,0.522882940123679));
#12318=CARTESIAN_POINT('Ctrl Pts',(97.6391636616687,-2.12324658262773,0.595892869763449));
#12319=CARTESIAN_POINT('Ctrl Pts',(97.6350988627082,-2.10169265681259,0.667929169585409));
#12320=CARTESIAN_POINT('Ctrl Pts',(97.6310340637477,-2.07655808902178,0.738594951863493));
#12321=CARTESIAN_POINT('Ctrl Pts',(97.6269620035222,-2.05137862140724,0.809386969897618));
#12322=CARTESIAN_POINT('Ctrl Pts',(97.6228899432968,-2.02260591864279,0.87880313844883));
#12323=CARTESIAN_POINT('Ctrl Pts',(97.6188178830713,-1.99043103409202,0.946467272822127));
#12324=CARTESIAN_POINT('Ctrl Pts',(97.6156797321283,-1.96563531921958,0.998612932594857));
#12325=CARTESIAN_POINT('Ctrl Pts',(97.6125415811853,-1.93882001339638,1.04971845874858));
#12326=CARTESIAN_POINT('Ctrl Pts',(97.6094034302423,-1.91009024138284,1.09962323992086));
#12327=CARTESIAN_POINT('Ctrl Pts',(97.6053303652977,-1.87280133164568,1.1643955910453));
#12328=CARTESIAN_POINT('Ctrl Pts',(97.6012573003531,-1.83214207195564,1.22739396603369));
#12329=CARTESIAN_POINT('Ctrl Pts',(97.5971842354084,-1.78830618136827,1.28824570702954));
#12330=CARTESIAN_POINT('Ctrl Pts',(97.5931171545946,-1.74453469429696,1.3490080448896));
#12331=CARTESIAN_POINT('Ctrl Pts',(97.5890500737809,-1.69759611917393,1.40762962619744));
#12332=CARTESIAN_POINT('Ctrl Pts',(97.584982992967,-1.64772923329867,1.46376376978424));
#12333=CARTESIAN_POINT('Ctrl Pts',(97.5809206705893,-1.59792069108524,1.51983223709243));
#12334=CARTESIAN_POINT('Ctrl Pts',(97.5768583482115,-1.54519096048288,1.57341869356677));
#12335=CARTESIAN_POINT('Ctrl Pts',(97.5727960258338,-1.4898201492766,1.6242080909814));
#12336=CARTESIAN_POINT('Ctrl Pts',(97.5687362816855,-1.43448448019958,1.6749652539474));
#12337=CARTESIAN_POINT('Ctrl Pts',(97.5646765375372,-1.37651140774591,1.72292855863136));
#12338=CARTESIAN_POINT('Ctrl Pts',(97.560616793389,-1.31621814823417,1.76781950047481));
#12339=CARTESIAN_POINT('Ctrl Pts',(97.5565583139249,-1.25594367117006,1.8126964579729));
#12340=CARTESIAN_POINT('Ctrl Pts',(97.5524998344608,-1.19335082481708,1.85450266795433));
#12341=CARTESIAN_POINT('Ctrl Pts',(97.5484413549967,-1.1287889196328,1.89300068011457));
#12342=CARTESIAN_POINT('Ctrl Pts',(97.5443828283553,-1.06422626395504,1.93149913979115));
#12343=CARTESIAN_POINT('Ctrl Pts',(97.5403243017138,-0.997694915004834,
1.96668908229734));
#12344=CARTESIAN_POINT('Ctrl Pts',(97.5362657750723,-0.929570707792732,
1.99837791701513));
#12345=CARTESIAN_POINT('Ctrl Pts',(97.5322030980781,-0.861376835031043,
2.03009915754249));
#12346=CARTESIAN_POINT('Ctrl Pts',(97.5281404210839,-0.791587285070047,
2.05831193875905));
#12347=CARTESIAN_POINT('Ctrl Pts',(97.5240777440897,-0.720599216502606,
2.08287128003049));
#12348=CARTESIAN_POINT('Ctrl Pts',(97.5200129451035,-0.649574069892286,
2.10744344898306));
#12349=CARTESIAN_POINT('Ctrl Pts',(97.5159481461174,-0.577349617097396,
2.12835824498218));
#12350=CARTESIAN_POINT('Ctrl Pts',(97.5118833471312,-0.504337011039581,
2.14552095755219));
#12351=CARTESIAN_POINT('Ctrl Pts',(97.5078112868801,-0.431193976914977,
2.16271432920345));
#12352=CARTESIAN_POINT('Ctrl Pts',(97.503739226629,-0.357260447751076,2.17614214398164));
#12353=CARTESIAN_POINT('Ctrl Pts',(97.499667166378,-0.282956121244091,2.18576115654261));
#12354=CARTESIAN_POINT('Ctrl Pts',(97.4965290156597,-0.225693172952624,
2.19317408987755));
#12355=CARTESIAN_POINT('Ctrl Pts',(97.4933908649415,-0.168210195148379,
2.1983260032933));
#12356=CARTESIAN_POINT('Ctrl Pts',(97.4902527142232,-0.110699139461686,
2.2012182310081));
#12357=CARTESIAN_POINT('Ctrl Pts',(97.4882534252855,-0.074059338587481,
2.20306084450716));
#12358=CARTESIAN_POINT('Ctrl Pts',(97.4862541363478,-0.0373731498197366,
2.20398871022549));
#12359=CARTESIAN_POINT('Ctrl Pts',(97.48425484741,-0.000671828267138261,
2.20399989760589));
#12360=CARTESIAN_POINT('',(96.7342548474632,-0.00162714762935965,2.20399939936258));
#12361=CARTESIAN_POINT('Ctrl Pts',(97.484254847371,-0.000671827551214084,
2.20399989760611));
#12362=CARTESIAN_POINT('Ctrl Pts',(97.4802137118767,0.0735120537378061,
2.20402251048162));
#12363=CARTESIAN_POINT('Ctrl Pts',(97.4761725763824,0.147847596217428,2.20029545639483));
#12364=CARTESIAN_POINT('Ctrl Pts',(97.472131440888,0.221920597882872,2.19279895299029));
#12365=CARTESIAN_POINT('Ctrl Pts',(97.4679218807762,0.299080780611764,2.18499001370719));
#12366=CARTESIAN_POINT('Ctrl Pts',(97.4637123206643,0.375955535407559,2.17309042861314));
#12367=CARTESIAN_POINT('Ctrl Pts',(97.4595027605525,0.452074506096688,2.15713806719399));
#12368=CARTESIAN_POINT('Ctrl Pts',(97.4554719719984,0.524960857081313,2.14186317050394));
#12369=CARTESIAN_POINT('Ctrl Pts',(97.4514411834444,0.597153779759007,2.12287284391787));
#12370=CARTESIAN_POINT('Ctrl Pts',(97.4474103948903,0.66824595962738,2.10025316032179));
#12371=CARTESIAN_POINT('Ctrl Pts',(97.4433818694975,0.739298223468306,2.07764617696803));
#12372=CARTESIAN_POINT('Ctrl Pts',(97.4393533441046,0.809250508664425,2.05141402580155));
#12373=CARTESIAN_POINT('Ctrl Pts',(97.4353248187118,0.87770894713221,2.0216931033478));
#12374=CARTESIAN_POINT('Ctrl Pts',(97.4312972029413,0.946151928001575,1.99197889174073));
#12375=CARTESIAN_POINT('Ctrl Pts',(97.4272695871709,1.01310128658206,1.95877766627834));
#12376=CARTESIAN_POINT('Ctrl Pts',(97.4232419714004,1.07818310152526,1.92227396579816));
#12377=CARTESIAN_POINT('Ctrl Pts',(97.4192139130876,1.14327206746455,1.88576625440003));
#12378=CARTESIAN_POINT('Ctrl Pts',(97.4151858547747,1.2064926603659,1.84595558777702));
#12379=CARTESIAN_POINT('Ctrl Pts',(97.4111577964618,1.26749705217653,1.80307160776377));
#12380=CARTESIAN_POINT('Ctrl Pts',(97.4071254264789,1.32856674363935,1.76014172435084));
#12381=CARTESIAN_POINT('Ctrl Pts',(97.403093056496,1.38741510392216,1.71413224480025));
#12382=CARTESIAN_POINT('Ctrl Pts',(97.3990606865131,1.44372549513439,1.66531459331231));
#12383=CARTESIAN_POINT('Ctrl Pts',(97.3950257630346,1.50007154486423,1.6164660280792));
#12384=CARTESIAN_POINT('Ctrl Pts',(97.3909908395561,1.55387607957638,1.56480609054044));
#12385=CARTESIAN_POINT('Ctrl Pts',(97.3869559160777,1.60485955438531,1.51064284683646));
#12386=CARTESIAN_POINT('Ctrl Pts',(97.382914382503,1.65592655139059,1.45639087177213));
#12387=CARTESIAN_POINT('Ctrl Pts',(97.3788728489284,1.70416295767579,1.39962778046808));
#12388=CARTESIAN_POINT('Ctrl Pts',(97.3748313153537,1.74933026441019,1.34069371074029));
#12389=CARTESIAN_POINT('Ctrl Pts',(97.3735882096371,1.76322294553387,1.32256661179982));
#12390=CARTESIAN_POINT('Ctrl Pts',(97.3723451039206,1.77682558613733,1.30423431700571));
#12391=CARTESIAN_POINT('Ctrl Pts',(97.371101998204,1.79013210898306,1.28570721098851));
#12392=CARTESIAN_POINT('Ctrl Pts',(97.3670289332697,1.83373124208839,1.22500271510592));
#12393=CARTESIAN_POINT('Ctrl Pts',(97.3629558683354,1.87432316218437,1.16196093021885));
#12394=CARTESIAN_POINT('Ctrl Pts',(97.3588828034011,1.91164843376739,1.09691215039068));
#12395=CARTESIAN_POINT('Ctrl Pts',(97.3548157225978,1.94891886720835,1.03195893997371));
#12396=CARTESIAN_POINT('Ctrl Pts',(97.3507486417945,1.98293194514319,0.965004999616546));
#12397=CARTESIAN_POINT('Ctrl Pts',(97.3466815609911,2.01347049427321,0.896410937400477));
#12398=CARTESIAN_POINT('Ctrl Pts',(97.342619238624,2.04397331366349,0.827897129422442));
#12399=CARTESIAN_POINT('Ctrl Pts',(97.3385569162569,2.07100948757194,0.757747446041395));
#12400=CARTESIAN_POINT('Ctrl Pts',(97.3344945938898,2.09440771754225,0.686347078889013));
#12401=CARTESIAN_POINT('Ctrl Pts',(97.3304348497523,2.11779109738413,0.61499202732774));
#12402=CARTESIAN_POINT('Ctrl Pts',(97.3263751056148,2.13754096672106,0.542388319715484));
#12403=CARTESIAN_POINT('Ctrl Pts',(97.3223153614773,2.15353463151827,0.468939858458917));
#12404=CARTESIAN_POINT('Ctrl Pts',(97.318256882024,2.16952331399747,0.395514277736344));
#12405=CARTESIAN_POINT('Ctrl Pts',(97.3141984025708,2.18175801365045,0.321244932078565));
#12406=CARTESIAN_POINT('Ctrl Pts',(97.3101399231176,2.19016667883116,0.246548005341155));
#12407=CARTESIAN_POINT('Ctrl Pts',(97.306081396487,2.19857544175739,0.171850210298192));
#12408=CARTESIAN_POINT('Ctrl Pts',(97.3020228698564,2.20315803027515,0.0967252989712811));
#12409=CARTESIAN_POINT('Ctrl Pts',(97.2979643432259,2.20389420162738,0.0215950928043276));
#12410=CARTESIAN_POINT('Ctrl Pts',(97.2939016662426,2.20463112580718,-0.0536119434247664));
#12411=CARTESIAN_POINT('Ctrl Pts',(97.2898389892594,2.2015137732694,-0.128823806808176));
#12412=CARTESIAN_POINT('Ctrl Pts',(97.2857763122762,2.19457406782218,-0.203618910817236));
#12413=CARTESIAN_POINT('Ctrl Pts',(97.281711513301,2.18763073767159,-0.278453081335427));
#12414=CARTESIAN_POINT('Ctrl Pts',(97.2776467143258,2.1768611472908,-0.352869586014872));
#12415=CARTESIAN_POINT('Ctrl Pts',(97.2735819153506,2.16234878396153,-0.426454846965158));
#12416=CARTESIAN_POINT('Ctrl Pts',(97.2695098551105,2.14781049607461,-0.500171558961478));
#12417=CARTESIAN_POINT('Ctrl Pts',(97.2654377948703,2.12951619687854,-0.573053597444631));
#12418=CARTESIAN_POINT('Ctrl Pts',(97.2613657346302,2.10759977559415,-0.644700849941666));
#12419=CARTESIAN_POINT('Ctrl Pts',(97.2582275838151,2.09070979085379,-0.69991611459003));
#12420=CARTESIAN_POINT('Ctrl Pts',(97.255089433,2.071669640917,-0.754398293751397));
#12421=CARTESIAN_POINT('Ctrl Pts',(97.2519512821849,2.05055979033752,-0.807973109856357));
#12422=CARTESIAN_POINT('Ctrl Pts',(97.2478782172477,2.02316091842555,-0.877508870833944));
#12423=CARTESIAN_POINT('Ctrl Pts',(97.2438051523106,1.99216819889427,-0.945783477852407));
#12424=CARTESIAN_POINT('Ctrl Pts',(97.2397320873735,1.95771867451018,-1.01239991676911));
#12425=CARTESIAN_POINT('Ctrl Pts',(97.2356650065672,1.92331976323126,-1.07891848307687));
#12426=CARTESIAN_POINT('Ctrl Pts',(97.231597925761,1.8854743479383,-1.14378329749517));
#12427=CARTESIAN_POINT('Ctrl Pts',(97.2275308449548,1.84436784868453,-1.20661644226275));
#12428=CARTESIAN_POINT('Ctrl Pts',(97.2234685225848,1.80330944354594,-1.26937607299831));
#12429=CARTESIAN_POINT('Ctrl Pts',(97.2194062002147,1.75899779491425,-1.33010835915344));
#12430=CARTESIAN_POINT('Ctrl Pts',(97.2153438778446,1.71166384110568,-1.388460620634));
#12431=CARTESIAN_POINT('Ctrl Pts',(97.2112841337041,1.66435992868409,-1.4467758477507));
#12432=CARTESIAN_POINT('Ctrl Pts',(97.2072243895636,1.6140378174979,-1.5027136778072));
#12433=CARTESIAN_POINT('Ctrl Pts',(97.2031646454231,1.56097050703468,-1.55595214456226));
#12434=CARTESIAN_POINT('Ctrl Pts',(97.1991061659669,1.50791972800526,-1.60917402656522));
#12435=CARTESIAN_POINT('Ctrl Pts',(97.1950476865106,1.45212578447304,-1.65969787690115));
#12436=CARTESIAN_POINT('Ctrl Pts',(97.1909892070544,1.39389943749807,-1.70723763962214));
#12437=CARTESIAN_POINT('Ctrl Pts',(97.1869306804208,1.33567241367731,-1.75477795496389));
#12438=CARTESIAN_POINT('Ctrl Pts',(97.1828721537871,1.27501330125152,-1.79933381323925));
#12439=CARTESIAN_POINT('Ctrl Pts',(97.1788136271535,1.21226567076068,-1.84065964901042));
#12440=CARTESIAN_POINT('Ctrl Pts',(97.1747509501672,1.14945387294469,-1.88202774563384));
#12441=CARTESIAN_POINT('Ctrl Pts',(97.1706882731809,1.08454969168412,-1.92015896044332));
#12442=CARTESIAN_POINT('Ctrl Pts',(97.1666255961946,1.01792476498994,-1.95485170097892));
#12443=CARTESIAN_POINT('Ctrl Pts',(97.1625607972163,0.95126503918211,-1.98956256200907));
#12444=CARTESIAN_POINT('Ctrl Pts',(97.1584959982381,0.882883212752135,-2.02083117354383));
#12445=CARTESIAN_POINT('Ctrl Pts',(97.1544311992598,0.81317213064539,-2.04850362116879));
#12446=CARTESIAN_POINT('Ctrl Pts',(97.1503591390166,0.74333651823827,-2.0762255022283));
#12447=CARTESIAN_POINT('Ctrl Pts',(97.1462870787733,0.672167360052406,-2.10033823428516));
#12448=CARTESIAN_POINT('Ctrl Pts',(97.1422150185301,0.600073492233046,-2.12073756130249));
#12449=CARTESIAN_POINT('Ctrl Pts',(97.139076867742,0.544514042076541,-2.13645839064523));
#12450=CARTESIAN_POINT('Ctrl Pts',(97.1359387169538,0.488405742393722,-2.14997481786457));
#12451=CARTESIAN_POINT('Ctrl Pts',(97.1328005661657,0.431938669814331,-2.16126004578788));
#12452=CARTESIAN_POINT('Ctrl Pts',(97.1287275012299,0.358648994181453,-2.17590735538197));
#12453=CARTESIAN_POINT('Ctrl Pts',(97.1246544362941,0.284472090730599,-2.18685073776327));
#12454=CARTESIAN_POINT('Ctrl Pts',(97.1205813713583,0.209815900133298,-2.19399026617058));
#12455=CARTESIAN_POINT('Ctrl Pts',(97.1165142905535,0.135269394116645,-2.20111930521093));
#12456=CARTESIAN_POINT('Ctrl Pts',(97.1124472097486,0.0602454703586018,
-2.20445554086714));
#12457=CARTESIAN_POINT('Ctrl Pts',(97.1083801289437,-0.0148377690601739,
-2.20395005401877));
#12458=CARTESIAN_POINT('Ctrl Pts',(97.1043178065751,-0.0898331619814498,
-2.20344515858399));
#12459=CARTESIAN_POINT('Ctrl Pts',(97.1002554842064,-0.164887257633621,
-2.19910747392425));
#12460=CARTESIAN_POINT('Ctrl Pts',(97.0961931618377,-0.239578503319732,
-2.19094001304168));
#12461=CARTESIAN_POINT('Ctrl Pts',(97.0921334176986,-0.314222344797098,
-2.18277773579231));
#12462=CARTESIAN_POINT('Ctrl Pts',(97.0880736735595,-0.388503319864604,
-2.17079055743129));
#12463=CARTESIAN_POINT('Ctrl Pts',(97.0840139294204,-0.462002901034642,
-2.15503348452769));
#12464=CARTESIAN_POINT('Ctrl Pts',(97.0799554499655,-0.535479585746291,
-2.13928132023934));
#12465=CARTESIAN_POINT('Ctrl Pts',(97.0758969705107,-0.608174893309045,
-2.11976169313124));
#12466=CARTESIAN_POINT('Ctrl Pts',(97.0718384910558,-0.679680018633716,
-2.09658080508958));
#12467=CARTESIAN_POINT('Ctrl Pts',(97.0677799644236,-0.751185975161896,
-2.07339964758422));
#12468=CARTESIAN_POINT('Ctrl Pts',(97.0637214377914,-0.821501268344636,
-2.0465572935882));
#12469=CARTESIAN_POINT('Ctrl Pts',(97.0596629111592,-0.890233348282234,
-2.01620945975516));
#12470=CARTESIAN_POINT('Ctrl Pts',(97.0556002341743,-0.959035715395272,
-1.98583059145434));
#12471=CARTESIAN_POINT('Ctrl Pts',(97.0515375571894,-1.02625119839503,-1.95193927797258));
#12472=CARTESIAN_POINT('Ctrl Pts',(97.0474748802044,-1.09150899888306,-1.91473865197246));
#12473=CARTESIAN_POINT('Ctrl Pts',(97.0434100812276,-1.15680088441586,-1.87751859557485));
#12474=CARTESIAN_POINT('Ctrl Pts',(97.0393452822508,-1.22013264865409,-1.83698604213826));
#12475=CARTESIAN_POINT('Ctrl Pts',(97.0352804832739,-1.28116207596802,-1.79338778157467));
#12476=CARTESIAN_POINT('Ctrl Pts',(97.0312084230321,-1.34230052487086,-1.74971163806429));
#12477=CARTESIAN_POINT('Ctrl Pts',(97.0271363627902,-1.40112804741936,-1.70295914603113));
#12478=CARTESIAN_POINT('Ctrl Pts',(97.0230643025484,-1.45733550120218,-1.65341744182641));
#12479=CARTESIAN_POINT('Ctrl Pts',(97.0199261517478,-1.50065201805453,-1.61523791365619));
#12480=CARTESIAN_POINT('Ctrl Pts',(97.0167880009472,-1.54241312561684,-1.57540269030054));
#12481=CARTESIAN_POINT('Ctrl Pts',(97.0136498501466,-1.58249331359919,-1.53405701080952));
#12482=CARTESIAN_POINT('Ctrl Pts',(97.0095767852108,-1.63451414327371,-1.48039367590884));
#12483=CARTESIAN_POINT('Ctrl Pts',(97.005503720275,-1.68390256182177,-1.42397776736522));
#12484=CARTESIAN_POINT('Ctrl Pts',(97.0014306553391,-1.73035355074903,-1.36509801457999));
#12485=CARTESIAN_POINT('Ctrl Pts',(96.9973635745343,-1.77673629406656,-1.30630476769532));
#12486=CARTESIAN_POINT('Ctrl Pts',(96.9932964937294,-1.82018988283804,-1.2450552352296));
#12487=CARTESIAN_POINT('Ctrl Pts',(96.9892294129245,-1.86044666453567,-1.18167432417655));
#12488=CARTESIAN_POINT('Ctrl Pts',(96.9851670905559,-1.90065634627732,-1.11836756803592));
#12489=CARTESIAN_POINT('Ctrl Pts',(96.9811047681872,-1.93767639721694,-1.05293478870622));
#12490=CARTESIAN_POINT('Ctrl Pts',(96.9770424458185,-1.9712809438603,-0.985731931294325));
#12491=CARTESIAN_POINT('Ctrl Pts',(96.9729827016794,-2.00486416274382,-0.918571725444404));
#12492=CARTESIAN_POINT('Ctrl Pts',(96.9689229575403,-2.03503596592421,-0.849644096768522));
#12493=CARTESIAN_POINT('Ctrl Pts',(96.9648632134011,-2.06161581931966,-0.779330618884511));
#12494=CARTESIAN_POINT('Ctrl Pts',(96.9608047339463,-2.08818739260662,-0.709039044929665));
#12495=CARTESIAN_POINT('Ctrl Pts',(96.9567462544914,-2.11116906903231,-0.637362925246967));
#12496=CARTESIAN_POINT('Ctrl Pts',(96.9526877750366,-2.13042861167752,-0.564703400508454));
#12497=CARTESIAN_POINT('Ctrl Pts',(96.9486292484044,-2.14968837820304,-0.492043031147718));
#12498=CARTESIAN_POINT('Ctrl Pts',(96.9445707217722,-2.16522580443817,-0.418399696015615));
#12499=CARTESIAN_POINT('Ctrl Pts',(96.94051219514,-2.17695907773433,-0.344187701509047));
#12500=CARTESIAN_POINT('Ctrl Pts',(96.9364495181551,-2.18870434977464,-0.269899815926551));
#12501=CARTESIAN_POINT('Ctrl Pts',(96.9323868411702,-2.19663762559302,-0.195042582346671));
#12502=CARTESIAN_POINT('Ctrl Pts',(96.9283241641853,-2.2007287308317,-0.120037716122496));
#12503=CARTESIAN_POINT('Ctrl Pts',(96.9242593652085,-2.20482197291079,-0.0449936738274561));
#12504=CARTESIAN_POINT('Ctrl Pts',(96.9201945662316,-2.20506904645644,0.0301976767676627));
#12505=CARTESIAN_POINT('Ctrl Pts',(96.9161297672548,-2.20149195750705,0.105114989567421));
#12506=CARTESIAN_POINT('Ctrl Pts',(96.912057707013,-2.19790847852686,0.18016613296061));
#12507=CARTESIAN_POINT('Ctrl Pts',(96.9079856467712,-2.19048723909058,0.254941784918909));
#12508=CARTESIAN_POINT('Ctrl Pts',(96.9039135865294,-2.1793020759338,0.329026536666328));
#12509=CARTESIAN_POINT('Ctrl Pts',(96.9007754357287,-2.17068218167106,0.386120270355525));
#12510=CARTESIAN_POINT('Ctrl Pts',(96.8976372849281,-2.15982793250988,0.442803781184796));
#12511=CARTESIAN_POINT('Ctrl Pts',(96.8944991341274,-2.14679339697907,0.498892884983425));
#12512=CARTESIAN_POINT('Ctrl Pts',(96.8904260691913,-2.12987562820314,0.57169198754225));
#12513=CARTESIAN_POINT('Ctrl Pts',(96.8863530042551,-2.10921804283281,0.643769964700029));
#12514=CARTESIAN_POINT('Ctrl Pts',(96.882279939319,-2.08489805097604,0.714714010661834));
#12515=CARTESIAN_POINT('Ctrl Pts',(96.8782128585138,-2.06061378995533,0.78555382591126));
#12516=CARTESIAN_POINT('Ctrl Pts',(96.8741457777086,-2.03267795906397,0.855262569679648));
#12517=CARTESIAN_POINT('Ctrl Pts',(96.8700786969034,-2.00121862111457,0.923439240288346));
#12518=CARTESIAN_POINT('Ctrl Pts',(96.8660163745344,-1.9697960902165,0.991536145003068));
#12519=CARTESIAN_POINT('Ctrl Pts',(96.8619540521654,-1.934858441693,1.05810410650828));
#12520=CARTESIAN_POINT('Ctrl Pts',(96.8578917297963,-1.89658246244903,1.12276042107423));
#12521=CARTESIAN_POINT('Ctrl Pts',(96.8538319856569,-1.85833077577774,1.18737570028976));
#12522=CARTESIAN_POINT('Ctrl Pts',(96.8497722415174,-1.81674520539716,1.25008133033255));
#12523=CARTESIAN_POINT('Ctrl Pts',(96.845712497378,-1.77204864465173,1.31051882893302));
#12524=CARTESIAN_POINT('Ctrl Pts',(96.8416540179228,-1.72736600769908,1.37093750015187));
#12525=CARTESIAN_POINT('Ctrl Pts',(96.8375955384676,-1.67957458826537,1.4290890591465));
#12526=CARTESIAN_POINT('Ctrl Pts',(96.8335370590124,-1.62893989408494,1.48464501530115));
#12527=CARTESIAN_POINT('Ctrl Pts',(96.8294785323798,-1.57830461130708,1.5402016172599));
#12528=CARTESIAN_POINT('Ctrl Pts',(96.8254200057472,-1.52482631110719,1.59316220479494));
#12529=CARTESIAN_POINT('Ctrl Pts',(96.8213614791147,-1.46880888784006,1.64323353513797));
#12530=CARTESIAN_POINT('Ctrl Pts',(96.8172988021294,-1.41273417972928,1.69335606969862));
#12531=CARTESIAN_POINT('Ctrl Pts',(96.8132361251442,-1.35411552011598,1.74058312794341));
#12532=CARTESIAN_POINT('Ctrl Pts',(96.8091734481589,-1.29329100922578,1.78466085446389));
#12533=CARTESIAN_POINT('Ctrl Pts',(96.8051086491817,-1.23243472885871,1.82876160338589));
#12534=CARTESIAN_POINT('Ctrl Pts',(96.8010438502045,-1.16937070365075,1.86970948459025));
#12535=CARTESIAN_POINT('Ctrl Pts',(96.7969790512273,-1.10446499587837,1.90729470006064));
#12536=CARTESIAN_POINT('Ctrl Pts',(96.7929069909851,-1.03944334201756,1.9449470569099));
#12537=CARTESIAN_POINT('Ctrl Pts',(96.788834930743,-0.972573859713514,1.97922453140597));
#12538=CARTESIAN_POINT('Ctrl Pts',(96.7847628705008,-0.904245703895851,
2.0099641058949));
#12539=CARTESIAN_POINT('Ctrl Pts',(96.7816247197033,-0.851588315763736,
2.03365369162292));
#12540=CARTESIAN_POINT('Ctrl Pts',(96.7784865689059,-0.798065098219529,
2.05524304783608));
#12541=CARTESIAN_POINT('Ctrl Pts',(96.7753484181084,-0.743860152430341,
2.07467782405517));
#12542=CARTESIAN_POINT('Ctrl Pts',(96.7706169458065,-0.662133933335203,
2.103980146126));
#12543=CARTESIAN_POINT('Ctrl Pts',(96.7658854735045,-0.578598797540645,
2.12847663192413));
#12544=CARTESIAN_POINT('Ctrl Pts',(96.7611540012026,-0.493786047533441,
2.14797377527318));
#12545=CARTESIAN_POINT('Ctrl Pts',(96.7564655031284,-0.409743620629903,
2.16729383321967));
#12546=CARTESIAN_POINT('Ctrl Pts',(96.7517770050542,-0.324446834544995,
2.18170486705532));
#12547=CARTESIAN_POINT('Ctrl Pts',(96.7470885069799,-0.238433665781087,
2.19106489794853));
#12548=CARTESIAN_POINT('Ctrl Pts',(96.7428106204744,-0.159953400218962,
2.19960519149573));
#12549=CARTESIAN_POINT('Ctrl Pts',(96.7385327339688,-0.080877055221892,
2.2039408914976));
#12550=CARTESIAN_POINT('Ctrl Pts',(96.7342548474632,-0.00162714762936041,
2.20399939936258));
#12551=CARTESIAN_POINT('',(95.9842548473824,0.00150560105777076,2.20399948574528));
#12552=CARTESIAN_POINT('Ctrl Pts',(96.73425484741,-0.00162714664304999,
2.2039993993633));
#12553=CARTESIAN_POINT('Ctrl Pts',(96.7301906605558,0.0736638719990596,
2.20405498446386));
#12554=CARTESIAN_POINT('Ctrl Pts',(96.7261264737017,0.148992315837502,2.20024821452564));
#12555=CARTESIAN_POINT('Ctrl Pts',(96.7220622868475,0.223934505578098,2.19259420258549));
#12556=CARTESIAN_POINT('Ctrl Pts',(96.7179984623146,0.298870014240871,2.18494087299862));
#12557=CARTESIAN_POINT('Ctrl Pts',(96.7139346377817,0.373418864702078,2.1734410315032));
#12558=CARTESIAN_POINT('Ctrl Pts',(96.7098708132488,0.447162387060237,2.15816167133016));
#12559=CARTESIAN_POINT('Ctrl Pts',(96.7058060546237,0.520922859768338,2.14287879911303));
#12560=CARTESIAN_POINT('Ctrl Pts',(96.7017412959986,0.593877172113965,2.12381478140672));
#12561=CARTESIAN_POINT('Ctrl Pts',(96.6976765373735,0.665618288343953,2.10108740756354));
#12562=CARTESIAN_POINT('Ctrl Pts',(96.6936067811457,0.737447609957902,2.0783320905151));
#12563=CARTESIAN_POINT('Ctrl Pts',(96.689537024918,0.808060305621242,2.0519045738805));
#12564=CARTESIAN_POINT('Ctrl Pts',(96.6854672686902,0.877066608908877,2.02197185033251));
#12565=CARTESIAN_POINT('Ctrl Pts',(96.681394634172,0.946121716147331,1.99201795719423));
#12566=CARTESIAN_POINT('Ctrl Pts',(96.6773219996537,1.01356774536582,1.9585541355077));
#12567=CARTESIAN_POINT('Ctrl Pts',(96.6732493651355,1.07903933529307,1.92179346259953));
#12568=CARTESIAN_POINT('Ctrl Pts',(96.6691695124382,1.14462696452116,1.88496763650374));
#12569=CARTESIAN_POINT('Ctrl Pts',(96.6650896597409,1.20823277037885,1.84483355202713));
#12570=CARTESIAN_POINT('Ctrl Pts',(96.6610098070436,1.26952072280493,1.80164733906746));
#12571=CARTESIAN_POINT('Ctrl Pts',(96.6594057720588,1.29361669565812,1.78466824653922));
#12572=CARTESIAN_POINT('Ctrl Pts',(96.657801737074,1.31735475748164,1.76721780370166));
#12573=CARTESIAN_POINT('Ctrl Pts',(96.6561977020891,1.34071599508255,1.74931318537585));
#12574=CARTESIAN_POINT('Ctrl Pts',(96.6521246371532,1.40003629584514,1.70384867008471));
#12575=CARTESIAN_POINT('Ctrl Pts',(96.6480515722172,1.45715577536579,1.65527567673152));
#12576=CARTESIAN_POINT('Ctrl Pts',(96.6439785072812,1.51173041220667,1.6038351414062));
#12577=CARTESIAN_POINT('Ctrl Pts',(96.6399114264762,1.56622486820639,1.55247018231247));
#12578=CARTESIAN_POINT('Ctrl Pts',(96.6358443456711,1.61818156015399,1.49824637050675));
#12579=CARTESIAN_POINT('Ctrl Pts',(96.6317772648661,1.66728813025811,1.44144590280052));
#12580=CARTESIAN_POINT('Ctrl Pts',(96.6277149424972,1.71633724625903,1.38471189096622));
#12581=CARTESIAN_POINT('Ctrl Pts',(96.6236526201284,1.76254255482621,1.32540757204212));
#12582=CARTESIAN_POINT('Ctrl Pts',(96.6195902977596,1.80562848010989,1.26385196594223));
#12583=CARTESIAN_POINT('Ctrl Pts',(96.6155305536203,1.84868706009789,1.20233542726956));
#12584=CARTESIAN_POINT('Ctrl Pts',(96.611470809481,1.88862991235382,1.1385708269324));
#12585=CARTESIAN_POINT('Ctrl Pts',(96.6074110653417,1.9252225573414,1.07290917821773));
#12586=CARTESIAN_POINT('Ctrl Pts',(96.6033525858867,1.96180380305348,1.00726798430276));
#12587=CARTESIAN_POINT('Ctrl Pts',(96.5992941064317,1.99503668134416,0.93973133214225));
#12588=CARTESIAN_POINT('Ctrl Pts',(96.5952356269766,2.02473162271737,0.870676665570101));
#12589=CARTESIAN_POINT('Ctrl Pts',(96.5911771003443,2.0544269092761,0.801621196279736));
#12590=CARTESIAN_POINT('Ctrl Pts',(96.5871185737119,2.08058399028871,0.731048116874426));
#12591=CARTESIAN_POINT('Ctrl Pts',(96.5830600470795,2.10306124812793,0.659355281030354));
#12592=CARTESIAN_POINT('Ctrl Pts',(96.5789973700945,2.12556149178352,0.58758913026626));
#12593=CARTESIAN_POINT('Ctrl Pts',(96.5749346931094,2.14437425445206,0.514701392987236));
#12594=CARTESIAN_POINT('Ctrl Pts',(96.5708720161243,2.15940791454958,0.441104815866537));
#12595=CARTESIAN_POINT('Ctrl Pts',(96.5668072171473,2.17444942693409,0.367469798243549));
#12596=CARTESIAN_POINT('Ctrl Pts',(96.5627424181703,2.1857078344072,0.293125676005957));
#12597=CARTESIAN_POINT('Ctrl Pts',(96.5586776191932,2.19314318703594,0.218492473915826));
#12598=CARTESIAN_POINT('Ctrl Pts',(96.5546055589513,2.20059182201046,0.143725948761373));
#12599=CARTESIAN_POINT('Ctrl Pts',(96.5505334987093,2.20420373792287,0.0686697898906166));
#12600=CARTESIAN_POINT('Ctrl Pts',(96.5464614384673,2.20399112617167,-0.0062542590722837));
#12601=CARTESIAN_POINT('Ctrl Pts',(96.5433232876682,2.20382727600805,-0.0639948007512024));
#12602=CARTESIAN_POINT('Ctrl Pts',(96.5401851368692,2.20139308210989,-0.12165683177191));
#12603=CARTESIAN_POINT('Ctrl Pts',(96.5370469860701,2.19671505058251,-0.179050234694871));
#12604=CARTESIAN_POINT('Ctrl Pts',(96.5329739211341,2.19064334549127,-0.253542211649531));
#12605=CARTESIAN_POINT('Ctrl Pts',(96.5289008561981,2.18076653246242,-0.327868648322466));
#12606=CARTESIAN_POINT('Ctrl Pts',(96.5248277912621,2.16710071900694,-0.401609852567912));
#12607=CARTESIAN_POINT('Ctrl Pts',(96.520760710457,2.15345498331064,-0.475242716527136));
#12608=CARTESIAN_POINT('Ctrl Pts',(96.5166936296519,2.13603138580631,-0.548291589584893));
#12609=CARTESIAN_POINT('Ctrl Pts',(96.5126265488468,2.11489786941609,-0.620341036800958));
#12610=CARTESIAN_POINT('Ctrl Pts',(96.5085642264779,2.0937890789888,-0.692306187020324));
#12611=CARTESIAN_POINT('Ctrl Pts',(96.504501904109,2.06897912709108,-0.763273778706842));
#12612=CARTESIAN_POINT('Ctrl Pts',(96.5004395817402,2.04058683546056,-0.832839340416293));
#12613=CARTESIAN_POINT('Ctrl Pts',(96.4963798376008,2.0122125635338,-0.902360751029051));
#12614=CARTESIAN_POINT('Ctrl Pts',(96.4923200934615,1.9802606435506,-0.9704814564863));
#12615=CARTESIAN_POINT('Ctrl Pts',(96.4882603493221,1.94489905431959,-1.03681419189109));
#12616=CARTESIAN_POINT('Ctrl Pts',(96.4842018698671,1.9095484808678,-1.10312626344042));
#12617=CARTESIAN_POINT('Ctrl Pts',(96.480143390412,1.87079057153174,-1.16765104975184));
#12618=CARTESIAN_POINT('Ctrl Pts',(96.4760849109569,1.82883985302339,-1.23002471194418));
#12619=CARTESIAN_POINT('Ctrl Pts',(96.4720263843245,1.78688864686362,-1.29239909919216));
#12620=CARTESIAN_POINT('Ctrl Pts',(96.4679678576921,1.74174482579206,-1.35262191748397));
#12621=CARTESIAN_POINT('Ctrl Pts',(96.4639093310597,1.6936660521818,-1.41035857273494));
#12622=CARTESIAN_POINT('Ctrl Pts',(96.4598466540746,1.64553811199305,-1.46815427096014));
#12623=CARTESIAN_POINT('Ctrl Pts',(96.4557839770894,1.59446953193652,-1.5234583613693));
#12624=CARTESIAN_POINT('Ctrl Pts',(96.4517213001043,1.54075758074572,-1.57597020193105));
#12625=CARTESIAN_POINT('Ctrl Pts',(96.4476565011272,1.48701757506562,-1.62850947014785));
#12626=CARTESIAN_POINT('Ctrl Pts',(96.4435917021502,1.43063180716094,-1.67825326803271));
#12627=CARTESIAN_POINT('Ctrl Pts',(96.4395269031731,1.37193165971791,-1.72494043985978));
#12628=CARTESIAN_POINT('Ctrl Pts',(96.4354548429311,1.31312665165904,-1.77171101259474));
#12629=CARTESIAN_POINT('Ctrl Pts',(96.431382782689,1.25199939498887,-1.81541377467077));
#12630=CARTESIAN_POINT('Ctrl Pts',(96.427310722447,1.18891096833104,-1.85583046353436));
#12631=CARTESIAN_POINT('Ctrl Pts',(96.4241725716483,1.14029160006606,-1.88697775922724));
#12632=CARTESIAN_POINT('Ctrl Pts',(96.4210344208496,1.09050810071271,-1.9161743054736));
#12633=CARTESIAN_POINT('Ctrl Pts',(96.4178962700509,1.03973462442981,-1.94333937096993));
#12634=CARTESIAN_POINT('Ctrl Pts',(96.4138232051149,0.973834774743817,-1.97859742032909));
#12635=CARTESIAN_POINT('Ctrl Pts',(96.4097501401789,0.906012375112024,-2.01056760538032));
#12636=CARTESIAN_POINT('Ctrl Pts',(96.4056770752429,0.836628901732491,-2.0390360665731));
#12637=CARTESIAN_POINT('Ctrl Pts',(96.4016099944379,0.767347366278208,-2.06746270201505));
#12638=CARTESIAN_POINT('Ctrl Pts',(96.3975429136328,0.696509748712963,-2.09239764822724));
#12639=CARTESIAN_POINT('Ctrl Pts',(96.3934758328278,0.624502032568093,-2.11367291966338));
#12640=CARTESIAN_POINT('Ctrl Pts',(96.3894135104589,0.552578564595041,-2.13492329928487));
#12641=CARTESIAN_POINT('Ctrl Pts',(96.3853511880901,0.479488173527562,-2.15252237643355));
#12642=CARTESIAN_POINT('Ctrl Pts',(96.3812888657212,0.405635195328789,-2.16635086916007));
#12643=CARTESIAN_POINT('Ctrl Pts',(96.3772291215819,0.331829089316586,-2.18017058537267));
#12644=CARTESIAN_POINT('Ctrl Pts',(96.3731693774426,0.257261824714813,-2.19022437830546));
#12645=CARTESIAN_POINT('Ctrl Pts',(96.3691096333033,0.182349909793452,-2.1964436051031));
#12646=CARTESIAN_POINT('Ctrl Pts',(96.3650511538482,0.107461331298148,-2.20266089449831));
#12647=CARTESIAN_POINT('Ctrl Pts',(96.3609926743932,0.0322287911648629,
-2.2050459499835));
#12648=CARTESIAN_POINT('Ctrl Pts',(96.3569341949382,-0.0429256711574192,
-2.20358194464279));
#12649=CARTESIAN_POINT('Ctrl Pts',(96.3528756683058,-0.118081007104319,
-2.20211792228391));
#12650=CARTESIAN_POINT('Ctrl Pts',(96.3488171416734,-0.193157786102896,
-2.19680476135209));
#12651=CARTESIAN_POINT('Ctrl Pts',(96.344758615041,-0.267735176999542,-2.1876777356359));
#12652=CARTESIAN_POINT('Ctrl Pts',(96.3406959380559,-0.342388832635664,
-2.17854137639075));
#12653=CARTESIAN_POINT('Ctrl Pts',(96.3366332610708,-0.416541605379462,
-2.16558342210309));
#12654=CARTESIAN_POINT('Ctrl Pts',(96.3325705840857,-0.489779741042405,
-2.14889083139755));
#12655=CARTESIAN_POINT('Ctrl Pts',(96.3285057851087,-0.563056129988674,
-2.13218952192279));
#12656=CARTESIAN_POINT('Ctrl Pts',(96.3244409861316,-0.635416470597316,
-2.11174982140798));
#12657=CARTESIAN_POINT('Ctrl Pts',(96.3203761871546,-0.706461713050952,
-2.08770875554832));
#12658=CARTESIAN_POINT('Ctrl Pts',(96.3163041269126,-0.777633869119079,
-2.06362474327228));
#12659=CARTESIAN_POINT('Ctrl Pts',(96.3122320666706,-0.847485790065002,
-2.03592669169464));
#12660=CARTESIAN_POINT('Ctrl Pts',(96.3081600064286,-0.915638387665817,
-2.00479982617536));
#12661=CARTESIAN_POINT('Ctrl Pts',(96.3050218556296,-0.96816048112697,-1.98081177293148));
#12662=CARTESIAN_POINT('Ctrl Pts',(96.3018837048307,-1.01967373109716,-1.95478831815319));
#12663=CARTESIAN_POINT('Ctrl Pts',(96.2987455540318,-1.07001592308488,-1.92683209552488));
#12664=CARTESIAN_POINT('Ctrl Pts',(96.2946724890958,-1.13535600076876,-1.89054718844879));
#12665=CARTESIAN_POINT('Ctrl Pts',(96.2905994241598,-1.19897432457061,-1.85086495690024));
#12666=CARTESIAN_POINT('Ctrl Pts',(96.2865263592238,-1.26049529155207,-1.80797334603558));
#12667=CARTESIAN_POINT('Ctrl Pts',(96.2824592784188,-1.32192587217154,-1.76514475135638));
#12668=CARTESIAN_POINT('Ctrl Pts',(96.2783921976137,-1.38126482544665,-1.7191164097707));
#12669=CARTESIAN_POINT('Ctrl Pts',(96.2743251168087,-1.43816182669763,-1.67012172018381));
#12670=CARTESIAN_POINT('Ctrl Pts',(96.2702627944398,-1.49499225913369,-1.62118435380116));
#12671=CARTESIAN_POINT('Ctrl Pts',(96.2662004720709,-1.54938605587491,-1.56928784467997));
#12672=CARTESIAN_POINT('Ctrl Pts',(96.2621381497021,-1.60102388360845,-1.51470740544678));
#12673=CARTESIAN_POINT('Ctrl Pts',(96.2580784055628,-1.65262893841995,-1.46016160671956));
#12674=CARTESIAN_POINT('Ctrl Pts',(96.2540186614234,-1.70148116787368,-1.40293560406399));
#12675=CARTESIAN_POINT('Ctrl Pts',(96.2499589172841,-1.74729720531625,-1.34334227816071));
#12676=CARTESIAN_POINT('Ctrl Pts',(96.2459004378291,-1.79309897022865,-1.28376751666392));
#12677=CARTESIAN_POINT('Ctrl Pts',(96.241841958374,-1.83586613020979,-1.22182727439976));
#12678=CARTESIAN_POINT('Ctrl Pts',(96.237783478919,-1.87535587269699,-1.15786715591251));
#12679=CARTESIAN_POINT('Ctrl Pts',(96.2337249522866,-1.91484607422822,-1.09390629392811));
#12680=CARTESIAN_POINT('Ctrl Pts',(96.2296664256542,-1.95105853331316,-1.02792591630782));
#12681=CARTESIAN_POINT('Ctrl Pts',(96.2256078990218,-1.98379488240875,-0.960298841261847));
#12682=CARTESIAN_POINT('Ctrl Pts',(96.2215452220367,-2.01656470852874,-0.892602609046438));
#12683=CARTESIAN_POINT('Ctrl Pts',(96.2174825450516,-2.04585111751407,-0.823256747355467));
#12684=CARTESIAN_POINT('Ctrl Pts',(96.2134198680665,-2.07150301707198,-0.752656130156174));
#12685=CARTESIAN_POINT('Ctrl Pts',(96.2093550690895,-2.09716831496909,-0.682018637285601));
#12686=CARTESIAN_POINT('Ctrl Pts',(96.2052902701124,-2.1191951830527,-0.610125540728479));
#12687=CARTESIAN_POINT('Ctrl Pts',(96.2012254711354,-2.13748257724314,-0.537386482879899));
#12688=CARTESIAN_POINT('Ctrl Pts',(96.1971534108933,-2.155802639621,-0.464517485623342));
#12689=CARTESIAN_POINT('Ctrl Pts',(96.1930813506513,-2.17036979240415,-0.390799977656557));
#12690=CARTESIAN_POINT('Ctrl Pts',(96.1890092904093,-2.18113431865364,-0.316652939337917));
#12691=CARTESIAN_POINT('Ctrl Pts',(96.1858711396104,-2.18943004726324,-0.259511204268338));
#12692=CARTESIAN_POINT('Ctrl Pts',(96.1827329888115,-2.19546842055734,-0.202114573975238));
#12693=CARTESIAN_POINT('Ctrl Pts',(96.1795948380126,-2.19924781041177,-0.144654997836399));
#12694=CARTESIAN_POINT('Ctrl Pts',(96.1755217730766,-2.20415315157665,-0.0700771334172606));
#12695=CARTESIAN_POINT('Ctrl Pts',(96.1714487081406,-2.20527017959899,0.00489434697652635));
#12696=CARTESIAN_POINT('Ctrl Pts',(96.1673756432046,-2.20255335191165,0.0798419187065264));
#12697=CARTESIAN_POINT('Ctrl Pts',(96.1633085623996,-2.19984051577682,0.154679377760128));
#12698=CARTESIAN_POINT('Ctrl Pts',(96.1592414815945,-2.19330502426454,0.229492524704092));
#12699=CARTESIAN_POINT('Ctrl Pts',(96.1551744007894,-2.18295323469984,0.303860453355697));
#12700=CARTESIAN_POINT('Ctrl Pts',(96.1511120784206,-2.17261355660587,0.378141372414798));
#12701=CARTESIAN_POINT('Ctrl Pts',(96.1470497560517,-2.15846651693741,0.4519776375663));
#12702=CARTESIAN_POINT('Ctrl Pts',(96.1429874336828,-2.14057040896888,0.52495173515933));
#12703=CARTESIAN_POINT('Ctrl Pts',(96.1389276895435,-2.12268565910306,0.59787951836394));
#12704=CARTESIAN_POINT('Ctrl Pts',(96.1348679454042,-2.10105667606701,0.66994575730682));
#12705=CARTESIAN_POINT('Ctrl Pts',(96.1308082012649,-2.07579290039091,0.740742758781129));
#12706=CARTESIAN_POINT('Ctrl Pts',(96.1267497218099,-2.05053699484118,0.811517705699732));
#12707=CARTESIAN_POINT('Ctrl Pts',(96.1226912423548,-2.02164870515795,0.881023750787546));
#12708=CARTESIAN_POINT('Ctrl Pts',(96.1186327628998,-1.98928694912814,0.948869555855008));
#12709=CARTESIAN_POINT('Ctrl Pts',(96.1145742362674,-1.95692481691258,1.01671614958869));
#12710=CARTESIAN_POINT('Ctrl Pts',(96.110515709635,-1.92108934535601,1.08290203480788));
#12711=CARTESIAN_POINT('Ctrl Pts',(96.1064571830025,-1.88198640639796,1.14705848418174));
#12712=CARTESIAN_POINT('Ctrl Pts',(96.1023945060174,-1.84284347977863,1.2112805415747));
#12713=CARTESIAN_POINT('Ctrl Pts',(96.0983318290323,-1.80042666222557,1.27346861015385));
#12714=CARTESIAN_POINT('Ctrl Pts',(96.0942691520472,-1.75498597811549,1.33328174690049));
#12715=CARTESIAN_POINT('Ctrl Pts',(96.0902043530702,-1.70952155971248,1.39312612486932));
#12716=CARTESIAN_POINT('Ctrl Pts',(96.0861395540932,-1.66103043771791,1.45059273550423));
#12717=CARTESIAN_POINT('Ctrl Pts',(96.0820747551161,-1.60980216643582,1.50537469918241));
#12718=CARTESIAN_POINT('Ctrl Pts',(96.0780026948741,-1.55848238212846,1.5602545241216));
#12719=CARTESIAN_POINT('Ctrl Pts',(96.0739306346321,-1.50441602602296,1.61243979080215));
#12720=CARTESIAN_POINT('Ctrl Pts',(96.0698585743901,-1.44792831102597,1.66166170026558));
#12721=CARTESIAN_POINT('Ctrl Pts',(96.0667204235912,-1.4043958096856,1.69959477721525));
#12722=CARTESIAN_POINT('Ctrl Pts',(96.0635822727924,-1.35942598893592,1.73576866756006));
#12723=CARTESIAN_POINT('Ctrl Pts',(96.0604441219935,-1.31317929896625,1.77007800075774));
#12724=CARTESIAN_POINT('Ctrl Pts',(96.0563512646815,-1.25286317162506,1.81482511912447));
#12725=CARTESIAN_POINT('Ctrl Pts',(96.0522584073694,-1.1901404740041,1.85657251872614));
#12726=CARTESIAN_POINT('Ctrl Pts',(96.0481655500574,-1.1253399084655,1.89505305741419));
#12727=CARTESIAN_POINT('Ctrl Pts',(96.044078778494,-1.06063569613981,1.93347637864577));
#12728=CARTESIAN_POINT('Ctrl Pts',(96.0399920069305,-0.993860150335465,
1.96864224341765));
#12729=CARTESIAN_POINT('Ctrl Pts',(96.0359052353671,-0.925373102248549,
2.00032512898151));
#12730=CARTESIAN_POINT('Ctrl Pts',(96.0318232633005,-0.856966485220754,
2.03197080622477));
#12731=CARTESIAN_POINT('Ctrl Pts',(96.0277412912338,-0.78685278257689,2.06014143048253));
#12732=CARTESIAN_POINT('Ctrl Pts',(96.0236593191671,-0.715417411484009,
2.0846567888613));
#12733=CARTESIAN_POINT('Ctrl Pts',(96.0195809795603,-0.644045609203774,
2.10915033154569));
#12734=CARTESIAN_POINT('Ctrl Pts',(96.0155026399535,-0.571354920030052,
2.12999492007944));
#12735=CARTESIAN_POINT('Ctrl Pts',(96.0114243003467,-0.497750332949793,
2.14705859399514));
#12736=CARTESIAN_POINT('Ctrl Pts',(96.0073480219645,-0.424182946201418,
2.16411364379707));
#12737=CARTESIAN_POINT('Ctrl Pts',(96.0032717435823,-0.349703037890821,
2.17739147084455));
#12738=CARTESIAN_POINT('Ctrl Pts',(95.9991954652001,-0.274728945169834,
2.18681046428031));
#12739=CARTESIAN_POINT('Ctrl Pts',(95.9951194772191,-0.19976019373505,2.19622878669041));
#12740=CARTESIAN_POINT('Ctrl Pts',(95.9910434892382,-0.124297794801206,
2.20178876026211));
#12741=CARTESIAN_POINT('Ctrl Pts',(95.9869675012572,-0.048767058015047,
2.20346040900502));
#12742=CARTESIAN_POINT('Ctrl Pts',(95.9860632833082,-0.0320113049980311,
2.20383124788015));
#12743=CARTESIAN_POINT('Ctrl Pts',(95.9851590653591,-0.0152522006656639,
2.20401093336839));
#12744=CARTESIAN_POINT('Ctrl Pts',(95.98425484741,0.00150560054724205,2.20399948574563));
#12745=CARTESIAN_POINT('',(95.2342548474574,0.000867116891644239,2.20399982942565));
#12746=CARTESIAN_POINT('Ctrl Pts',(95.9842548473825,0.00150560105777081,
2.20399948574528));
#12747=CARTESIAN_POINT('Ctrl Pts',(95.9796357852113,0.0871103225000559,
2.20394100725652));
#12748=CARTESIAN_POINT('Ctrl Pts',(95.9750167230401,0.172519533150872,2.19889107907991));
#12749=CARTESIAN_POINT('Ctrl Pts',(95.9703976608689,0.257195271049002,2.18894188880154));
#12750=CARTESIAN_POINT('Ctrl Pts',(95.9655469517198,0.346117515718511,2.17849374445514));
#12751=CARTESIAN_POINT('Ctrl Pts',(95.9606962425707,0.434230493468681,2.16264236725634));
#12752=CARTESIAN_POINT('Ctrl Pts',(95.9558455334216,0.520933001701834,2.14155196241836));
#12753=CARTESIAN_POINT('Ctrl Pts',(95.9509948242725,0.607635509934981,2.12046155758038));
#12754=CARTESIAN_POINT('Ctrl Pts',(95.9461441151234,0.692927346047603,2.09413232587469));
#12755=CARTESIAN_POINT('Ctrl Pts',(95.9412934059743,0.776232806747002,2.06278419368815));
#12756=CARTESIAN_POINT('Ctrl Pts',(95.9372203410383,0.846183104841956,2.03646165525239));
#12757=CARTESIAN_POINT('Ctrl Pts',(95.9331472761023,0.914927859152941,2.00652623511549));
#12758=CARTESIAN_POINT('Ctrl Pts',(95.9290742111664,0.982067987979568,1.97310883303121));
#12759=CARTESIAN_POINT('Ctrl Pts',(95.9250071303613,1.04910947479376,1.93974052766225));
#12760=CARTESIAN_POINT('Ctrl Pts',(95.9209400495562,1.11455059284824,1.90290060810877));
#12761=CARTESIAN_POINT('Ctrl Pts',(95.9168729687512,1.17801060799517,1.86276864034449));
#12762=CARTESIAN_POINT('Ctrl Pts',(95.9128106463823,1.2413963756789,1.82268362650533));
#12763=CARTESIAN_POINT('Ctrl Pts',(95.9087483240135,1.30280524401684,1.77931447073365));
#12764=CARTESIAN_POINT('Ctrl Pts',(95.9046860016446,1.36188101108845,1.73288664131175));
#12765=CARTESIAN_POINT('Ctrl Pts',(95.9006262575053,1.42091928460951,1.68648827818806));
#12766=CARTESIAN_POINT('Ctrl Pts',(95.896566513366,1.47762702079588,1.63703538788661));
#12767=CARTESIAN_POINT('Ctrl Pts',(95.8925067692267,1.53167807883756,1.58479596882643));
#12768=CARTESIAN_POINT('Ctrl Pts',(95.8884482897716,1.58571229899001,1.53257282329692));
#12769=CARTESIAN_POINT('Ctrl Pts',(95.8843898103166,1.63709114107314,1.47756520409031));
#12770=CARTESIAN_POINT('Ctrl Pts',(95.8803313308615,1.68552378756024,1.42007942086652));
#12771=CARTESIAN_POINT('Ctrl Pts',(95.8762728042292,1.73395699704716,1.36259296940574));
#12772=CARTESIAN_POINT('Ctrl Pts',(95.8722142775968,1.77944363667206,1.30262866302669));
#12773=CARTESIAN_POINT('Ctrl Pts',(95.8681557509644,1.82173286828323,1.24052624180892));
#12774=CARTESIAN_POINT('Ctrl Pts',(95.8640930739793,1.86406534593982,1.17836031307337));
#12775=CARTESIAN_POINT('Ctrl Pts',(95.8600303969942,1.90319361674,1.11405229872748));
#12776=CARTESIAN_POINT('Ctrl Pts',(95.8559677200091,1.93891037713846,1.04797068156739));
#12777=CARTESIAN_POINT('Ctrl Pts',(95.8519029210321,1.97464579289105,0.98185454907175));
#12778=CARTESIAN_POINT('Ctrl Pts',(95.847838122055,2.00696594438313,0.913963400475804));
#12779=CARTESIAN_POINT('Ctrl Pts',(95.843773323078,2.03571087317361,0.844687658748921));
#12780=CARTESIAN_POINT('Ctrl Pts',(95.839701262836,2.06450715125482,0.77528816440368));
#12781=CARTESIAN_POINT('Ctrl Pts',(95.835629202594,2.08971528929234,0.704499586951367));
#12782=CARTESIAN_POINT('Ctrl Pts',(95.831557142352,2.11122473453427,0.632729104981504));
#12783=CARTESIAN_POINT('Ctrl Pts',(95.8284189915531,2.12780108133615,0.577418873318676));
#12784=CARTESIAN_POINT('Ctrl Pts',(95.8252808407542,2.14218175830437,0.521525839307777));
#12785=CARTESIAN_POINT('Ctrl Pts',(95.8221426899553,2.1543370382082,0.465239643414357));
#12786=CARTESIAN_POINT('Ctrl Pts',(95.8180696250193,2.17011360458,0.392184731281153));
#12787=CARTESIAN_POINT('Ctrl Pts',(95.8139965600833,2.18220037643508,0.318185538243844));
#12788=CARTESIAN_POINT('Ctrl Pts',(95.8099234951473,2.19049114360055,0.243648414334174));
#12789=CARTESIAN_POINT('Ctrl Pts',(95.8058564143422,2.19876973000362,0.169220800072788));
#12790=CARTESIAN_POINT('Ctrl Pts',(95.8017893335372,2.20326333214251,0.0942572946533874));
#12791=CARTESIAN_POINT('Ctrl Pts',(95.7977222527321,2.203916584601,0.0191751954530534));
#12792=CARTESIAN_POINT('Ctrl Pts',(95.7936599303632,2.20456907276188,-0.0558190585838011));
#12793=CARTESIAN_POINT('Ctrl Pts',(95.7895976079943,2.20139013399951,-0.130931155687019));
#12794=CARTESIAN_POINT('Ctrl Pts',(95.7855352856255,2.19437627558659,-0.205739546861371));
#12795=CARTESIAN_POINT('Ctrl Pts',(95.7814755414861,2.18736686865129,-0.280500459478317));
#12796=CARTESIAN_POINT('Ctrl Pts',(95.7774157973468,2.17652741634232,-0.354957574492192));
#12797=CARTESIAN_POINT('Ctrl Pts',(95.7733560532075,2.16190645999275,-0.428691565395923));
#12798=CARTESIAN_POINT('Ctrl Pts',(95.7692975737525,2.14729005833742,-0.502402586818363));
#12799=CARTESIAN_POINT('Ctrl Pts',(95.7652390942974,2.12889458433321,-0.575390463351062));
#12800=CARTESIAN_POINT('Ctrl Pts',(95.7611806148423,2.10681991856933,-0.647244799685204));
#12801=CARTESIAN_POINT('Ctrl Pts',(95.7571220882099,2.08474499620098,-0.71909997128198));
#12802=CARTESIAN_POINT('Ctrl Pts',(95.7530635615775,2.05899093908381,-0.789821120635661));
#12803=CARTESIAN_POINT('Ctrl Pts',(95.7490050349451,2.0297073875272,-0.859013341582951));
#12804=CARTESIAN_POINT('Ctrl Pts',(95.74494235796,2.0003938898649,-0.928276320257746));
#12805=CARTESIAN_POINT('Ctrl Pts',(95.7408796809749,1.9675438766001,-0.996006807583816));
#12806=CARTESIAN_POINT('Ctrl Pts',(95.7368170039898,1.93135473407245,-1.06183091458854));
#12807=CARTESIAN_POINT('Ctrl Pts',(95.7327522050128,1.89514668945899,-1.12768940242773));
#12808=CARTESIAN_POINT('Ctrl Pts',(95.7286874060357,1.85559629380616,-1.19163912059643));
#12809=CARTESIAN_POINT('Ctrl Pts',(95.7246226070587,1.81294502659153,-1.25333408577164));
#12810=CARTESIAN_POINT('Ctrl Pts',(95.7205505468166,1.77021756811771,-1.3151392614374));
#12811=CARTESIAN_POINT('Ctrl Pts',(95.7164784865746,1.72437846540206,-1.37468125991971));
#12812=CARTESIAN_POINT('Ctrl Pts',(95.7124064263326,1.6757100499405,-1.43164654455225));
#12813=CARTESIAN_POINT('Ctrl Pts',(95.7092682755337,1.63820352553184,-1.47554708699346));
#12814=CARTESIAN_POINT('Ctrl Pts',(95.7061301247349,1.59901750013507,-1.51791795593156));
#12815=CARTESIAN_POINT('Ctrl Pts',(95.702991973936,1.55829525863933,-1.558631414704));
#12816=CARTESIAN_POINT('Ctrl Pts',(95.698918909,1.50544109560459,-1.611474178477));
#12817=CARTESIAN_POINT('Ctrl Pts',(95.694845844064,1.44979406352332,-1.66172732210596));
#12818=CARTESIAN_POINT('Ctrl Pts',(95.690772779128,1.3916381503919,-1.7090814077667));
#12819=CARTESIAN_POINT('Ctrl Pts',(95.686705698323,1.33356767969855,-1.75636592099167));
#12820=CARTESIAN_POINT('Ctrl Pts',(95.6826386175179,1.27299601341587,-1.80075953369305));
#12821=CARTESIAN_POINT('Ctrl Pts',(95.6785715367128,1.21024388945352,-1.84198961127375));
#12822=CARTESIAN_POINT('Ctrl Pts',(95.674509214344,1.14756518473018,-1.88317145015384));
#12823=CARTESIAN_POINT('Ctrl Pts',(95.6704468919751,1.08271148783142,-1.92119684668641));
#12824=CARTESIAN_POINT('Ctrl Pts',(95.6663845696062,1.01603521581505,-1.95583446135497));
#12825=CARTESIAN_POINT('Ctrl Pts',(95.6623248254669,0.949401261153161,-1.99045009260762));
#12826=CARTESIAN_POINT('Ctrl Pts',(95.6582650813276,0.88094744940858,-2.0216819891268));
#12827=CARTESIAN_POINT('Ctrl Pts',(95.6542053371883,0.811052522772792,-2.04934374991213));
#12828=CARTESIAN_POINT('Ctrl Pts',(95.6501468577333,0.741179369679854,-2.07699689355508));
#12829=CARTESIAN_POINT('Ctrl Pts',(95.6460883782783,0.669866436701337,-2.1010819340282));
#12830=CARTESIAN_POINT('Ctrl Pts',(95.6420298988232,0.597512776071211,-2.12146045978512));
#12831=CARTESIAN_POINT('Ctrl Pts',(95.6379713721908,0.525158274374103,-2.14183922242992));
#12832=CARTESIAN_POINT('Ctrl Pts',(95.6339128455584,0.451763481070672,-2.15851125709418));
#12833=CARTESIAN_POINT('Ctrl Pts',(95.6298543189261,0.377741390695677,-2.17138836732522));
#12834=CARTESIAN_POINT('Ctrl Pts',(95.625791641941,0.303643603445691,-2.18427864601717));
#12835=CARTESIAN_POINT('Ctrl Pts',(95.6217289649559,0.228917709546249,-2.1933661685537));
#12836=CARTESIAN_POINT('Ctrl Pts',(95.6176662879708,0.153984908484414,-2.19861425628941));
#12837=CARTESIAN_POINT('Ctrl Pts',(95.6136014889937,0.0790129689921754,
-2.20386508517337));
#12838=CARTESIAN_POINT('Ctrl Pts',(95.6095366900167,0.003834384947001,-2.20527247677358));
#12839=CARTESIAN_POINT('Ctrl Pts',(95.6054718910397,-0.071129208133638,
-2.20285193232552));
#12840=CARTESIAN_POINT('Ctrl Pts',(95.6013998307977,-0.146226714481638,
-2.20042706387161));
#12841=CARTESIAN_POINT('Ctrl Pts',(95.5973277705557,-0.221107986241424,
-2.19416064059518));
#12842=CARTESIAN_POINT('Ctrl Pts',(95.5932557103136,-0.295356524660395,
-2.18412007988126));
#12843=CARTESIAN_POINT('Ctrl Pts',(95.5901175595148,-0.352576481219793,
-2.17638227843606));
#12844=CARTESIAN_POINT('Ctrl Pts',(95.5869794087159,-0.409420744171687,
-2.16640405763089));
#12845=CARTESIAN_POINT('Ctrl Pts',(95.583841257917,-0.465704316896587,-2.15423663723925));
#12846=CARTESIAN_POINT('Ctrl Pts',(95.579768192981,-0.538755824370337,-2.13844431349996));
#12847=CARTESIAN_POINT('Ctrl Pts',(95.575695128045,-0.611144004893231,-2.11890149014625));
#12848=CARTESIAN_POINT('Ctrl Pts',(95.571622063109,-0.682454907239795,-2.09567919767896));
#12849=CARTESIAN_POINT('Ctrl Pts',(95.567554982304,-0.753661039890029,-2.07249102331213));
#12850=CARTESIAN_POINT('Ctrl Pts',(95.5634879014989,-0.823792586508467,
-2.04563425928801));
#12851=CARTESIAN_POINT('Ctrl Pts',(95.5594208206938,-0.892446616911418,
-2.01523076494067));
#12852=CARTESIAN_POINT('Ctrl Pts',(95.555358498325,-0.96102032291499,-1.98486284232027));
#12853=CARTESIAN_POINT('Ctrl Pts',(95.5512961759561,-1.02811951281543,-1.95095662611143));
#12854=CARTESIAN_POINT('Ctrl Pts',(95.5472338535872,-1.09335880029237,-1.91368297631118));
#12855=CARTESIAN_POINT('Ctrl Pts',(95.5431741094479,-1.15855668242417,-1.8764329829363));
#12856=CARTESIAN_POINT('Ctrl Pts',(95.5391143653086,-1.22189659103513,-1.83582003328102));
#12857=CARTESIAN_POINT('Ctrl Pts',(95.5350546211693,-1.28301664686955,-1.79206146207534));
#12858=CARTESIAN_POINT('Ctrl Pts',(95.5309961417142,-1.34411766269323,-1.7483165224617));
#12859=CARTESIAN_POINT('Ctrl Pts',(95.5269376622592,-1.4029998107652,-1.70142818464707));
#12860=CARTESIAN_POINT('Ctrl Pts',(95.5228791828041,-1.45933054229003,-1.65165685550586));
#12861=CARTESIAN_POINT('Ctrl Pts',(95.5188206561717,-1.51566192862509,-1.60188494780344));
#12862=CARTESIAN_POINT('Ctrl Pts',(95.5147621295393,-1.56944148290727,-1.54923029971699));
#12863=CARTESIAN_POINT('Ctrl Pts',(95.5107036029069,-1.62037130761176,-1.49399224411259));
#12864=CARTESIAN_POINT('Ctrl Pts',(95.5066409259218,-1.6713532144522,-1.43869770066557));
#12865=CARTESIAN_POINT('Ctrl Pts',(95.5025782489367,-1.71947924784372,-1.3808148258672));
#12866=CARTESIAN_POINT('Ctrl Pts',(95.4985155719516,-1.76449036506856,-1.32067776220403));
#12867=CARTESIAN_POINT('Ctrl Pts',(95.4944507729746,-1.80952499221767,-1.26050928812716));
#12868=CARTESIAN_POINT('Ctrl Pts',(95.4903859739975,-1.85144119684918,-1.1980846772798));
#12869=CARTESIAN_POINT('Ctrl Pts',(95.4863211750204,-1.89002355688284,-1.13376671076018));
#12870=CARTESIAN_POINT('Ctrl Pts',(95.4822491147784,-1.92867483957191,-1.06933384807972));
#12871=CARTESIAN_POINT('Ctrl Pts',(95.4781770545364,-1.96398015734139,-1.00300129605404));
#12872=CARTESIAN_POINT('Ctrl Pts',(95.4741049942944,-1.99577050653869,-0.935155647595793));
#12873=CARTESIAN_POINT('Ctrl Pts',(95.4709668434955,-2.02026987634191,-0.882870105816989));
#12874=CARTESIAN_POINT('Ctrl Pts',(95.4678286926966,-2.04268262813904,-0.82968642713777));
#12875=CARTESIAN_POINT('Ctrl Pts',(95.4646905418978,-2.06295157688694,-0.7757878520702));
#12876=CARTESIAN_POINT('Ctrl Pts',(95.4606174769618,-2.08925902663219,-0.705831877906623));
#12877=CARTESIAN_POINT('Ctrl Pts',(95.4565444120258,-2.11205479901269,-0.634401328520342));
#12878=CARTESIAN_POINT('Ctrl Pts',(95.4524713470898,-2.13117430748127,-0.561882613302562));
#12879=CARTESIAN_POINT('Ctrl Pts',(95.4484042662847,-2.15026572564346,-0.489470442295007));
#12880=CARTESIAN_POINT('Ctrl Pts',(95.4443371854797,-2.1656914826729,-0.415973737436818));
#12881=CARTESIAN_POINT('Ctrl Pts',(95.4402701046746,-2.17733568478907,-0.341797185102692));
#12882=CARTESIAN_POINT('Ctrl Pts',(95.4362077823057,-2.18896626332719,-0.267707418452967));
#12883=CARTESIAN_POINT('Ctrl Pts',(95.4321454599369,-2.19682400350121,-0.192939853946335));
#12884=CARTESIAN_POINT('Ctrl Pts',(95.428083137568,-2.20084370192936,-0.117910982007089));
#12885=CARTESIAN_POINT('Ctrl Pts',(95.4240233934287,-2.20486084918003,-0.0429297285575062));
#12886=CARTESIAN_POINT('Ctrl Pts',(95.4199636492894,-2.20504476295785,0.032312027657186));
#12887=CARTESIAN_POINT('Ctrl Pts',(95.4159039051501,-2.20138203823516,0.107392372800067));
#12888=CARTESIAN_POINT('Ctrl Pts',(95.411845425695,-2.19772045451793,0.182449329047782));
#12889=CARTESIAN_POINT('Ctrl Pts',(95.40778694624,-2.19021463471915,0.257344497474993));
#12890=CARTESIAN_POINT('Ctrl Pts',(95.4037284667849,-2.17890326754456,0.331657278954689));
#12891=CARTESIAN_POINT('Ctrl Pts',(95.3996699401525,-2.16759176888227,0.405970924274905));
#12892=CARTESIAN_POINT('Ctrl Pts',(95.3956114135202,-2.15247470863038,0.479701697451623));
#12893=CARTESIAN_POINT('Ctrl Pts',(95.3915528868878,-2.13364226733496,0.552437032648741));
#12894=CARTESIAN_POINT('Ctrl Pts',(95.3874902099027,-2.11479056750539,0.625246748852262));
#12895=CARTESIAN_POINT('Ctrl Pts',(95.3834275329176,-2.09221601930329,0.697058531022004));
#12896=CARTESIAN_POINT('Ctrl Pts',(95.3793648559325,-2.06605911289123,0.767473609995231));
#12897=CARTESIAN_POINT('Ctrl Pts',(95.3753000569555,-2.03988854436796,0.837925467730612));
#12898=CARTESIAN_POINT('Ctrl Pts',(95.3712352579784,-2.01013208061837,0.906978730617126));
#12899=CARTESIAN_POINT('Ctrl Pts',(95.3671704590014,-1.97697791694915,0.974255775397501));
#12900=CARTESIAN_POINT('Ctrl Pts',(95.3630983987593,-1.94376452743175,1.04165300236919));
#12901=CARTESIAN_POINT('Ctrl Pts',(95.3590263385173,-1.90714154754015,1.10726725588856));
#12902=CARTESIAN_POINT('Ctrl Pts',(95.3549542782753,-1.8673423367302,1.17074702538806));
#12903=CARTESIAN_POINT('Ctrl Pts',(95.3518161274765,-1.83667090316217,1.21966798370595));
#12904=CARTESIAN_POINT('Ctrl Pts',(95.3486779766776,-1.8041140182598,1.26732178068403));
#12905=CARTESIAN_POINT('Ctrl Pts',(95.3455398258787,-1.76979471058198,1.31356106915363));
#12906=CARTESIAN_POINT('Ctrl Pts',(95.3415053544189,-1.72567310004701,1.37300725310416));
#12907=CARTESIAN_POINT('Ctrl Pts',(95.337470882959,-1.67845985876083,1.43035320436202));
#12908=CARTESIAN_POINT('Ctrl Pts',(95.3334364114992,-1.62838390961034,1.48525480740584));
#12909=CARTESIAN_POINT('Ctrl Pts',(95.3293038463307,-1.57709041917589,1.54149128216742));
#12910=CARTESIAN_POINT('Ctrl Pts',(95.3251712811623,-1.52279341517083,1.59516252052928));
#12911=CARTESIAN_POINT('Ctrl Pts',(95.3210387159939,-1.4657859356181,1.64593061547082));
#12912=CARTESIAN_POINT('Ctrl Pts',(95.3170149216926,-1.41027891709368,1.69536247263202));
#12913=CARTESIAN_POINT('Ctrl Pts',(95.3129911273913,-1.35220273106132,1.74204177364241));
#12914=CARTESIAN_POINT('Ctrl Pts',(95.30896733309,-1.29186683262772,1.78569204701047));
#12915=CARTESIAN_POINT('Ctrl Pts',(95.3049459527131,-1.23156713045278,1.82931613403462));
#12916=CARTESIAN_POINT('Ctrl Pts',(95.3009245723363,-1.16901079881204,1.86991451268246));
#12917=CARTESIAN_POINT('Ctrl Pts',(95.2969031919594,-1.10453991000684,1.90725131726316));
#12918=CARTESIAN_POINT('Ctrl Pts',(95.292882863597,-1.04008588712866,1.94457835433744));
#12919=CARTESIAN_POINT('Ctrl Pts',(95.2888625352346,-0.973718723115101,
1.97864526717714));
#12920=CARTESIAN_POINT('Ctrl Pts',(95.2848422068722,-0.905807482380869,
2.00926076079309));
#12921=CARTESIAN_POINT('Ctrl Pts',(95.2806265935876,-0.834597495831594,
2.04136338275995));
#12922=CARTESIAN_POINT('Ctrl Pts',(95.2764109803031,-0.761690125013591,
2.06967047871341));
#12923=CARTESIAN_POINT('Ctrl Pts',(95.2721953670185,-0.687535305187299,
2.09401795697196));
#12924=CARTESIAN_POINT('Ctrl Pts',(95.268170641133,-0.616738293520773,2.11726295583189));
#12925=CARTESIAN_POINT('Ctrl Pts',(95.2641459152475,-0.5448048662267,2.13689908807007));
#12926=CARTESIAN_POINT('Ctrl Pts',(95.260121189362,-0.472140595541541,2.15283516741103));
#12927=CARTESIAN_POINT('Ctrl Pts',(95.2560939465934,-0.399430883880333,
2.16878121246132));
#12928=CARTESIAN_POINT('Ctrl Pts',(95.2520667038249,-0.325989900197102,
2.18102252395255));
#12929=CARTESIAN_POINT('Ctrl Pts',(95.2480394610563,-0.252230387745128,
2.18951954352957));
#12930=CARTESIAN_POINT('Ctrl Pts',(95.2440061136435,-0.178359067883193,
2.19802944320463));
#12931=CARTESIAN_POINT('Ctrl Pts',(95.2399727662307,-0.1041687412949,2.20278370595594));
#12932=CARTESIAN_POINT('Ctrl Pts',(95.2359394188179,-0.0300731305126705,
2.20379481958307));
#12933=CARTESIAN_POINT('Ctrl Pts',(95.235377895031,-0.0197575182690645,
2.20393558711304));
#12934=CARTESIAN_POINT('Ctrl Pts',(95.2348163712442,-0.00944373356853099,
2.20400388601063));
#12935=CARTESIAN_POINT('Ctrl Pts',(95.2342548474574,0.000867116891639564,
2.20399982942565));
#12936=CARTESIAN_POINT('',(94.484254847381,-0.00201577163552605,2.20399907819053));
#12937=CARTESIAN_POINT('Ctrl Pts',(95.23425484741,0.000867117761720935,
2.20399982942531));
#12938=CARTESIAN_POINT('Ctrl Pts',(95.2316329348932,0.0490113789919599,
2.20398088806992));
#12939=CARTESIAN_POINT('Ctrl Pts',(95.2290110223763,0.0971228006821106,
2.20238457773465));
#12940=CARTESIAN_POINT('Ctrl Pts',(95.2263891098594,0.145129365900741,2.19921655758437));
#12941=CARTESIAN_POINT('Ctrl Pts',(95.2223160449234,0.219706170516748,2.19429513030269));
#12942=CARTESIAN_POINT('Ctrl Pts',(95.2182429799874,0.294176174713683,2.18556649358735));
#12943=CARTESIAN_POINT('Ctrl Pts',(95.2141699150513,0.368119487752487,2.17304027637245));
#12944=CARTESIAN_POINT('Ctrl Pts',(95.2101028342462,0.441954163567666,2.16053246262643));
#12945=CARTESIAN_POINT('Ctrl Pts',(95.2060357534412,0.515263217712541,2.14423822483221));
#12946=CARTESIAN_POINT('Ctrl Pts',(95.2019686726361,0.587630216226328,2.1242190868594));
#12947=CARTESIAN_POINT('Ctrl Pts',(95.1979063502672,0.659912546212096,2.10422337104005));
#12948=CARTESIAN_POINT('Ctrl Pts',(95.1938440278984,0.731254552509463,2.08051154023093));
#12949=CARTESIAN_POINT('Ctrl Pts',(95.1897817055295,0.801249978189934,2.05319616024642));
#12950=CARTESIAN_POINT('Ctrl Pts',(95.1857219613902,0.8712009799524,2.02589811648336));
#12951=CARTESIAN_POINT('Ctrl Pts',(95.1816622172509,0.939806653360161,1.99500123510716));
#12952=CARTESIAN_POINT('Ctrl Pts',(95.1776024731116,1.00667718739468,1.96066749867976));
#12953=CARTESIAN_POINT('Ctrl Pts',(95.1735439936566,1.07352689003975,1.92634445783667));
#12954=CARTESIAN_POINT('Ctrl Pts',(95.1694855142016,1.13864210203628,1.88858690559608));
#12955=CARTESIAN_POINT('Ctrl Pts',(95.1654270347466,1.20165571726809,1.847603728389));
#12956=CARTESIAN_POINT('Ctrl Pts',(95.1613685081143,1.26467006499454,1.8066200747776));
#12957=CARTESIAN_POINT('Ctrl Pts',(95.1573099814819,1.32558236817435,1.7624109835724));
#12958=CARTESIAN_POINT('Ctrl Pts',(95.1532514548496,1.38405409633897,1.71522892303252));
#12959=CARTESIAN_POINT('Ctrl Pts',(95.1491887778645,1.44258561918211,1.6679986129158));
#12960=CARTESIAN_POINT('Ctrl Pts',(95.1451261008795,1.49867121064966,1.61778956278921));
#12961=CARTESIAN_POINT('Ctrl Pts',(95.1410634238944,1.55200567708095,1.56489436650162));
#12962=CARTESIAN_POINT('Ctrl Pts',(95.1369986249174,1.60536800083603,1.51197154232707));
#12963=CARTESIAN_POINT('Ctrl Pts',(95.1329338259405,1.65597601635295,1.45636013148767));
#12964=CARTESIAN_POINT('Ctrl Pts',(95.1288690269635,1.70356348513045,1.39838744707259));
#12965=CARTESIAN_POINT('Ctrl Pts',(95.1247969667215,1.751235963086,1.34031120156511));
#12966=CARTESIAN_POINT('Ctrl Pts',(95.1207249064795,1.79587683246783,1.27986564174607));
#12967=CARTESIAN_POINT('Ctrl Pts',(95.1166528462376,1.83726228457379,1.21740843503021));
#12968=CARTESIAN_POINT('Ctrl Pts',(95.1135146954386,1.86915616184366,1.16927551913227));
#12969=CARTESIAN_POINT('Ctrl Pts',(95.1103765446396,1.89911748674715,1.11994850694536));
#12970=CARTESIAN_POINT('Ctrl Pts',(95.1072383938406,1.92706285005977,1.0696002860506));
#12971=CARTESIAN_POINT('Ctrl Pts',(95.1031653289046,1.96333366262495,1.00425238333646));
#12972=CARTESIAN_POINT('Ctrl Pts',(95.0990922639686,1.99634667105031,0.936931421528423));
#12973=CARTESIAN_POINT('Ctrl Pts',(95.0950191990326,2.02588246297701,0.867995533515123));
#12974=CARTESIAN_POINT('Ctrl Pts',(95.0909521182276,2.05537486103475,0.7991609258365));
#12975=CARTESIAN_POINT('Ctrl Pts',(95.0868850374225,2.08139999899706,0.728716537848663));
#12976=CARTESIAN_POINT('Ctrl Pts',(95.0828179566175,2.10378395485132,0.657045714779518));
#12977=CARTESIAN_POINT('Ctrl Pts',(95.0787556342486,2.12614172174337,0.585458745721258));
#12978=CARTESIAN_POINT('Ctrl Pts',(95.0746933118797,2.14486662882977,0.512648645889528));
#12979=CARTESIAN_POINT('Ctrl Pts',(95.0706309895108,2.1598331686819,0.439017862349023));
#12980=CARTESIAN_POINT('Ctrl Pts',(95.0665712453715,2.17479020973704,0.365433809974987));
#12981=CARTESIAN_POINT('Ctrl Pts',(95.0625115012322,2.18599352210005,0.291030574194199));
#12982=CARTESIAN_POINT('Ctrl Pts',(95.0584517570929,2.19336804356406,0.216223554387558));
#12983=CARTESIAN_POINT('Ctrl Pts',(95.0543932776378,2.20074026773029,0.141439838330293));
#12984=CARTESIAN_POINT('Ctrl Pts',(95.0503347981827,2.20428602231726,0.0662530628375085));
#12985=CARTESIAN_POINT('Ctrl Pts',(95.0462763187276,2.2039819695306,-0.00891504256971563));
#12986=CARTESIAN_POINT('Ctrl Pts',(95.0422177920952,2.20367791320951,-0.0840840217600974));
#12987=CARTESIAN_POINT('Ctrl Pts',(95.0381592654628,2.199523964383,-0.159233852984441));
#12988=CARTESIAN_POINT('Ctrl Pts',(95.0341007388304,2.19154889840338,-0.233943210858857));
#12989=CARTESIAN_POINT('Ctrl Pts',(95.0300380618453,2.18356567691815,-0.308728968425563));
#12990=CARTESIAN_POINT('Ctrl Pts',(95.0259753848602,2.17175358587468,-0.383072877322738));
#12991=CARTESIAN_POINT('Ctrl Pts',(95.021912707875,2.15619318851793,-0.456559890692193));
#12992=CARTESIAN_POINT('Ctrl Pts',(95.017847908898,2.14062466375209,-0.530085287337291));
#12993=CARTESIAN_POINT('Ctrl Pts',(95.0137831099209,2.12130405671947,-0.602752435307004));
#12994=CARTESIAN_POINT('Ctrl Pts',(95.0097183109438,2.09836221869048,-0.674160217731919));
#12995=CARTESIAN_POINT('Ctrl Pts',(95.0056462507018,2.07537939788088,-0.745695561404457));
#12996=CARTESIAN_POINT('Ctrl Pts',(95.0015741904597,2.04876259435406,-0.815966598760288));
#12997=CARTESIAN_POINT('Ctrl Pts',(94.9975021302177,2.01869116135146,-0.884591428333714));
#12998=CARTESIAN_POINT('Ctrl Pts',(94.9943639794188,1.99551648173194,-0.937477449401332));
#12999=CARTESIAN_POINT('Ctrl Pts',(94.99122582862,1.97029107455252,-0.989386157279503));
#13000=CARTESIAN_POINT('Ctrl Pts',(94.9880876778211,1.94311505799379,-1.04015377295754));
#13001=CARTESIAN_POINT('Ctrl Pts',(94.9840146128851,1.90784279504664,-1.10604601605083));
#13002=CARTESIAN_POINT('Ctrl Pts',(94.9799415479491,1.86914704219674,-1.1702691375526));
#13003=CARTESIAN_POINT('Ctrl Pts',(94.9758684830131,1.82720992594269,-1.23244467889496));
#13004=CARTESIAN_POINT('Ctrl Pts',(94.971801402208,1.78533442353437,-1.29452887217732));
#13005=CARTESIAN_POINT('Ctrl Pts',(94.967734321403,1.74022727740138,-1.35457106544739));
#13006=CARTESIAN_POINT('Ctrl Pts',(94.9636672405979,1.69211645247092,-1.41221737394681));
#13007=CARTESIAN_POINT('Ctrl Pts',(94.9596049182291,1.64406191663366,-1.46979623695062));
#13008=CARTESIAN_POINT('Ctrl Pts',(94.9555425958602,1.59301098844483,-1.52498441968892));
#13009=CARTESIAN_POINT('Ctrl Pts',(94.9514802734913,1.53923391983028,-1.57745837981352));
#13010=CARTESIAN_POINT('Ctrl Pts',(94.947420529352,1.48549098184732,-1.62989903634894));
#13011=CARTESIAN_POINT('Ctrl Pts',(94.9433607852127,1.42902567769116,-1.67962855604401));
#13012=CARTESIAN_POINT('Ctrl Pts',(94.9393010410734,1.37014647789114,-1.72635877763647));
#13013=CARTESIAN_POINT('Ctrl Pts',(94.9352425616184,1.31128562003442,-1.77307444191366));
#13014=CARTESIAN_POINT('Ctrl Pts',(94.9311840821634,1.2500127332865,-1.81679236654611));
#13015=CARTESIAN_POINT('Ctrl Pts',(94.9271256027083,1.18666963397142,-1.85726443454079));
#13016=CARTESIAN_POINT('Ctrl Pts',(94.9230670760759,1.1233257983316,-1.89773697299848));
#13017=CARTESIAN_POINT('Ctrl Pts',(94.9190085494436,1.05791210565424,-1.93496332434018));
#13018=CARTESIAN_POINT('Ctrl Pts',(94.9149500228112,0.990798268561067,-1.96873939134066));
#13019=CARTESIAN_POINT('Ctrl Pts',(94.9108873458261,0.923615799148664,-2.00254999860755));
#13020=CARTESIAN_POINT('Ctrl Pts',(94.906824668841,0.854730140856377,-2.03290306050522));
#13021=CARTESIAN_POINT('Ctrl Pts',(94.9027619918559,0.784533788984808,-2.05964140906643));
#13022=CARTESIAN_POINT('Ctrl Pts',(94.8986971928789,0.714300772595258,-2.08639372343405));
#13023=CARTESIAN_POINT('Ctrl Pts',(94.8946323939019,0.642756154050088,-2.10952741763499));
#13024=CARTESIAN_POINT('Ctrl Pts',(94.8905675949248,0.570307967659544,-2.12893513805002));
#13025=CARTESIAN_POINT('Ctrl Pts',(94.8864955346828,0.497730361467263,-2.14837752797789));
#13026=CARTESIAN_POINT('Ctrl Pts',(94.8824234744408,0.424246430975652,-2.16408054936068));
#13027=CARTESIAN_POINT('Ctrl Pts',(94.8783514141988,0.350274339422994,-2.17598802550515));
#13028=CARTESIAN_POINT('Ctrl Pts',(94.8752132634,0.293267427834428,-2.18516457338371));
#13029=CARTESIAN_POINT('Ctrl Pts',(94.8720751126011,0.235970816031289,-2.19208796827572));
#13030=CARTESIAN_POINT('Ctrl Pts',(94.8689369618022,0.178576405409072,-2.19675362010199));
#13031=CARTESIAN_POINT('Ctrl Pts',(94.8648638968662,0.10408312053836,-2.20280925734669));
#13032=CARTESIAN_POINT('Ctrl Pts',(94.8607908319302,0.0291378055903611,
-2.20508310681169));
#13033=CARTESIAN_POINT('Ctrl Pts',(94.8567177669943,-0.0458427673246245,
-2.20352318814303));
#13034=CARTESIAN_POINT('Ctrl Pts',(94.8526506861892,-0.120713179077782,
-2.20196556130072));
#13035=CARTESIAN_POINT('Ctrl Pts',(94.8485836053841,-0.195618272557399,
-2.19658535909733));
#13036=CARTESIAN_POINT('Ctrl Pts',(94.8445165245791,-0.270137093596187,
-2.18738244270713));
#13037=CARTESIAN_POINT('Ctrl Pts',(94.8404542022102,-0.344568728500258,
-2.1781902936197));
#13038=CARTESIAN_POINT('Ctrl Pts',(94.8363918798413,-0.41861451737398,-2.16518437446876));
#13039=CARTESIAN_POINT('Ctrl Pts',(94.8323295574724,-0.491856096706097,
-2.14841652854679));
#13040=CARTESIAN_POINT('Ctrl Pts',(94.8282698133331,-0.565051191887526,
-2.13165932465471));
#13041=CARTESIAN_POINT('Ctrl Pts',(94.8242100691938,-0.637442626134506,
-2.11114503816434));
#13042=CARTESIAN_POINT('Ctrl Pts',(94.8201503250545,-0.708621065909673,
-2.08697680508171));
#13043=CARTESIAN_POINT('Ctrl Pts',(94.8160918455994,-0.779777332304277,
-2.06281610084392));
#13044=CARTESIAN_POINT('Ctrl Pts',(94.8120333661444,-0.849720902656972,
-2.03500386341315));
#13045=CARTESIAN_POINT('Ctrl Pts',(94.8079748866893,-0.918058032970696,
-2.00369295254986));
#13046=CARTESIAN_POINT('Ctrl Pts',(94.8039163600569,-0.986395957661693,
-1.97238167771642));
#13047=CARTESIAN_POINT('Ctrl Pts',(94.7998578334245,-1.05312697191543,-1.93757184921118));
#13048=CARTESIAN_POINT('Ctrl Pts',(94.7957993067921,-1.11787921530799,-1.89946362428513));
#13049=CARTESIAN_POINT('Ctrl Pts',(94.791736629807,-1.18269767599392,-1.86131642891763));
#13050=CARTESIAN_POINT('Ctrl Pts',(94.7876739528219,-1.24553291251983,-1.81986434410088));
#13051=CARTESIAN_POINT('Ctrl Pts',(94.7836112758368,-1.30604016410821,-1.77535210303089));
#13052=CARTESIAN_POINT('Ctrl Pts',(94.7795464768597,-1.36657901946451,-1.73081661260649));
#13053=CARTESIAN_POINT('Ctrl Pts',(94.7754816778827,-1.42478709850043,-1.68321808547488));
#13054=CARTESIAN_POINT('Ctrl Pts',(94.7714168789056,-1.4803530897551,-1.63284130571606));
#13055=CARTESIAN_POINT('Ctrl Pts',(94.7673448186636,-1.53601834283991,-1.58237453401717));
#13056=CARTESIAN_POINT('Ctrl Pts',(94.7632727584216,-1.5890317434293,-1.52911993535198));
#13057=CARTESIAN_POINT('Ctrl Pts',(94.7592006981796,-1.63911950591113,-1.47339853581495));
#13058=CARTESIAN_POINT('Ctrl Pts',(94.7560625473807,-1.67771985622653,-1.43045659879045));
#13059=CARTESIAN_POINT('Ctrl Pts',(94.7529243965818,-1.71458341002876,-1.38605036587126));
#13060=CARTESIAN_POINT('Ctrl Pts',(94.7497862457829,-1.74960233326733,-1.34033864206981));
#13061=CARTESIAN_POINT('Ctrl Pts',(94.7457131808469,-1.79505405228274,-1.28100853612167));
#13062=CARTESIAN_POINT('Ctrl Pts',(94.7416401159109,-1.83757211974619,-1.21924945125779));
#13063=CARTESIAN_POINT('Ctrl Pts',(94.7375670509749,-1.8768870307861,-1.15538351800038));
#13064=CARTESIAN_POINT('Ctrl Pts',(94.7334999701698,-1.91614418051386,-1.09161141632008));
#13065=CARTESIAN_POINT('Ctrl Pts',(94.7294328893648,-1.95220726905968,-1.02573901504703));
#13066=CARTESIAN_POINT('Ctrl Pts',(94.7253658085597,-1.98484809813193,-0.958120048502315));
#13067=CARTESIAN_POINT('Ctrl Pts',(94.7213034861908,-2.01745073782221,-0.890580195344562));
#13068=CARTESIAN_POINT('Ctrl Pts',(94.717241163822,-2.04663886656072,-0.821298264629233));
#13069=CARTESIAN_POINT('Ctrl Pts',(94.7131788414531,-2.07222938039574,-0.750653978224795));
#13070=CARTESIAN_POINT('Ctrl Pts',(94.7091190973138,-2.09780365272815,-0.680054527550057));
#13071=CARTESIAN_POINT('Ctrl Pts',(94.7050593531745,-2.11978467890283,-0.608094884757306));
#13072=CARTESIAN_POINT('Ctrl Pts',(94.7009996090352,-2.13803735882198,-0.535174973519425));
#13073=CARTESIAN_POINT('Ctrl Pts',(94.6969411295802,-2.15628435269885,-0.462277778162198));
#13074=CARTESIAN_POINT('Ctrl Pts',(94.6928826501251,-2.17080519046376,-0.388421371160504));
#13075=CARTESIAN_POINT('Ctrl Pts',(94.6888241706701,-2.18151501127954,-0.314019514619797));
#13076=CARTESIAN_POINT('Ctrl Pts',(94.6847656440377,-2.19222495659042,-0.23961679320304));
#13077=CARTESIAN_POINT('Ctrl Pts',(94.6807071174053,-2.1991237307389,-0.164669082503113));
#13078=CARTESIAN_POINT('Ctrl Pts',(94.6766485907729,-2.20217808312383,-0.0895973783602944));
#13079=CARTESIAN_POINT('Ctrl Pts',(94.6725859137878,-2.20523555896731,-0.0144489039807578));
#13080=CARTESIAN_POINT('Ctrl Pts',(94.6685232368027,-2.20444074280571,0.0608233389258848));
#13081=CARTESIAN_POINT('Ctrl Pts',(94.6644605598176,-2.19981253300626,0.135796979453149));
#13082=CARTESIAN_POINT('Ctrl Pts',(94.6603957608406,-2.19518190582931,0.210809779741819));
#13083=CARTESIAN_POINT('Ctrl Pts',(94.6563309618636,-2.1867139515811,0.285523192199072));
#13084=CARTESIAN_POINT('Ctrl Pts',(94.6522661628865,-2.17447935469135,0.359521259484193));
#13085=CARTESIAN_POINT('Ctrl Pts',(94.6481941026445,-2.1622229021944,0.433651515243245));
#13086=CARTESIAN_POINT('Ctrl Pts',(94.6441220424025,-2.14618646915675,0.507063406217915));
#13087=CARTESIAN_POINT('Ctrl Pts',(94.6400499821605,-2.12649153348655,0.579352878658624));
#13088=CARTESIAN_POINT('Ctrl Pts',(94.6369118313616,-2.11131354631698,0.635063072566992));
#13089=CARTESIAN_POINT('Ctrl Pts',(94.6337736805628,-2.09396379492343,0.69010688463997));
#13090=CARTESIAN_POINT('Ctrl Pts',(94.6306355297639,-2.07451732729691,0.744307637166844));
#13091=CARTESIAN_POINT('Ctrl Pts',(94.6265624648279,-2.04927739126605,0.814655813137714));
#13092=CARTESIAN_POINT('Ctrl Pts',(94.6224893998919,-2.02040639988904,0.88385434260875));
#13093=CARTESIAN_POINT('Ctrl Pts',(94.618416334956,-1.98802907873226,0.951502171366401));
#13094=CARTESIAN_POINT('Ctrl Pts',(94.6143492541509,-1.95569932620795,1.019050612201));
#13095=CARTESIAN_POINT('Ctrl Pts',(94.6102821733458,-1.91987367612162,1.0850524485454));
#13096=CARTESIAN_POINT('Ctrl Pts',(94.6062150925408,-1.88072579760258,1.14912422054021));
#13097=CARTESIAN_POINT('Ctrl Pts',(94.6021527701719,-1.841623721636,1.21312102932351));
#13098=CARTESIAN_POINT('Ctrl Pts',(94.598090447803,-1.79920738744258,1.2751918548093));
#13099=CARTESIAN_POINT('Ctrl Pts',(94.5940281254341,-1.75369673957379,1.33497705808311));
#13100=CARTESIAN_POINT('Ctrl Pts',(94.5899683812948,-1.70821497589665,1.39472431754928));
#13101=CARTESIAN_POINT('Ctrl Pts',(94.5859086371555,-1.65964308408925,1.45218845444174));
#13102=CARTESIAN_POINT('Ctrl Pts',(94.5818488930162,-1.60824399767617,1.50703923105491));
#13103=CARTESIAN_POINT('Ctrl Pts',(94.5777904135612,-1.55686092301483,1.56187292065197));
#13104=CARTESIAN_POINT('Ctrl Pts',(94.5737319341061,-1.50265272864739,1.61409451817641));
#13105=CARTESIAN_POINT('Ctrl Pts',(94.569673454651,-1.44592119988364,1.66340851378339));
#13106=CARTESIAN_POINT('Ctrl Pts',(94.5656149280186,-1.38918901165063,1.71272308263534));
#13107=CARTESIAN_POINT('Ctrl Pts',(94.5615564013863,-1.32993379230777,1.7591296705784));
#13108=CARTESIAN_POINT('Ctrl Pts',(94.5574978747539,-1.26849137056239,1.80237222648618));
#13109=CARTESIAN_POINT('Ctrl Pts',(94.5534351977688,-1.20698611623151,1.84565900333308));
#13110=CARTESIAN_POINT('Ctrl Pts',(94.5493725207836,-1.1432895842801,1.88577501138828));
#13111=CARTESIAN_POINT('Ctrl Pts',(94.5453098437985,-1.07776701453231,1.9225072853922));
#13112=CARTESIAN_POINT('Ctrl Pts',(94.5412450448215,-1.01221022144705,1.95925874516699));
#13113=CARTESIAN_POINT('Ctrl Pts',(94.5371802458444,-0.94482591951831,1.99262273928844));
#13114=CARTESIAN_POINT('Ctrl Pts',(94.5331154468674,-0.876002016757105,
2.02243330338419));
#13115=CARTESIAN_POINT('Ctrl Pts',(94.5290433866254,-0.807055168532504,
2.05229712039745));
#13116=CARTESIAN_POINT('Ctrl Pts',(94.5249713263834,-0.73666403069448,2.07859466087012));
#13117=CARTESIAN_POINT('Ctrl Pts',(94.5208992661413,-0.665234027303954,
2.10120910166432));
#13118=CARTESIAN_POINT('Ctrl Pts',(94.5177611153424,-0.610186186927786,
2.11863701805723));
#13119=CARTESIAN_POINT('Ctrl Pts',(94.5146229645435,-0.55452173018533,2.13387851983892));
#13120=CARTESIAN_POINT('Ctrl Pts',(94.5114848137447,-0.49842981621141,2.14690095680063));
#13121=CARTESIAN_POINT('Ctrl Pts',(94.5060042023378,-0.400468308540214,
2.16964394180405));
#13122=CARTESIAN_POINT('Ctrl Pts',(94.5005235909309,-0.300897817452928,
2.18569009051323));
#13123=CARTESIAN_POINT('Ctrl Pts',(94.4950429795241,-0.200495865891814,
2.19486159193702));
#13124=CARTESIAN_POINT('Ctrl Pts',(94.4914469354861,-0.134618208726679,
2.2008793736344));
#13125=CARTESIAN_POINT('Ctrl Pts',(94.487850891448,-0.0683829464465262,
2.20393837893462));
#13126=CARTESIAN_POINT('Ctrl Pts',(94.48425484741,-0.00201577217147137,
2.20399907819004));
#13127=CARTESIAN_POINT('',(93.734254847381,0.000279264059390885,2.20399998230753));
#13128=CARTESIAN_POINT('Ctrl Pts',(94.484254847381,-0.00201577163552312,
2.20399907819053));
#13129=CARTESIAN_POINT('Ctrl Pts',(94.4802443723136,0.0719999787032919,
2.20406677279694));
#13130=CARTESIAN_POINT('Ctrl Pts',(94.4762338972462,0.146123122639629,2.20040178212574));
#13131=CARTESIAN_POINT('Ctrl Pts',(94.4722234221788,0.21994154036407,2.19299833990413));
#13132=CARTESIAN_POINT('Ctrl Pts',(94.4682158556641,0.293706422096562,2.18560026694721));
#13133=CARTESIAN_POINT('Ctrl Pts',(94.4642082891495,0.367166528766565,2.17446916659792));
#13134=CARTESIAN_POINT('Ctrl Pts',(94.4602007226348,0.439911613805786,2.15965130797515));
#13135=CARTESIAN_POINT('Ctrl Pts',(94.4561946870196,0.512628910058618,2.14483910980777));
#13136=CARTESIAN_POINT('Ctrl Pts',(94.4521886514044,0.584631245720701,2.1263430451521));
#13137=CARTESIAN_POINT('Ctrl Pts',(94.4481826157892,0.655517147150896,2.10426074187377));
#13138=CARTESIAN_POINT('Ctrl Pts',(94.4441767355832,0.726400298648532,2.08217929525161));
#13139=CARTESIAN_POINT('Ctrl Pts',(94.4401708553773,0.796166633606758,2.0565120343155));
#13140=CARTESIAN_POINT('Ctrl Pts',(94.4361649751714,0.864430195458748,2.02740633252911));
#13141=CARTESIAN_POINT('Ctrl Pts',(94.4321552226181,0.932759745360509,1.99827249525659));
#13142=CARTESIAN_POINT('Ctrl Pts',(94.4281454700648,0.999583169482648,1.96569377490942));
#13143=CARTESIAN_POINT('Ctrl Pts',(94.4241357175115,1.06453577329586,1.92986517336663));
#13144=CARTESIAN_POINT('Ctrl Pts',(94.4201239061042,1.12952172777926,1.89401817521148));
#13145=CARTESIAN_POINT('Ctrl Pts',(94.4161120946968,1.19263453356797,1.85491823532025));
#13146=CARTESIAN_POINT('Ctrl Pts',(94.4121002832894,1.25353773672876,1.81280422070254));
#13147=CARTESIAN_POINT('Ctrl Pts',(94.4080815480228,1.31454605081407,1.77061752283039));
#13148=CARTESIAN_POINT('Ctrl Pts',(94.4040628127562,1.37333676154219,1.72540666685662));
#13149=CARTESIAN_POINT('Ctrl Pts',(94.4000440774896,1.42960639689859,1.67745090835667));
#13150=CARTESIAN_POINT('Ctrl Pts',(94.3974740842349,1.46559099745434,1.64678305698287));
#13151=CARTESIAN_POINT('Ctrl Pts',(94.3949040909802,1.50054528958034,1.61499341728707));
#13152=CARTESIAN_POINT('Ctrl Pts',(94.3923340977256,1.53439831437836,1.58216238510238));
#13153=CARTESIAN_POINT('Ctrl Pts',(94.3882610327896,1.58805042729019,1.53012998160833));
#13154=CARTESIAN_POINT('Ctrl Pts',(94.3841879678536,1.63915632778103,1.47526507881002));
#13155=CARTESIAN_POINT('Ctrl Pts',(94.3801149029176,1.68740223239212,1.41784685566464));
#13156=CARTESIAN_POINT('Ctrl Pts',(94.3760478221125,1.73557725431059,1.36051299114606));
#13157=CARTESIAN_POINT('Ctrl Pts',(94.3719807413075,1.78090031822109,1.30063361671115));
#13158=CARTESIAN_POINT('Ctrl Pts',(94.3679136605024,1.82309387238746,1.23852522479896));
#13159=CARTESIAN_POINT('Ctrl Pts',(94.3638513381335,1.86523806059701,1.176489498967));
#13160=CARTESIAN_POINT('Ctrl Pts',(94.3597890157646,1.90425974664773,1.11223032996636));
#13161=CARTESIAN_POINT('Ctrl Pts',(94.3557266933958,1.93992218009633,1.04609652287459));
#13162=CARTESIAN_POINT('Ctrl Pts',(94.3516669492565,1.97556197970846,0.980004688851698));
#13163=CARTESIAN_POINT('Ctrl Pts',(94.3476072051172,2.00784653142256,0.912040996903966));
#13164=CARTESIAN_POINT('Ctrl Pts',(94.3435474609778,2.03658361171268,0.842581267595792));
#13165=CARTESIAN_POINT('Ctrl Pts',(94.3394889815228,2.0653117398788,0.77314317625862));
#13166=CARTESIAN_POINT('Ctrl Pts',(94.3354305020678,2.09049440834122,0.702210413774042));
#13167=CARTESIAN_POINT('Ctrl Pts',(94.3313720226127,2.11198706389033,0.630179848900211));
#13168=CARTESIAN_POINT('Ctrl Pts',(94.3273134959803,2.13347996927842,0.558148446715127));
#13169=CARTESIAN_POINT('Ctrl Pts',(94.3232549693479,2.15128264178525,0.485019674843072));
#13170=CARTESIAN_POINT('Ctrl Pts',(94.3191964427155,2.16530052215873,0.411205117598434));
#13171=CARTESIAN_POINT('Ctrl Pts',(94.3151337657304,2.17933273757372,0.337315075707495));
#13172=CARTESIAN_POINT('Ctrl Pts',(94.3110710887453,2.18957234255911,0.262738318103916));
#13173=CARTESIAN_POINT('Ctrl Pts',(94.3070084117602,2.19597616291718,0.187895428096429));
#13174=CARTESIAN_POINT('Ctrl Pts',(94.3029436127832,2.20238332807852,0.113013446620275));
#13175=CARTESIAN_POINT('Ctrl Pts',(94.2988788138061,2.20495070255364,0.0378655335523711));
#13176=CARTESIAN_POINT('Ctrl Pts',(94.2948140148291,2.20368727908339,-0.0371264865839261));
#13177=CARTESIAN_POINT('Ctrl Pts',(94.2907419545871,2.20242159866202,-0.112252470769029));
#13178=CARTESIAN_POINT('Ctrl Pts',(94.2866698943451,2.19731148395123,-0.187221528710871));
#13179=CARTESIAN_POINT('Ctrl Pts',(94.282597834103,2.18841791692943,-0.261616170873024));
#13180=CARTESIAN_POINT('Ctrl Pts',(94.2794596833042,2.18156405112303,-0.318948722912514));
#13181=CARTESIAN_POINT('Ctrl Pts',(94.2763215325053,2.17246423506766,-0.375940200071185));
#13182=CARTESIAN_POINT('Ctrl Pts',(94.2731833817064,2.16116682758316,-0.432404837338979));
#13183=CARTESIAN_POINT('Ctrl Pts',(94.2691103167704,2.14650370995695,-0.505691351887988));
#13184=CARTESIAN_POINT('Ctrl Pts',(94.2650372518344,2.12808030290967,-0.578372495913159));
#13185=CARTESIAN_POINT('Ctrl Pts',(94.2609641868984,2.10596124041854,-0.650033271344486));
#13186=CARTESIAN_POINT('Ctrl Pts',(94.2568971060934,2.08387467516676,-0.721588763047257));
#13187=CARTESIAN_POINT('Ctrl Pts',(94.2528300252883,2.0581033741769,-0.79212641008916));
#13188=CARTESIAN_POINT('Ctrl Pts',(94.2487629444833,2.02876296428268,-0.861241449742725));
#13189=CARTESIAN_POINT('Ctrl Pts',(94.2447006221144,1.99945688231918,-0.930275625621683));
#13190=CARTESIAN_POINT('Ctrl Pts',(94.2406382997456,1.96659017347895,-0.997890063672327));
#13191=CARTESIAN_POINT('Ctrl Pts',(94.2365759773767,1.93032773015936,-1.0636967867667));
#13192=CARTESIAN_POINT('Ctrl Pts',(94.2325162332374,1.89408830148383,-1.12946174438226));
#13193=CARTESIAN_POINT('Ctrl Pts',(94.2284564890981,1.85445764487347,-1.19342084662097));
#13194=CARTESIAN_POINT('Ctrl Pts',(94.2243967449588,1.81164748468374,-1.25520890342567));
#13195=CARTESIAN_POINT('Ctrl Pts',(94.2203382655037,1.76885066063877,-1.31697771212511));
#13196=CARTESIAN_POINT('Ctrl Pts',(94.2162797860487,1.72287657129991,-1.37657642598749));
#13197=CARTESIAN_POINT('Ctrl Pts',(94.2122213065936,1.67398046066359,-1.433668517237));
#13198=CARTESIAN_POINT('Ctrl Pts',(94.2081627799612,1.62508378163987,-1.49076127214717));
#13199=CARTESIAN_POINT('Ctrl Pts',(94.2041042533288,1.57326532581928,-1.54534698511569));
#13200=CARTESIAN_POINT('Ctrl Pts',(94.2000457266964,1.51881979329052,-1.59712317480805));
#13201=CARTESIAN_POINT('Ctrl Pts',(94.1959830497113,1.46431858337352,-1.64895231215068));
#13202=CARTESIAN_POINT('Ctrl Pts',(94.1919203727262,1.40718527868952,-1.69796585906177));
#13203=CARTESIAN_POINT('Ctrl Pts',(94.1878576957411,1.34774998440714,-1.74389964720753));
#13204=CARTESIAN_POINT('Ctrl Pts',(94.1837928967641,1.28828364625489,-1.78985742720123));
#13205=CARTESIAN_POINT('Ctrl Pts',(94.179728097787,1.22651331672078,-1.83273197255615));
#13206=CARTESIAN_POINT('Ctrl Pts',(94.17566329881,1.16279840932539,-1.87230228843271));
#13207=CARTESIAN_POINT('Ctrl Pts',(94.171591238568,1.09896968306027,-1.9119432918267));
#13208=CARTESIAN_POINT('Ctrl Pts',(94.167519178326,1.03318985897519,-1.94826804460465));
#13209=CARTESIAN_POINT('Ctrl Pts',(94.163447118084,0.965842875895455,-1.98110159736496));
#13210=CARTESIAN_POINT('Ctrl Pts',(94.1603089672851,0.913941632742322,-2.00640491649622));
#13211=CARTESIAN_POINT('Ctrl Pts',(94.1571708164862,0.861110159100261,-2.02963572607796));
#13212=CARTESIAN_POINT('Ctrl Pts',(94.1540326656873,0.807530791185746,-2.05073402012229));
#13213=CARTESIAN_POINT('Ctrl Pts',(94.1499596007513,0.737989121989469,-2.07811789272372));
#13214=CARTESIAN_POINT('Ctrl Pts',(94.1458865358153,0.666918861211004,-2.10201326166652));
#13215=CARTESIAN_POINT('Ctrl Pts',(94.1418134708793,0.59470383234052,-2.12224959696062));
#13216=CARTESIAN_POINT('Ctrl Pts',(94.1377463900743,0.522594901505407,-2.14245620111078));
#13217=CARTESIAN_POINT('Ctrl Pts',(94.1336793092692,0.449344997747966,-2.15901431708036));
#13218=CARTESIAN_POINT('Ctrl Pts',(94.1296122284641,0.375356970788698,-2.17180181979856));
#13219=CARTESIAN_POINT('Ctrl Pts',(94.1255499060953,0.301455508941461,-2.18457436129059));
#13220=CARTESIAN_POINT('Ctrl Pts',(94.1214875837264,0.226818107780517,-2.19358497341288));
#13221=CARTESIAN_POINT('Ctrl Pts',(94.1174252613575,0.151860201920908,-2.19876203329795));
#13222=CARTESIAN_POINT('Ctrl Pts',(94.1133655172182,0.0769498695110541,
-2.20393580746425));
#13223=CARTESIAN_POINT('Ctrl Pts',(94.1093057730789,0.00171991117514311,
-2.20528082467623));
#13224=CARTESIAN_POINT('Ctrl Pts',(94.1052460289396,-0.0734080163565206,
-2.2027771705587));
#13225=CARTESIAN_POINT('Ctrl Pts',(94.1011875494846,-0.148512540170232,
-2.20027429637503));
#13226=CARTESIAN_POINT('Ctrl Pts',(94.0971290700296,-0.223514619401914,
-2.19392514718078));
#13227=CARTESIAN_POINT('Ctrl Pts',(94.0930705905745,-0.297993107967888,
-2.18376191641938));
#13228=CARTESIAN_POINT('Ctrl Pts',(94.0890120639421,-0.372472462300833,
-2.17359856751663));
#13229=CARTESIAN_POINT('Ctrl Pts',(94.0849535373097,-0.44642774104921,-2.15962111534711));
#13230=CARTESIAN_POINT('Ctrl Pts',(94.0808950106773,-0.519445035845304,
-2.14191336303214));
#13231=CARTESIAN_POINT('Ctrl Pts',(94.0768323336922,-0.592536999986773,
-2.12418750231866));
#13232=CARTESIAN_POINT('Ctrl Pts',(94.0727696567071,-0.664688599654287,
-2.102723836501));
#13233=CARTESIAN_POINT('Ctrl Pts',(94.068706979722,-0.735498945136245,-2.07765668523543));
#13234=CARTESIAN_POINT('Ctrl Pts',(94.064642180745,-0.806346275833395,-2.05257644105275));
#13235=CARTESIAN_POINT('Ctrl Pts',(94.060577381768,-0.875850515500875,-2.02388914563516));
#13236=CARTESIAN_POINT('Ctrl Pts',(94.0565125827909,-0.943631181632175,
-1.99177714442441));
#13237=CARTESIAN_POINT('Ctrl Pts',(94.0524405225489,-1.01153292961262,-1.9596077790609));
#13238=CARTESIAN_POINT('Ctrl Pts',(94.0483684623069,-1.07770453300776,-1.92400171461756));
#13239=CARTESIAN_POINT('Ctrl Pts',(94.0442964020649,-1.14179092192146,-1.88518685827632));
#13240=CARTESIAN_POINT('Ctrl Pts',(94.041158251266,-1.19117937410965,-1.85527402172717));
#13241=CARTESIAN_POINT('Ctrl Pts',(94.038020100467,-1.23932991199915,-1.82345640361977));
#13242=CARTESIAN_POINT('Ctrl Pts',(94.0348819496681,-1.28609330739947,-1.78985474401201));
#13243=CARTESIAN_POINT('Ctrl Pts',(94.0308088847321,-1.34678839769241,-1.74624251811552));
#13244=CARTESIAN_POINT('Ctrl Pts',(94.0267358197961,-1.40537964316221,-1.69945537695057));
#13245=CARTESIAN_POINT('Ctrl Pts',(94.0226627548601,-1.46151575089349,-1.64972352528848));
#13246=CARTESIAN_POINT('Ctrl Pts',(94.018595674055,-1.51756938367673,-1.60006473946667));
#13247=CARTESIAN_POINT('Ctrl Pts',(94.01452859325,-1.57117468582549,-1.54747014671698));
#13248=CARTESIAN_POINT('Ctrl Pts',(94.0104615124449,-1.62201073967655,-1.49221217002607));
#13249=CARTESIAN_POINT('Ctrl Pts',(94.006399190076,-1.67278731594906,-1.43701884451085));
#13250=CARTESIAN_POINT('Ctrl Pts',(94.0023368677071,-1.72080075940068,-1.37916867570505));
#13251=CARTESIAN_POINT('Ctrl Pts',(93.9982745453383,-1.76576578042336,-1.31897202725679));
#13252=CARTESIAN_POINT('Ctrl Pts',(93.9942148011989,-1.81070226354682,-1.25881358374756));
#13253=CARTESIAN_POINT('Ctrl Pts',(93.9901550570596,-1.85259387851181,-1.19631199738186));
#13254=CARTESIAN_POINT('Ctrl Pts',(93.9860953129203,-1.89119542512883,-1.13181087818229));
#13255=CARTESIAN_POINT('Ctrl Pts',(93.9820368334652,-1.92978494666091,-1.06732985225632));
#13256=CARTESIAN_POINT('Ctrl Pts',(93.9779783540101,-1.9650861897439,-1.00085093964909));
#13257=CARTESIAN_POINT('Ctrl Pts',(93.9739198745551,-1.99689802718692,-0.932745554273499));
#13258=CARTESIAN_POINT('Ctrl Pts',(93.9698613479227,-2.02871023442301,-0.864639377214648));
#13259=CARTESIAN_POINT('Ctrl Pts',(93.9658028212903,-2.05703275504176,-0.794907123201642));
#13260=CARTESIAN_POINT('Ctrl Pts',(93.9617442946579,-2.08171176103076,-0.723942086071967));
#13261=CARTESIAN_POINT('Ctrl Pts',(93.9576816176728,-2.10641600439989,-0.652904478287715));
#13262=CARTESIAN_POINT('Ctrl Pts',(93.9536189406876,-2.12746913544939,-0.580632021860763));
#13263=CARTESIAN_POINT('Ctrl Pts',(93.9495562637025,-2.14476683879704,-0.507534439419188));
#13264=CARTESIAN_POINT('Ctrl Pts',(93.9454914647255,-2.16207357697252,-0.434398677107195));
#13265=CARTESIAN_POINT('Ctrl Pts',(93.9414266657484,-2.17562089518297,-0.360437400620822));
#13266=CARTESIAN_POINT('Ctrl Pts',(93.9373618667714,-2.18535590048339,-0.286069201806934));
#13267=CARTESIAN_POINT('Ctrl Pts',(93.9332898065293,-2.19510829617712,-0.211568153324482));
#13268=CARTESIAN_POINT('Ctrl Pts',(93.9292177462873,-2.20103473834352,-0.136659207234329));
#13269=CARTESIAN_POINT('Ctrl Pts',(93.9251456860453,-2.20313439749033,-0.0617642825176407));
#13270=CARTESIAN_POINT('Ctrl Pts',(93.9220075352465,-2.20475250887302,-0.00404618557138921));
#13271=CARTESIAN_POINT('Ctrl Pts',(93.9188693844478,-2.20409893500785,0.0536635013265952));
#13272=CARTESIAN_POINT('Ctrl Pts',(93.9157312336491,-2.20119430231718,0.111173933304467));
#13273=CARTESIAN_POINT('Ctrl Pts',(93.9116581687131,-2.19742432492508,0.185817804477317));
#13274=CARTESIAN_POINT('Ctrl Pts',(93.9075851037772,-2.18984594332277,0.260413640529149));
#13275=CARTESIAN_POINT('Ctrl Pts',(93.9035120388412,-2.17846230557427,0.334541452128176));
#13276=CARTESIAN_POINT('Ctrl Pts',(93.8994449580361,-2.16709539262136,0.408560355439342));
#13277=CARTESIAN_POINT('Ctrl Pts',(93.8953778772311,-2.15193439514934,0.482112131492625));
#13278=CARTESIAN_POINT('Ctrl Pts',(93.891310796426,-2.13303440332286,0.554779446483994));
#13279=CARTESIAN_POINT('Ctrl Pts',(93.8872484740572,-2.11415652426219,0.627361741580495));
#13280=CARTESIAN_POINT('Ctrl Pts',(93.8831861516883,-2.09154846171698,0.69906117177914));
#13281=CARTESIAN_POINT('Ctrl Pts',(93.8791238293194,-2.06531649876985,0.769469791420714));
#13282=CARTESIAN_POINT('Ctrl Pts',(93.8750640851802,-2.03910118443314,0.83983372490286));
#13283=CARTESIAN_POINT('Ctrl Pts',(93.8710043410409,-2.00926670002053,0.908908027232522));
#13284=CARTESIAN_POINT('Ctrl Pts',(93.8669445969016,-1.97596899326979,0.976300434106421));
#13285=CARTESIAN_POINT('Ctrl Pts',(93.8628861174465,-1.94268165936119,1.04367184701807));
#13286=CARTESIAN_POINT('Ctrl Pts',(93.8588276379915,-1.90593345650014,1.10936197695432));
#13287=CARTESIAN_POINT('Ctrl Pts',(93.8547691585364,-1.8659275810886,1.17300053799342));
#13288=CARTESIAN_POINT('Ctrl Pts',(93.8507106319041,-1.82592124063332,1.23663983879172));
#13289=CARTESIAN_POINT('Ctrl Pts',(93.8466521052717,-1.78265740806778,1.29822712007275));
#13290=CARTESIAN_POINT('Ctrl Pts',(93.8425935786393,-1.73638329740971,1.35741999560807));
#13291=CARTESIAN_POINT('Ctrl Pts',(93.8385309016542,-1.69006186566747,1.41667340328554));
#13292=CARTESIAN_POINT('Ctrl Pts',(93.8344682246692,-1.64072430318569,1.47352713854738));
#13293=CARTESIAN_POINT('Ctrl Pts',(93.8304055476841,-1.58865845924492,1.52767152878803));
#13294=CARTESIAN_POINT('Ctrl Pts',(93.826340748707,-1.53656542059916,1.58184419938694));
#13295=CARTESIAN_POINT('Ctrl Pts',(93.82227594973,-1.48174161115821,1.63330437980348));
#13296=CARTESIAN_POINT('Ctrl Pts',(93.8182111507529,-1.42451019646175,1.68178081216802));
#13297=CARTESIAN_POINT('Ctrl Pts',(93.8141390905109,-1.36717654486046,1.73034384173495));
#13298=CARTESIAN_POINT('Ctrl Pts',(93.810067030269,-1.30742707751986,1.77591218681686));
#13299=CARTESIAN_POINT('Ctrl Pts',(93.805994970027,-1.2456159654642,1.81825654586494));
#13300=CARTESIAN_POINT('Ctrl Pts',(93.8028568192279,-1.19798096520409,1.85088940890829));
#13301=CARTESIAN_POINT('Ctrl Pts',(93.7997186684289,-1.14912218783894,1.88160837691966));
#13302=CARTESIAN_POINT('Ctrl Pts',(93.7965805176298,-1.09921121319741,1.91032738261825));
#13303=CARTESIAN_POINT('Ctrl Pts',(93.7923397722511,-1.0317639333775,1.94913685944001));
#13304=CARTESIAN_POINT('Ctrl Pts',(93.7880990268724,-0.962152378046453,
1.98443203271001));
#13305=CARTESIAN_POINT('Ctrl Pts',(93.7838582814936,-0.890761497316347,
2.01597617914963));
#13306=CARTESIAN_POINT('Ctrl Pts',(93.7796285982377,-0.819556842030956,
2.04743804165272));
#13307=CARTESIAN_POINT('Ctrl Pts',(93.7753989149819,-0.746582486492347,
2.07516819060959));
#13308=CARTESIAN_POINT('Ctrl Pts',(93.771169231726,-0.672247882970542,2.09897565108355));
#13309=CARTESIAN_POINT('Ctrl Pts',(93.7669460737044,-0.598027957232878,
2.12274638321454));
#13310=CARTESIAN_POINT('Ctrl Pts',(93.7627229156828,-0.522452354479371,
2.14260632975068));
#13311=CARTESIAN_POINT('Ctrl Pts',(93.7584997576612,-0.445950619526727,
2.15841238991619));
#13312=CARTESIAN_POINT('Ctrl Pts',(93.7542842631783,-0.369587708175099,
2.17418976767089));
#13313=CARTESIAN_POINT('Ctrl Pts',(93.7500687686954,-0.292302421946365,
2.18592782015334));
#13314=CARTESIAN_POINT('Ctrl Pts',(93.7458532742125,-0.214538074458878,
2.19353354535723));
#13315=CARTESIAN_POINT('Ctrl Pts',(93.741987131945,-0.143218320170691,2.20050895851572));
#13316=CARTESIAN_POINT('Ctrl Pts',(93.7381209896775,-0.071496035973098,
2.20400907678262));
#13317=CARTESIAN_POINT('Ctrl Pts',(93.73425484741,0.00027926351991633,2.2039999823076));
#13318=CARTESIAN_POINT('',(92.9842548474409,0.00188421767977092,2.20399919458328));
#13319=CARTESIAN_POINT('Ctrl Pts',(93.734254847381,0.00027926405938751,
2.20399998230753));
#13320=CARTESIAN_POINT('Ctrl Pts',(93.7299610335033,0.0799943277350516,
2.20398988178464));
#13321=CARTESIAN_POINT('Ctrl Pts',(93.7256672196257,0.15960883666517,2.19965076805581));
#13322=CARTESIAN_POINT('Ctrl Pts',(93.7213734057481,0.23865534179794,2.19104076361699));
#13323=CARTESIAN_POINT('Ctrl Pts',(93.7170655055175,0.3179611681322,2.18240251306289));
#13324=CARTESIAN_POINT('Ctrl Pts',(93.7127576052869,0.396694877691193,2.16946540440215));
#13325=CARTESIAN_POINT('Ctrl Pts',(93.7084497050562,0.474397220033825,2.15233902478773));
#13326=CARTESIAN_POINT('Ctrl Pts',(93.7041342620763,0.552235612252334,2.13518265840906));
#13327=CARTESIAN_POINT('Ctrl Pts',(93.6998188190963,0.629038661404861,2.11382249435064));
#13328=CARTESIAN_POINT('Ctrl Pts',(93.6955033761164,0.704363112905398,2.08841772765369));
#13329=CARTESIAN_POINT('Ctrl Pts',(93.6911756325087,0.779902267285068,2.06294054786319));
#13330=CARTESIAN_POINT('Ctrl Pts',(93.6868478889011,0.853954037648477,2.03339586354069));
#13331=CARTESIAN_POINT('Ctrl Pts',(93.6825201452935,0.926095192750267,1.99999092347062));
#13332=CARTESIAN_POINT('Ctrl Pts',(93.6808233640659,0.954379621961421,1.98689382707146));
#13333=CARTESIAN_POINT('Ctrl Pts',(93.6791265828383,0.982370638153006,1.97320382397862));
#13334=CARTESIAN_POINT('Ctrl Pts',(93.6774298016107,1.01004390129631,1.95893525096011));
#13335=CARTESIAN_POINT('Ctrl Pts',(93.6733567366746,1.07647261699902,1.92468403253235));
#13336=CARTESIAN_POINT('Ctrl Pts',(93.6692836717384,1.14128524091617,1.88698397410478));
#13337=CARTESIAN_POINT('Ctrl Pts',(93.6652106068023,1.20410054898345,1.84601134014332));
#13338=CARTESIAN_POINT('Ctrl Pts',(93.661143525997,1.26682356904803,1.80509890301399));
#13339=CARTESIAN_POINT('Ctrl Pts',(93.6570764451918,1.327554702752,1.76092369498526));
#13340=CARTESIAN_POINT('Ctrl Pts',(93.6530093643866,1.38593658953909,1.71370819271449));
#13341=CARTESIAN_POINT('Ctrl Pts',(93.6489470420176,1.4442501702127,1.66654793202006));
#13342=CARTESIAN_POINT('Ctrl Pts',(93.6448847196485,1.50021959541092,1.61635474297736));
#13343=CARTESIAN_POINT('Ctrl Pts',(93.6408223972795,1.55351719080458,1.56339385244879));
#13344=CARTESIAN_POINT('Ctrl Pts',(93.6367626531401,1.60678095987339,1.51046657454895));
#13345=CARTESIAN_POINT('Ctrl Pts',(93.6327029090006,1.65737592629956,1.45477541658576));
#13346=CARTESIAN_POINT('Ctrl Pts',(93.6286431648611,1.70500920283994,1.39662436547237));
#13347=CARTESIAN_POINT('Ctrl Pts',(93.6245846854059,1.75262764074699,1.3384914294707));
#13348=CARTESIAN_POINT('Ctrl Pts',(93.6205262059507,1.79728591823297,1.27790049089922));
#13349=CARTESIAN_POINT('Ctrl Pts',(93.6164677264955,1.83873067296567,1.21518949645527));
#13350=CARTESIAN_POINT('Ctrl Pts',(93.612409199863,1.88017590946827,1.1524777730344));
#13351=CARTESIAN_POINT('Ctrl Pts',(93.6083506732304,1.91840728729221,1.08764634412842));
#13352=CARTESIAN_POINT('Ctrl Pts',(93.6042921465978,1.95321502813759,1.02106172872038));
#13353=CARTESIAN_POINT('Ctrl Pts',(93.6002294696126,1.98805836426528,0.954409022188786));
#13354=CARTESIAN_POINT('Ctrl Pts',(93.5961667926273,2.01947085023301,0.885999973001929));
#13355=CARTESIAN_POINT('Ctrl Pts',(93.5921041156421,2.0472892798299,0.81622460431769));
#13356=CARTESIAN_POINT('Ctrl Pts',(93.5880393166649,2.07512223937437,0.746412791000746));
#13357=CARTESIAN_POINT('Ctrl Pts',(93.5839745176877,2.09935725020407,0.675233689428349));
#13358=CARTESIAN_POINT('Ctrl Pts',(93.5799097187105,2.11988067472745,0.603093628649058));
#13359=CARTESIAN_POINT('Ctrl Pts',(93.5758376584683,2.14044076183223,0.530824698496752));
#13360=CARTESIAN_POINT('Ctrl Pts',(93.5717655982262,2.15727591200396,0.457591846304882));
#13361=CARTESIAN_POINT('Ctrl Pts',(93.567693537984,2.17032350217403,0.383812318602512));
#13362=CARTESIAN_POINT('Ctrl Pts',(93.5645553871865,2.18037868384186,0.326953807203578));
#13363=CARTESIAN_POINT('Ctrl Pts',(93.5614172363891,2.18818545146171,0.269770859593916));
#13364=CARTESIAN_POINT('Ctrl Pts',(93.5582790855916,2.19373625409253,0.212455283483507));
#13365=CARTESIAN_POINT('Ctrl Pts',(93.5542060206558,2.20094074521493,0.13806431937878));
#13366=CARTESIAN_POINT('Ctrl Pts',(93.55013295572,2.20437087458598,0.0631630187489451));
#13367=CARTESIAN_POINT('Ctrl Pts',(93.5460598907842,2.20396823644446,-0.0118326980817148));
#13368=CARTESIAN_POINT('Ctrl Pts',(93.5419928099794,2.20356618985732,-0.0867182315011731));
#13369=CARTESIAN_POINT('Ctrl Pts',(93.5379257291745,2.19934255830485,-0.161697432223492));
#13370=CARTESIAN_POINT('Ctrl Pts',(93.5338586483697,2.19129070684363,-0.236349398350684));
#13371=CARTESIAN_POINT('Ctrl Pts',(93.529796326001,2.1832482759529,-0.310914022565039));
#13372=CARTESIAN_POINT('Ctrl Pts',(93.5257340036323,2.17138657479198,-0.385151700518907));
#13373=CARTESIAN_POINT('Ctrl Pts',(93.5216716812637,2.15575098432446,-0.458643318477556));
#13374=CARTESIAN_POINT('Ctrl Pts',(93.5176119371246,2.14012531727954,-0.532088293593804));
#13375=CARTESIAN_POINT('Ctrl Pts',(93.5135521929855,2.12073061298998,-0.604787682501735));
#13376=CARTESIAN_POINT('Ctrl Pts',(93.5094924488463,2.09766367837493,-0.676330608819784));
#13377=CARTESIAN_POINT('Ctrl Pts',(93.5054339693915,2.0746039295302,-0.747851248213083));
#13378=CARTESIAN_POINT('Ctrl Pts',(93.5013754899366,2.04787436807721,-0.818215686167462));
#13379=CARTESIAN_POINT('Ctrl Pts',(93.4973170104818,2.01762175934515,-0.887027866651888));
#13380=CARTESIAN_POINT('Ctrl Pts',(93.4932584838496,1.98736879894502,-0.955840847035797));
#13381=CARTESIAN_POINT('Ctrl Pts',(93.4891999572174,1.95359290375311,-1.02310109775934));
#13382=CARTESIAN_POINT('Ctrl Pts',(93.4851414305852,1.91648846866269,-1.0884337138673));
#13383=CARTESIAN_POINT('Ctrl Pts',(93.4810787536003,1.87934608963182,-1.15383314077262));
#13384=CARTESIAN_POINT('Ctrl Pts',(93.4770160766154,1.83886860972418,-1.21730058049374));
#13385=CARTESIAN_POINT('Ctrl Pts',(93.4729533996305,1.79529541266976,-1.27848753660211));
#13386=CARTESIAN_POINT('Ctrl Pts',(93.4688886006536,1.75169945673649,-1.33970645149742));
#13387=CARTESIAN_POINT('Ctrl Pts',(93.4648238016767,1.70500486046904,-1.39864213618045));
#13388=CARTESIAN_POINT('Ctrl Pts',(93.4607590026999,1.6554915698996,-1.45497892149383));
#13389=CARTESIAN_POINT('Ctrl Pts',(93.4566869424581,1.60588982990756,-1.51141634556652));
#13390=CARTESIAN_POINT('Ctrl Pts',(93.4526148822162,1.55345967172619,-1.56524525446865));
#13391=CARTESIAN_POINT('Ctrl Pts',(93.4485428219744,1.4985178581826,-1.61618694113888));
#13392=CARTESIAN_POINT('Ctrl Pts',(93.4454046711738,1.45617671244284,-1.65544537183887));
#13393=CARTESIAN_POINT('Ctrl Pts',(93.4422665203731,1.41234464305599,-1.69298980974854));
#13394=CARTESIAN_POINT('Ctrl Pts',(93.4391283695725,1.3671787720371,-1.72870998299054));
#13395=CARTESIAN_POINT('Ctrl Pts',(93.4350553046367,1.30855713871575,-1.77507186754473));
#13396=CARTESIAN_POINT('Ctrl Pts',(93.4309822397009,1.24746154382153,-1.81853793371124));
#13397=CARTESIAN_POINT('Ctrl Pts',(93.4269091747651,1.18420992053786,-1.85883373761607));
#13398=CARTESIAN_POINT('Ctrl Pts',(93.4228420939602,1.12105122628956,-1.89907033908478));
#13399=CARTESIAN_POINT('Ctrl Pts',(93.4187750131553,1.05574319202988,-1.93614567138971));
#13400=CARTESIAN_POINT('Ctrl Pts',(93.4147079323504,0.988635988417915,-1.96982610461049));
#13401=CARTESIAN_POINT('Ctrl Pts',(93.4106456099818,0.921607299436438,-2.00346713212477));
#13402=CARTESIAN_POINT('Ctrl Pts',(93.4065832876131,0.852784047856998,-2.03372093889994));
#13403=CARTESIAN_POINT('Ctrl Pts',(93.4025209652444,0.78254308468408,-2.06039858294776));
#13404=CARTESIAN_POINT('Ctrl Pts',(93.3984612211053,0.712346701264204,-2.08705929552526));
#13405=CARTESIAN_POINT('Ctrl Pts',(93.3944014769662,0.640734836982481,-2.11014818021287));
#13406=CARTESIAN_POINT('Ctrl Pts',(93.3903417328271,0.568105283034198,-2.12952398140726));
#13407=CARTESIAN_POINT('Ctrl Pts',(93.3862832533722,0.495498354515015,-2.14889374668663));
#13408=CARTESIAN_POINT('Ctrl Pts',(93.3822247739173,0.42187482680223,-2.16455260204706));
#13409=CARTESIAN_POINT('Ctrl Pts',(93.3781662944625,0.347647103164469,-2.17640931160969));
#13410=CARTESIAN_POINT('Ctrl Pts',(93.3741077678303,0.273418516674914,-2.1882661589993));
#13411=CARTESIAN_POINT('Ctrl Pts',(93.3700492411981,0.198586192081613,-2.19632069929357));
#13412=CARTESIAN_POINT('Ctrl Pts',(93.3659907145659,0.123570561972054,-2.20053318907348));
#13413=CARTESIAN_POINT('Ctrl Pts',(93.361928037581,0.0484782189684729,-2.20474998665274));
#13414=CARTESIAN_POINT('Ctrl Pts',(93.3578653605961,-0.0267973261153622,
-2.20511686094239));
#13415=CARTESIAN_POINT('Ctrl Pts',(93.3538026836112,-0.10183346103039,-2.20164619006201));
#13416=CARTESIAN_POINT('Ctrl Pts',(93.3497378846343,-0.176908788348498,
-2.1981737064026));
#13417=CARTESIAN_POINT('Ctrl Pts',(93.3456730856575,-0.251743980839748,
-2.1908597324871));
#13418=CARTESIAN_POINT('Ctrl Pts',(93.3416082866806,-0.325922039898365,
-2.17976852530458));
#13419=CARTESIAN_POINT('Ctrl Pts',(93.3375362264388,-0.400232608964159,
-2.16865750504037));
#13420=CARTESIAN_POINT('Ctrl Pts',(93.333464166197,-0.473883231174135,-2.15375586859984));
#13421=CARTESIAN_POINT('Ctrl Pts',(93.3293921059552,-0.546468026254893,
-2.13517884409739));
#13422=CARTESIAN_POINT('Ctrl Pts',(93.3262539551545,-0.60240581186443,-2.12086237998498));
#13423=CARTESIAN_POINT('Ctrl Pts',(93.3231158043539,-0.657710809498464,
-2.10436412670199));
#13424=CARTESIAN_POINT('Ctrl Pts',(93.3199776535533,-0.712205204349463,
-2.08575639682527));
#13425=CARTESIAN_POINT('Ctrl Pts',(93.3159045886161,-0.782934504196159,
-2.06160507429907));
#13426=CARTESIAN_POINT('Ctrl Pts',(93.3118315236789,-0.852570328624139,
-2.03380538754666));
#13427=CARTESIAN_POINT('Ctrl Pts',(93.3077584587417,-0.920709746421028,
-2.00247585824282));
#13428=CARTESIAN_POINT('Ctrl Pts',(93.3036913779354,-0.988749054054269,
-1.97119235815976));
#13429=CARTESIAN_POINT('Ctrl Pts',(93.2996242971292,-1.05529588980259,-1.93638950971336));
#13430=CARTESIAN_POINT('Ctrl Pts',(93.2955572163229,-1.11996415941918,-1.89823504382795));
#13431=CARTESIAN_POINT('Ctrl Pts',(93.2914948939528,-1.18455676792911,-1.86012521821403));
#13432=CARTESIAN_POINT('Ctrl Pts',(93.2874325715827,-1.24727476787778,-1.81867180739638));
#13433=CARTESIAN_POINT('Ctrl Pts',(93.2833702492127,-1.30775516900774,-1.77408917981412));
#13434=CARTESIAN_POINT('Ctrl Pts',(93.2793105050721,-1.36819718510961,-1.72953484743792));
#13435=CARTESIAN_POINT('Ctrl Pts',(93.2752507609316,-1.42640403714235,-1.68185552191804));
#13436=CARTESIAN_POINT('Ctrl Pts',(93.2711910167911,-1.4820414691536,-1.63130900926497));
#13437=CARTESIAN_POINT('Ctrl Pts',(93.2671325373349,-1.53766156909124,-1.58077824277138));
#13438=CARTESIAN_POINT('Ctrl Pts',(93.2630740578786,-1.59071348504336,-1.52738238336798));
#13439=CARTESIAN_POINT('Ctrl Pts',(93.2590155784223,-1.64089708522505,-1.47141862014178));
#13440=CARTESIAN_POINT('Ctrl Pts',(93.2549570517888,-1.6910812687603,-1.41545420637117));
#13441=CARTESIAN_POINT('Ctrl Pts',(93.2508985251552,-1.73839675289855,-1.35692218617953));
#13442=CARTESIAN_POINT('Ctrl Pts',(93.2468399985216,-1.78258233451936,-1.29615439692172));
#13443=CARTESIAN_POINT('Ctrl Pts',(93.2427773215353,-1.82681310144118,-1.23532446497509));
#13444=CARTESIAN_POINT('Ctrl Pts',(93.238714644549,-1.86790729277984,-1.17225458526842));
#13445=CARTESIAN_POINT('Ctrl Pts',(93.2346519675628,-1.9056463322809,-1.10730666766906));
#13446=CARTESIAN_POINT('Ctrl Pts',(93.2305871685845,-1.94340508340016,-1.04232482688109));
#13447=CARTESIAN_POINT('Ctrl Pts',(93.2265223696063,-1.97780497422523,-0.975463419742705));
#13448=CARTESIAN_POINT('Ctrl Pts',(93.2224575706281,-2.00867407397818,-0.907107746923103));
#13449=CARTESIAN_POINT('Ctrl Pts',(93.2183855103849,-2.03959831759262,-0.838629965075903));
#13450=CARTESIAN_POINT('Ctrl Pts',(93.2143134501417,-2.06697899750677,-0.768653031078391));
#13451=CARTESIAN_POINT('Ctrl Pts',(93.2102413898986,-2.0906930480191,-0.697580517907859));
#13452=CARTESIAN_POINT('Ctrl Pts',(93.2071032391105,-2.10896838331895,-0.642808179115762));
#13453=CARTESIAN_POINT('Ctrl Pts',(93.2039650883223,-2.12506707995825,-0.587385556796277));
#13454=CARTESIAN_POINT('Ctrl Pts',(93.2008269375342,-2.13895357252642,-0.531501283701617));
#13455=CARTESIAN_POINT('Ctrl Pts',(93.1967538726001,-2.15697711242492,-0.458968034511747));
#13456=CARTESIAN_POINT('Ctrl Pts',(93.192680807666,-2.17134175589633,-0.385377086445622));
#13457=CARTESIAN_POINT('Ctrl Pts',(93.1886077427318,-2.18192880331932,-0.311131318329639));
#13458=CARTESIAN_POINT('Ctrl Pts',(93.1845406619286,-2.19250029629402,-0.236994631803124));
#13459=CARTESIAN_POINT('Ctrl Pts',(93.1804735811254,-2.19930514545084,-0.162205504061917));
#13460=CARTESIAN_POINT('Ctrl Pts',(93.1764065003222,-2.20227513387128,-0.0871793251420103));
#13461=CARTESIAN_POINT('Ctrl Pts',(93.1723441779552,-2.20524164744059,-0.0122409259592655));
#13462=CARTESIAN_POINT('Ctrl Pts',(93.1682818555882,-2.20438219561364,0.0629334986872736));
#13463=CARTESIAN_POINT('Ctrl Pts',(93.1642195332212,-2.19968027824874,0.137922708367928));
#13464=CARTESIAN_POINT('Ctrl Pts',(93.1601597890837,-2.19498134504443,0.212864324731502));
#13465=CARTESIAN_POINT('Ctrl Pts',(93.1561000449462,-2.18644481542838,0.287620484077586));
#13466=CARTESIAN_POINT('Ctrl Pts',(93.1520403008087,-2.17410626712244,0.361770561625636));
#13467=CARTESIAN_POINT('Ctrl Pts',(93.1479818213555,-2.16177156249902,0.435897540074029));
#13468=CARTESIAN_POINT('Ctrl Pts',(93.1439233419023,-2.14563726907795,0.509418340912239));
#13469=CARTESIAN_POINT('Ctrl Pts',(93.139864862449,-2.12579055500329,0.581919681965469));
#13470=CARTESIAN_POINT('Ctrl Pts',(93.1358063358184,-2.10594361022266,0.654421865802651));
#13471=CARTESIAN_POINT('Ctrl Pts',(93.1317478091879,-2.08238428689612,0.725904106280534));
#13472=CARTESIAN_POINT('Ctrl Pts',(93.1276892825573,-2.05524996718571,0.795967067398613));
#13473=CARTESIAN_POINT('Ctrl Pts',(93.1236266055739,-2.02808789922857,0.866101676685974));
#13474=CARTESIAN_POINT('Ctrl Pts',(93.1195639285906,-1.99734370711549,0.934813662042519));
#13475=CARTESIAN_POINT('Ctrl Pts',(93.1155012516073,-1.96320314489218,1.00172322119709));
#13476=CARTESIAN_POINT('Ctrl Pts',(93.111436452632,-1.92904475058451,1.06866772813299));
#13477=CARTESIAN_POINT('Ctrl Pts',(93.1073716536567,-1.8914866921888,1.13380752008037));
#13478=CARTESIAN_POINT('Ctrl Pts',(93.1033068546814,-1.85075965706099,1.19678932640439));
#13479=CARTESIAN_POINT('Ctrl Pts',(93.0992347944411,-1.80995986807815,1.2598836420037));
#13480=CARTESIAN_POINT('Ctrl Pts',(93.0951627342008,-1.76598007484198,1.32081188424882));
#13481=CARTESIAN_POINT('Ctrl Pts',(93.0910906739605,-1.71909279857905,1.37925195300701));
#13482=CARTESIAN_POINT('Ctrl Pts',(93.0879525231453,-1.68295891657785,1.42428904445179));
#13483=CARTESIAN_POINT('Ctrl Pts',(93.0848143723301,-1.64509912749844,1.46784902064739));
#13484=CARTESIAN_POINT('Ctrl Pts',(93.081676221515,-1.60565270601093,1.5097997839713));
#13485=CARTESIAN_POINT('Ctrl Pts',(93.0776169975952,-1.55462843500475,1.56406344176426));
#13486=CARTESIAN_POINT('Ctrl Pts',(93.0735577736755,-1.50073622542071,1.61585852701187));
#13487=CARTESIAN_POINT('Ctrl Pts',(93.0694985497557,-1.44424906282091,1.66486054807631));
#13488=CARTESIAN_POINT('Ctrl Pts',(93.0654926831042,-1.38850440685476,1.71321845242416));
#13489=CARTESIAN_POINT('Ctrl Pts',(93.0614868164527,-1.33023296663678,1.75885591939796));
#13490=CARTESIAN_POINT('Ctrl Pts',(93.0574809498012,-1.26973675548576,1.80149509346223));
#13491=CARTESIAN_POINT('Ctrl Pts',(93.0534789146843,-1.20929840779994,1.84409348397465));
#13492=CARTESIAN_POINT('Ctrl Pts',(93.0494768795674,-1.14663990856198,1.88369898483093));
#13493=CARTESIAN_POINT('Ctrl Pts',(93.0454748444505,-1.08209667048888,1.92007364330561));
#13494=CARTESIAN_POINT('Ctrl Pts',(93.0414752540233,-1.01759285940324,1.95642608189721));
#13495=CARTESIAN_POINT('Ctrl Pts',(93.0374756635961,-0.95120702175299,1.9895513517484));
#13496=CARTESIAN_POINT('Ctrl Pts',(93.0334760731688,-0.883302375358345,
2.01925553451917));
#13497=CARTESIAN_POINT('Ctrl Pts',(93.0293743043582,-0.813662954585416,
2.04971857633619));
#13498=CARTESIAN_POINT('Ctrl Pts',(93.0252725355475,-0.742426518699399,
2.07658305520151));
#13499=CARTESIAN_POINT('Ctrl Pts',(93.0211707667368,-0.670008820827188,
2.09969144876426));
#13500=CARTESIAN_POINT('Ctrl Pts',(93.0171702427475,-0.599378624206823,
2.12222945299353));
#13501=CARTESIAN_POINT('Ctrl Pts',(93.0131697187582,-0.527625316494081,
2.14119457669626));
#13502=CARTESIAN_POINT('Ctrl Pts',(93.0091691947689,-0.455149799192628,
2.15649128453952));
#13503=CARTESIAN_POINT('Ctrl Pts',(93.0050168035476,-0.379922978253986,
2.17236868348363));
#13504=CARTESIAN_POINT('Ctrl Pts',(93.0008644123262,-0.30391857829625,2.18429343026794));
#13505=CARTESIAN_POINT('Ctrl Pts',(92.9967120211049,-0.227593599682892,
2.19221740559265));
#13506=CARTESIAN_POINT('Ctrl Pts',(92.9925596298835,-0.151268621069534,
2.20014138091737));
#13507=CARTESIAN_POINT('Ctrl Pts',(92.9884072386622,-0.0746236549780797,
2.20406460181512));
#13508=CARTESIAN_POINT('Ctrl Pts',(92.9842548474409,0.00188421767977065,
2.20399919458328));
#13509=CARTESIAN_POINT('',(92.2342548473559,-0.00137440680590686,2.20399957146228));
#13510=CARTESIAN_POINT('Ctrl Pts',(92.98425484741,0.00188421824854456,2.20399919458279));
#13511=CARTESIAN_POINT('Ctrl Pts',(92.9781257762528,0.114812449383132,2.2039026512472));
#13512=CARTESIAN_POINT('Ctrl Pts',(92.9719967050956,0.227381640137665,2.19512359098658));
#13513=CARTESIAN_POINT('Ctrl Pts',(92.9658676339383,0.338536671029629,2.1778450179864));
#13514=CARTESIAN_POINT('Ctrl Pts',(92.9647535911242,0.358740623674827,2.17470440016757));
#13515=CARTESIAN_POINT('Ctrl Pts',(92.96363954831,0.378897939605397,2.17128308505399));
#13516=CARTESIAN_POINT('Ctrl Pts',(92.9625255054959,0.399002376888916,2.16758231752268));
#13517=CARTESIAN_POINT('Ctrl Pts',(92.9584524405509,0.472506444865692,2.15405189812562));
#13518=CARTESIAN_POINT('Ctrl Pts',(92.9543793756058,0.545463242913075,2.13675229502994));
#13519=CARTESIAN_POINT('Ctrl Pts',(92.9503063106608,0.61745682495046,2.11574173029746));
#13520=CARTESIAN_POINT('Ctrl Pts',(92.9462392298466,0.689344634301983,2.09476203420356));
#13521=CARTESIAN_POINT('Ctrl Pts',(92.9421721490325,0.76027158276383,2.07008233382741));
#13522=CARTESIAN_POINT('Ctrl Pts',(92.9381050682184,0.829831171461187,2.04181199596617));
#13523=CARTESIAN_POINT('Ctrl Pts',(92.9340427458404,0.899309376266912,2.01357473406407));
#13524=CARTESIAN_POINT('Ctrl Pts',(92.9299804234625,0.967422959632449,1.98175535997734));
#13525=CARTESIAN_POINT('Ctrl Pts',(92.9259181010845,1.0337814460212,1.9465127592344));
#13526=CARTESIAN_POINT('Ctrl Pts',(92.9218583569362,1.10009781674412,1.91129252587319));
#13527=CARTESIAN_POINT('Ctrl Pts',(92.9177986127878,1.16466088030358,1.87265360056057));
#13528=CARTESIAN_POINT('Ctrl Pts',(92.9137388686394,1.22710222281299,1.83080204685472));
#13529=CARTESIAN_POINT('Ctrl Pts',(92.9096803891753,1.28952411370656,1.78896353067036));
#13530=CARTESIAN_POINT('Ctrl Pts',(92.9056219097112,1.34982519949281,1.74391463878128));
#13531=CARTESIAN_POINT('Ctrl Pts',(92.9015634302472,1.40766505356151,1.69590539151854));
#13532=CARTESIAN_POINT('Ctrl Pts',(92.8975049036057,1.46550557998272,1.64789558617803));
#13533=CARTESIAN_POINT('Ctrl Pts',(92.8934463769643,1.52088445163445,1.59692566346434));
#13534=CARTESIAN_POINT('Ctrl Pts',(92.8893878503229,1.57349467541003,1.54328562050461));
#13535=CARTESIAN_POINT('Ctrl Pts',(92.885325173329,1.6261586997389,1.48959072387229));
#13536=CARTESIAN_POINT('Ctrl Pts',(92.8812624963349,1.67604808719716,1.43322059590487));
#13537=CARTESIAN_POINT('Ctrl Pts',(92.8771998193409,1.72289360674796,1.37450122583685));
#13538=CARTESIAN_POINT('Ctrl Pts',(92.873135020355,1.76976359435597,1.31575118583668));
#13539=CARTESIAN_POINT('Ctrl Pts',(92.8690702213691,1.81358626948841,1.25464984855142));
#13540=CARTESIAN_POINT('Ctrl Pts',(92.8650054223832,1.85413511717714,1.19155317432774));
#13541=CARTESIAN_POINT('Ctrl Pts',(92.8609333621325,1.89475640040844,1.12834378563517));
#13542=CARTESIAN_POINT('Ctrl Pts',(92.8568613018818,1.93209193710563,1.06313235531274));
#13543=CARTESIAN_POINT('Ctrl Pts',(92.8527892416311,1.96596087378275,0.996300076661332));
#13544=CARTESIAN_POINT('Ctrl Pts',(92.849651090913,1.99206211527021,0.944795494132873));
#13545=CARTESIAN_POINT('Ctrl Pts',(92.8465129401949,2.01610544935589,0.892328809120288));
#13546=CARTESIAN_POINT('Ctrl Pts',(92.8433747894768,2.03802806340256,0.83908141010489));
#13547=CARTESIAN_POINT('Ctrl Pts',(92.8393017245573,2.06648183705378,0.769970608086717));
#13548=CARTESIAN_POINT('Ctrl Pts',(92.8352286596379,2.0914711115984,0.69927756218022));
#13549=CARTESIAN_POINT('Ctrl Pts',(92.8311555947184,2.1128194542164,0.627383418560555));
#13550=CARTESIAN_POINT('Ctrl Pts',(92.8270885139298,2.13413643193369,0.555594901532919));
#13551=CARTESIAN_POINT('Ctrl Pts',(92.8230214331413,2.15182296336987,0.482609244246773));
#13552=CARTESIAN_POINT('Ctrl Pts',(92.8189543523527,2.16575072124869,0.40882736382337));
#13553=CARTESIAN_POINT('Ctrl Pts',(92.8148920300002,2.17966218381672,0.335131807321105));
#13554=CARTESIAN_POINT('Ctrl Pts',(92.8108297076477,2.18982352197309,0.260642345318643));
#13555=CARTESIAN_POINT('Ctrl Pts',(92.8067673852952,2.19615671042189,0.185773257679682));
#13556=CARTESIAN_POINT('Ctrl Pts',(92.8027076411722,2.20248587939321,0.110951687118969));
#13557=CARTESIAN_POINT('Ctrl Pts',(92.7986478970492,2.20499167980752,0.0357514435901753));
#13558=CARTESIAN_POINT('Ctrl Pts',(92.7945881529262,2.20364769268452,-0.039406173706866));
#13559=CARTESIAN_POINT('Ctrl Pts',(92.7905296734873,2.20230412423795,-0.114540378038851));
#13560=CARTESIAN_POINT('Ctrl Pts',(92.7864711940484,2.19711315790207,-0.18963150543074));
#13561=CARTESIAN_POINT('Ctrl Pts',(92.7824127146095,2.18810048419052,-0.264257963144402));
#13562=CARTESIAN_POINT('Ctrl Pts',(92.7783541879932,2.17908770571187,-0.338885288347263));
#13563=CARTESIAN_POINT('Ctrl Pts',(92.7742956613769,2.16625319067707,-0.413047459345614));
#13564=CARTESIAN_POINT('Ctrl Pts',(92.7702371347605,2.14967434482391,-0.486329323818632));
#13565=CARTESIAN_POINT('Ctrl Pts',(92.7661744577912,2.1330785450194,-0.559686128198569));
#13566=CARTESIAN_POINT('Ctrl Pts',(92.7621117808218,2.11273087359491,-0.632160361630832));
#13567=CARTESIAN_POINT('Ctrl Pts',(92.7580491038525,2.08875944771065,-0.703349109332978));
#13568=CARTESIAN_POINT('Ctrl Pts',(92.753984304891,2.06477550122077,-0.774575039897725));
#13569=CARTESIAN_POINT('Ctrl Pts',(92.7499195059296,2.03716420656243,-0.844513703133851));
#13570=CARTESIAN_POINT('Ctrl Pts',(92.7458547069682,2.00610201588495,-0.912781847903619));
#13571=CARTESIAN_POINT('Ctrl Pts',(92.7417826467414,1.97498433640915,-0.981171945350702));
#13572=CARTESIAN_POINT('Ctrl Pts',(92.7377105865146,1.94040366765108,-1.047885139144));
#13573=CARTESIAN_POINT('Ctrl Pts',(92.7336385262877,1.90258241024026,-1.11256288462467));
#13574=CARTESIAN_POINT('Ctrl Pts',(92.7305003753443,1.87343529354423,-1.16240707078391));
#13575=CARTESIAN_POINT('Ctrl Pts',(92.727362224401,1.84236451852845,-1.21104288439625));
#13576=CARTESIAN_POINT('Ctrl Pts',(92.7242240734576,1.8094885080123,-1.25831925176857));
#13577=CARTESIAN_POINT('Ctrl Pts',(92.7201510085218,1.76681811768437,-1.31968013520277));
#13578=CARTESIAN_POINT('Ctrl Pts',(92.716077943586,1.72094072377547,-1.37898641940612));
#13579=CARTESIAN_POINT('Ctrl Pts',(92.7120048786501,1.67208108251626,-1.43588330079128));
#13580=CARTESIAN_POINT('Ctrl Pts',(92.7079377978454,1.62329322565133,-1.49269658950033));
#13581=CARTESIAN_POINT('Ctrl Pts',(92.7038707170407,1.57153212899213,-1.54710714428562));
#13582=CARTESIAN_POINT('Ctrl Pts',(92.6998036362361,1.51706523070615,-1.5987898816863));
#13583=CARTESIAN_POINT('Ctrl Pts',(92.6957413138678,1.4626620580471,-1.65041215089538));
#13584=CARTESIAN_POINT('Ctrl Pts',(92.6916789914996,1.405559718007,-1.69931261653392));
#13585=CARTESIAN_POINT('Ctrl Pts',(92.6876166691313,1.34606413470656,-1.7452012334561));
#13586=CARTESIAN_POINT('Ctrl Pts',(92.6835569249928,1.28660631140329,-1.79106072629965));
#13587=CARTESIAN_POINT('Ctrl Pts',(92.6794971808543,1.22475863607776,-1.83391187278125));
#13588=CARTESIAN_POINT('Ctrl Pts',(92.6754374367157,1.16086089392329,-1.87350419934401));
#13589=CARTESIAN_POINT('Ctrl Pts',(92.6713789572616,1.0969830570819,-1.91308419217431));
#13590=CARTESIAN_POINT('Ctrl Pts',(92.6673204778075,1.03105682698992,-1.94940712936845));
#13591=CARTESIAN_POINT('Ctrl Pts',(92.6632619983534,0.963450469551541,-1.98226617605228));
#13592=CARTESIAN_POINT('Ctrl Pts',(92.6592034717221,0.895843326233218,-2.01512560470116));
#13593=CARTESIAN_POINT('Ctrl Pts',(92.6551449450908,0.826556446999674,-2.04452085578788));
#13594=CARTESIAN_POINT('Ctrl Pts',(92.6510864184595,0.755980704991898,-2.07029205033492));
#13595=CARTESIAN_POINT('Ctrl Pts',(92.6470237414757,0.685332790436652,-2.09608959916048));
#13596=CARTESIAN_POINT('Ctrl Pts',(92.6429610644919,0.613393830580244,-2.11825552653667));
#13597=CARTESIAN_POINT('Ctrl Pts',(92.6388983875081,0.540571889473374,-2.13667920669229));
#13598=CARTESIAN_POINT('Ctrl Pts',(92.6348335885325,0.467711912469498,-2.15511250978833));
#13599=CARTESIAN_POINT('Ctrl Pts',(92.630768789557,0.393968504493352,-2.16979957986629));
#13600=CARTESIAN_POINT('Ctrl Pts',(92.6267039905813,0.31975939130576,-2.18068107059968));
#13601=CARTESIAN_POINT('Ctrl Pts',(92.622631930341,0.245417712640053,-2.19158199978153));
#13602=CARTESIAN_POINT('Ctrl Pts',(92.6185598701006,0.170609143097865,-2.19866372567662));
#13603=CARTESIAN_POINT('Ctrl Pts',(92.6144878098602,0.0957555386176693,
-2.20191890786742));
#13604=CARTESIAN_POINT('Ctrl Pts',(92.611349659053,0.0380692851103723,-2.20442752807849));
#13605=CARTESIAN_POINT('Ctrl Pts',(92.6082115082458,-0.0196436158345241,
-2.20466460375587));
#13606=CARTESIAN_POINT('Ctrl Pts',(92.6050733574385,-0.0771920237636312,
-2.20264781376126));
#13607=CARTESIAN_POINT('Ctrl Pts',(92.6010002924366,-0.151885185644805,
-2.20003018406536));
#13608=CARTESIAN_POINT('Ctrl Pts',(92.5969272274347,-0.226589089110338,
-2.19360386226274));
#13609=CARTESIAN_POINT('Ctrl Pts',(92.5928541624328,-0.300883746248021,
-2.18336551480593));
#13610=CARTESIAN_POINT('Ctrl Pts',(92.5887870815615,-0.375069249975267,
-2.17314220948788));
#13611=CARTESIAN_POINT('Ctrl Pts',(92.5847200006903,-0.448846232063083,
-2.15911806265758));
#13612=CARTESIAN_POINT('Ctrl Pts',(92.580652919819,-0.52179655824522,-2.14134171766289));
#13613=CARTESIAN_POINT('Ctrl Pts',(92.5765905973839,-0.594661533415905,
-2.12358617077979));
#13614=CARTESIAN_POINT('Ctrl Pts',(92.5725282749488,-0.666701312686266,
-2.10208726018484));
#13615=CARTESIAN_POINT('Ctrl Pts',(92.5684659525136,-0.737506358812478,
-2.07694496092486));
#13616=CARTESIAN_POINT('Ctrl Pts',(92.564406208308,-0.808266467180875,-2.05181861869925));
#13617=CARTESIAN_POINT('Ctrl Pts',(92.5603464641024,-0.877792948671281,
-2.02305363577183));
#13618=CARTESIAN_POINT('Ctrl Pts',(92.5562867198968,-0.94569117910778,-1.99079988792388));
#13619=CARTESIAN_POINT('Ctrl Pts',(92.5522282403755,-1.01356825800776,-1.95855618770635));
#13620=CARTESIAN_POINT('Ctrl Pts',(92.5481697608542,-1.07981766194409,-1.92282608512564));
#13621=CARTESIAN_POINT('Ctrl Pts',(92.544111281333,-1.14406601336773,-1.88380703816948));
#13622=CARTESIAN_POINT('Ctrl Pts',(92.5400527546345,-1.20831511163644,-1.84478753764241));
#13623=CARTESIAN_POINT('Ctrl Pts',(92.535994227936,-1.27056270404162,-1.80247926620495));
#13624=CARTESIAN_POINT('Ctrl Pts',(92.5319357012376,-1.33046263012875,-1.75712412476492));
#13625=CARTESIAN_POINT('Ctrl Pts',(92.5278730241872,-1.39042381139436,-1.71172260201083));
#13626=CARTESIAN_POINT('Ctrl Pts',(92.5238103471367,-1.44803215061752,-1.66326827603025));
#13627=CARTESIAN_POINT('Ctrl Pts',(92.5197476700863,-1.50297356999078,-1.61204418298916));
#13628=CARTESIAN_POINT('Ctrl Pts',(92.5156828710442,-1.55794368601694,-1.56079333490542));
#13629=CARTESIAN_POINT('Ctrl Pts',(92.5116180720021,-1.61024377582217,-1.50677018218588));
#13630=CARTESIAN_POINT('Ctrl Pts',(92.50755327296,-1.65959762676236,-1.45029366586383));
#13631=CARTESIAN_POINT('Ctrl Pts',(92.5034812126542,-1.70903964228944,-1.39371626118888));
#13632=CARTESIAN_POINT('Ctrl Pts',(92.4994091523483,-1.75552461052594,-1.33467711463645));
#13633=CARTESIAN_POINT('Ctrl Pts',(92.4953370920425,-1.7988177916779,-1.27352681649938));
#13634=CARTESIAN_POINT('Ctrl Pts',(92.4921989418348,-1.83218186176058,-1.22640108495611));
#13635=CARTESIAN_POINT('Ctrl Pts',(92.4890607916271,-1.86365115066336,-1.17802218742702));
#13636=CARTESIAN_POINT('Ctrl Pts',(92.4859226414194,-1.89313695359527,-1.12856035502406));
#13637=CARTESIAN_POINT('Ctrl Pts',(92.4818495766249,-1.93140713759191,-1.06436290273681));
#13638=CARTESIAN_POINT('Ctrl Pts',(92.4777765118305,-1.96648195830376,-0.998092794767605));
#13639=CARTESIAN_POINT('Ctrl Pts',(92.473703447036,-1.9981310558318,-0.930101222298135));
#13640=CARTESIAN_POINT('Ctrl Pts',(92.4696363663724,-2.02973365462996,-0.862209542780111));
#13641=CARTESIAN_POINT('Ctrl Pts',(92.4655692857087,-2.05792032310153,-0.792601849463247));
#13642=CARTESIAN_POINT('Ctrl Pts',(92.4615022050451,-2.08250539196889,-0.721655937701978));
#13643=CARTESIAN_POINT('Ctrl Pts',(92.4574398828168,-2.10706169660204,-0.650793031802234));
#13644=CARTESIAN_POINT('Ctrl Pts',(92.4533775605885,-2.12802461799624,-0.578595467019371));
#13645=CARTESIAN_POINT('Ctrl Pts',(92.4493152383602,-2.14525628891183,-0.505461625530791));
#13646=CARTESIAN_POINT('Ctrl Pts',(92.4452554943608,-2.16247702342434,-0.432374199806173));
#13647=CARTESIAN_POINT('Ctrl Pts',(92.4411957503615,-2.17597109749026,-0.358352140109323));
#13648=CARTESIAN_POINT('Ctrl Pts',(92.4371360063622,-2.18565066535416,-0.28380833151428));
#13649=CARTESIAN_POINT('Ctrl Pts',(92.4330775270464,-2.19532721785809,-0.20928774466007));
#13650=CARTESIAN_POINT('Ctrl Pts',(92.4290190477305,-2.20119156201161,-0.134246204789088));
#13651=CARTESIAN_POINT('Ctrl Pts',(92.4249605684147,-2.20320735648669,-0.0591045203256604));
#13652=CARTESIAN_POINT('Ctrl Pts',(92.4209020419205,-2.20522317439463,0.0160380376317814));
#13653=CARTESIAN_POINT('Ctrl Pts',(92.4168435154264,-2.20339034278361,0.0912802651559923));
#13654=CARTESIAN_POINT('Ctrl Pts',(92.4127849889322,-2.19772462112312,0.166200149546355));
#13655=CARTESIAN_POINT('Ctrl Pts',(92.4087223120829,-2.19205310554775,0.241196648966532));
#13656=CARTESIAN_POINT('Ctrl Pts',(92.4046596352336,-2.18254090876318,0.315869669828599));
#13657=CARTESIAN_POINT('Ctrl Pts',(92.4005969583843,-2.16925574722204,0.389801876783747));
#13658=CARTESIAN_POINT('Ctrl Pts',(92.3965321595419,-2.15596364665474,0.46377269956734));
#13659=CARTESIAN_POINT('Ctrl Pts',(92.3924673606996,-2.13889476541545,0.537001472467057));
#13660=CARTESIAN_POINT('Ctrl Pts',(92.3884025618572,-2.11816751391238,0.609083231591761));
#13661=CARTESIAN_POINT('Ctrl Pts',(92.3843305017464,-2.09740323569742,0.681293756005356));
#13662=CARTESIAN_POINT('Ctrl Pts',(92.3802584416357,-2.0729676890925,0.752352721743964));
#13663=CARTESIAN_POINT('Ctrl Pts',(92.3761863815249,-2.04502835636642,0.82187287438949));
#13664=CARTESIAN_POINT('Ctrl Pts',(92.3730482294833,-2.02349677980574,0.87544890298952));
#13665=CARTESIAN_POINT('Ctrl Pts',(92.3699100774418,-1.99988529071204,0.928111369000052));
#13666=CARTESIAN_POINT('Ctrl Pts',(92.3667719254002,-1.97428890545549,0.979693481551935));
#13667=CARTESIAN_POINT('Ctrl Pts',(92.3626988604202,-1.94106688847823,1.04664284966569));
#13668=CARTESIAN_POINT('Ctrl Pts',(92.3586257954403,-1.90437150272862,1.11202954067353));
#13669=CARTESIAN_POINT('Ctrl Pts',(92.3545527304603,-1.86437310865938,1.17546965580051));
#13670=CARTESIAN_POINT('Ctrl Pts',(92.3504856496126,-1.82443348008519,1.23881656494114));
#13671=CARTESIAN_POINT('Ctrl Pts',(92.3464185687648,-1.78120073044798,1.30022217574047));
#13672=CARTESIAN_POINT('Ctrl Pts',(92.3423514879171,-1.73489179514915,1.35932573694614));
#13673=CARTESIAN_POINT('Ctrl Pts',(92.3382891655078,-1.68863704077807,1.41836014765723));
#13674=CARTESIAN_POINT('Ctrl Pts',(92.3342268430984,-1.63931354433605,1.47509748594237));
#13675=CARTESIAN_POINT('Ctrl Pts',(92.330164520689,-1.58718144445485,1.52920602352274));
#13676=CARTESIAN_POINT('Ctrl Pts',(92.3261047765105,-1.53508243121155,1.58328022008108));
#13677=CARTESIAN_POINT('Ctrl Pts',(92.3220450323321,-1.48017868221333,1.6347285837659));
#13678=CARTESIAN_POINT('Ctrl Pts',(92.3179852881536,-1.42276962835954,1.68325357109904));
#13679=CARTESIAN_POINT('Ctrl Pts',(92.3139268086607,-1.36537845849114,1.73176344199833));
#13680=CARTESIAN_POINT('Ctrl Pts',(92.3098683291679,-1.30548389772671,1.77735143665518));
#13681=CARTESIAN_POINT('Ctrl Pts',(92.3058098496751,-1.24341994265218,1.81975900773011));
#13682=CARTESIAN_POINT('Ctrl Pts',(92.3017513230063,-1.18135526614401,1.86216707175215));
#13683=CARTESIAN_POINT('Ctrl Pts',(92.2976927963376,-1.11712154048893,1.90139437090195));
#13684=CARTESIAN_POINT('Ctrl Pts',(92.2936342696688,-1.05108200374273,1.93722549575628));
#13685=CARTESIAN_POINT('Ctrl Pts',(92.2895715926498,-0.984974933324328,
1.97309326240975));
#13686=CARTESIAN_POINT('Ctrl Pts',(92.2855089156307,-0.917058784726257,
2.00555769115483));
#13687=CARTESIAN_POINT('Ctrl Pts',(92.2814462386117,-0.84772101607827,2.03444957639634));
#13688=CARTESIAN_POINT('Ctrl Pts',(92.277381439602,-0.77834703138449,2.0633565522567));
#13689=CARTESIAN_POINT('Ctrl Pts',(92.2733166405923,-0.707550397932581,
2.0886871076851));
#13690=CARTESIAN_POINT('Ctrl Pts',(92.2692518415826,-0.635735642741988,
2.11032134817128));
#13691=CARTESIAN_POINT('Ctrl Pts',(92.2651797813105,-0.5637925993416,2.13199423556191));
#13692=CARTESIAN_POINT('Ctrl Pts',(92.2611077210383,-0.490828265697908,
2.14995750469995));
#13693=CARTESIAN_POINT('Ctrl Pts',(92.2570356607661,-0.417258872264442,
2.16414210104526));
#13694=CARTESIAN_POINT('Ctrl Pts',(92.2538975103044,-0.360562308231048,
2.17507352017824));
#13695=CARTESIAN_POINT('Ctrl Pts',(92.2507593598427,-0.303506649324913,
2.18376180015199));
#13696=CARTESIAN_POINT('Ctrl Pts',(92.247621209381,-0.246283563827301,2.19019643095968));
#13697=CARTESIAN_POINT('Ctrl Pts',(92.2431657553906,-0.165039905266901,
2.19933213106666));
#13698=CARTESIAN_POINT('Ctrl Pts',(92.2387103014003,-0.0832786634272042,
2.20394849620317));
#13699=CARTESIAN_POINT('Ctrl Pts',(92.23425484741,-0.00137440780056379,
2.20399957146166));
#13700=CARTESIAN_POINT('',(91.4842548474582,-0.0010753174540008,2.20399973767974));
#13701=CARTESIAN_POINT('Ctrl Pts',(92.2342548473559,-0.0013744068059098,
2.20399957146228));
#13702=CARTESIAN_POINT('Ctrl Pts',(92.2302387400664,0.0724533734342382,
2.20404561022061));
#13703=CARTESIAN_POINT('Ctrl Pts',(92.2262226327769,0.146428553931805,2.20037789196652));
#13704=CARTESIAN_POINT('Ctrl Pts',(92.2222065254874,0.220140399541928,2.19297838669001));
#13705=CARTESIAN_POINT('Ctrl Pts',(92.2181961246188,0.293747509200828,2.18558939524906));
#13706=CARTESIAN_POINT('Ctrl Pts',(92.2141857237502,0.367091541643953,2.17447919365826));
#13707=CARTESIAN_POINT('Ctrl Pts',(92.2101753228816,0.439762030251839,2.1596817721018));
#13708=CARTESIAN_POINT('Ctrl Pts',(92.2061680589867,0.512375675311427,2.14489592522941));
#13709=CARTESIAN_POINT('Ctrl Pts',(92.2021607950919,0.584316341462203,2.12642867372763));
#13710=CARTESIAN_POINT('Ctrl Pts',(92.1981535311971,0.655180387247884,2.10436561941259));
#13711=CARTESIAN_POINT('Ctrl Pts',(92.1941480252822,0.726013345094562,2.08231224412277));
#13712=CARTESIAN_POINT('Ctrl Pts',(92.1901425193674,0.795770150846152,2.05666634077465));
#13713=CARTESIAN_POINT('Ctrl Pts',(92.1861370134526,0.864060794999802,2.02756379493823));
#13714=CARTESIAN_POINT('Ctrl Pts',(92.1821318889681,0.932344936073281,1.99846402043588));
#13715=CARTESIAN_POINT('Ctrl Pts',(92.1781267644837,0.999162741319519,1.96590845093099));
#13716=CARTESIAN_POINT('Ctrl Pts',(92.1741216399992,1.064144396598,1.93008100948874));
#13717=CARTESIAN_POINT('Ctrl Pts',(92.1701128062925,1.12918623262785,1.89422038756907));
#13718=CARTESIAN_POINT('Ctrl Pts',(92.1661039725858,1.19238809133431,1.85508207992179));
#13719=CARTESIAN_POINT('Ctrl Pts',(92.1620951388791,1.2534058599113,1.81289540523992));
#13720=CARTESIAN_POINT('Ctrl Pts',(92.1580844473776,1.31445190566342,1.77068918018746));
#13721=CARTESIAN_POINT('Ctrl Pts',(92.1540737558761,1.37331145722272,1.72543207662454));
#13722=CARTESIAN_POINT('Ctrl Pts',(92.1500630643746,1.42967270748152,1.67739439294475));
#13723=CARTESIAN_POINT('Ctrl Pts',(92.1460452816161,1.48613360941294,1.62927177439382));
#13724=CARTESIAN_POINT('Ctrl Pts',(92.1420274988575,1.54008703202777,1.57835909641725));
#13725=CARTESIAN_POINT('Ctrl Pts',(92.1380097160989,1.59125779570186,1.52496381190442));
#13726=CARTESIAN_POINT('Ctrl Pts',(92.1348299751866,1.63175519950507,1.48270588486085));
#13727=CARTESIAN_POINT('Ctrl Pts',(92.1316502342742,1.670510419511,1.43889377606131));
#13728=CARTESIAN_POINT('Ctrl Pts',(92.1284704933619,1.70740591897501,1.3936933048017));
#13729=CARTESIAN_POINT('Ctrl Pts',(92.124397429607,1.75466691467617,1.33579412173266));
#13730=CARTESIAN_POINT('Ctrl Pts',(92.120324365852,1.79907061672403,1.27537658465011));
#13731=CARTESIAN_POINT('Ctrl Pts',(92.1162513020971,1.84033770764652,1.212754353451));
#13732=CARTESIAN_POINT('Ctrl Pts',(92.112184222473,1.8815441691054,1.15022412661185));
#13733=CARTESIAN_POINT('Ctrl Pts',(92.1081171428489,1.91962290824784,1.08549603201815));
#13734=CARTESIAN_POINT('Ctrl Pts',(92.1040500632247,1.95433491919863,1.01891659305406));
#13735=CARTESIAN_POINT('Ctrl Pts',(92.0999877420311,1.98900631754633,0.952415051170976));
#13736=CARTESIAN_POINT('Ctrl Pts',(92.0959254208374,2.02031859402991,0.884066889609817));
#13737=CARTESIAN_POINT('Ctrl Pts',(92.0918630996438,2.04807701364881,0.814245998555335));
#13738=CARTESIAN_POINT('Ctrl Pts',(92.0878033566756,2.07581781588542,0.744469420590216));
#13739=CARTESIAN_POINT('Ctrl Pts',(92.0837436137075,2.10000906114561,0.673222410490049));
#13740=CARTESIAN_POINT('Ctrl Pts',(92.0796838707393,2.12050337198444,0.600900532037216));
#13741=CARTESIAN_POINT('Ctrl Pts',(92.0756253924497,2.14099129849895,0.528601183072256));
#13742=CARTESIAN_POINT('Ctrl Pts',(92.0715669141601,2.15778444706843,0.455228089637544));
#13743=CARTESIAN_POINT('Ctrl Pts',(92.0675084358706,2.17078522852257,0.381192197753571));
#13744=CARTESIAN_POINT('Ctrl Pts',(92.0634499103963,2.18378616112626,0.307155445114334));
#13745=CARTESIAN_POINT('Ctrl Pts',(92.0593913849222,2.19299455825756,0.232456349301329));
#13746=CARTESIAN_POINT('Ctrl Pts',(92.0553328594479,2.19836419316657,0.157514679325787));
#13747=CARTESIAN_POINT('Ctrl Pts',(92.0512701836017,2.20373931922807,0.082496371711897));
#13748=CARTESIAN_POINT('Ctrl Pts',(92.0472075077555,2.20526780959875,0.00723547186445174));
#13749=CARTESIAN_POINT('Ctrl Pts',(92.0431448319093,2.2029555192246,-0.0678452674684539));
#13750=CARTESIAN_POINT('Ctrl Pts',(92.0390800340623,2.20064202110406,-0.142965222677246));
#13751=CARTESIAN_POINT('Ctrl Pts',(92.0350152362152,2.19448378642386,-0.217904353679332));
#13752=CARTESIAN_POINT('Ctrl Pts',(92.0309504383682,2.18453862945074,-0.292244720119107));
#13753=CARTESIAN_POINT('Ctrl Pts',(92.0268783792288,2.17457570660222,-0.366717887045642));
#13754=CARTESIAN_POINT('Ctrl Pts',(92.0228063200895,2.16081243668112,-0.4405896828391));
#13755=CARTESIAN_POINT('Ctrl Pts',(92.0187342609501,2.14335777058606,-0.513452497577281));
#13756=CARTESIAN_POINT('Ctrl Pts',(92.0155960997477,2.12990620859569,-0.569604741562107));
#13757=CARTESIAN_POINT('Ctrl Pts',(92.0124579385452,2.11426333756261,-0.625157938330927));
#13758=CARTESIAN_POINT('Ctrl Pts',(92.0093197773427,2.09649871821207,-0.67993317652188));
#13759=CARTESIAN_POINT('Ctrl Pts',(92.0052467117079,2.07344175716888,-0.751026764748001));
#13760=CARTESIAN_POINT('Ctrl Pts',(92.001173646073,2.04671999095601,-0.821083308681164));
#13761=CARTESIAN_POINT('Ctrl Pts',(91.9971005804382,2.01644570916557,-0.889698095978488));
#13762=CARTESIAN_POINT('Ctrl Pts',(91.993033498944,1.98621590629478,-0.958212074555331));
#13763=CARTESIAN_POINT('Ctrl Pts',(91.9889664174498,1.95244414152328,-1.02528806883605));
#13764=CARTESIAN_POINT('Ctrl Pts',(91.9848993359555,1.91529216765947,-1.0905374420451));
#13765=CARTESIAN_POINT('Ctrl Pts',(91.980837012915,1.8781836613162,-1.15571047399486));
#13766=CARTESIAN_POINT('Ctrl Pts',(91.9767746898745,1.83770303826206,-1.21906071803572));
#13767=CARTESIAN_POINT('Ctrl Pts',(91.972712366834,1.79405903980528,-1.2802219189238));
#13768=CARTESIAN_POINT('Ctrl Pts',(91.9686526220341,1.75044274094981,-1.34134430254171));
#13769=CARTESIAN_POINT('Ctrl Pts',(91.9645928772342,1.70366732739993,-1.40028001230021));
#13770=CARTESIAN_POINT('Ctrl Pts',(91.9605331324343,1.65398541629023,-1.45669085350984));
#13771=CARTESIAN_POINT('Ctrl Pts',(91.9564746523305,1.60431898214355,-1.51308412155283));
#13772=CARTESIAN_POINT('Ctrl Pts',(91.9524161722267,1.55174816350242,-1.56695372463285));
#13773=CARTESIAN_POINT('Ctrl Pts',(91.948357692123,1.49656548249368,-1.61799498040274));
#13774=CARTESIAN_POINT('Ctrl Pts',(91.9442991648546,1.441382160193,-1.66903682933602));
#13775=CARTESIAN_POINT('Ctrl Pts',(91.9402406375861,1.38358726698711,-1.71724994280651));
#13776=CARTESIAN_POINT('Ctrl Pts',(91.9361821103177,1.32350856989508,-1.76236802780074));
#13777=CARTESIAN_POINT('Ctrl Pts',(91.9321194327205,1.26336843516074,-1.80753225142484));
#13778=CARTESIAN_POINT('Ctrl Pts',(91.9280567551233,1.20094021539189,-1.8495948388225));
#13779=CARTESIAN_POINT('Ctrl Pts',(91.9239940775261,1.13658240435961,-1.8883316546889));
#13780=CARTESIAN_POINT('Ctrl Pts',(91.9199292779492,1.07219097855911,-1.92708870320564));
#13781=CARTESIAN_POINT('Ctrl Pts',(91.9158644783724,1.00586837600202,-1.96251629578272));
#13782=CARTESIAN_POINT('Ctrl Pts',(91.9117996787955,0.937997198317188,-1.99443657606581));
#13783=CARTESIAN_POINT('Ctrl Pts',(91.9077276179805,0.870004777560957,-2.02641387779678));
#13784=CARTESIAN_POINT('Ctrl Pts',(91.9036555571654,0.800458698702858,-2.0548711715784));
#13785=CARTESIAN_POINT('Ctrl Pts',(91.8995834963504,0.729760587596923,-2.07967917833261));
#13786=CARTESIAN_POINT('Ctrl Pts',(91.8964453513415,0.675276891359718,-2.09879753783477));
#13787=CARTESIAN_POINT('Ctrl Pts',(91.8933072063326,0.620109401788552,-2.1157495609114));
#13788=CARTESIAN_POINT('Ctrl Pts',(91.8901690613237,0.564446179252859,-2.13049677557298));
#13789=CARTESIAN_POINT('Ctrl Pts',(91.8860959932116,0.492199646322581,-2.14963751304994));
#13790=CARTESIAN_POINT('Ctrl Pts',(91.8820229250996,0.418839076505349,-2.16513610574375));
#13791=CARTESIAN_POINT('Ctrl Pts',(91.8779498569875,0.344765469576315,-2.17686765123372));
#13792=CARTESIAN_POINT('Ctrl Pts',(91.8738827729859,0.270800690841802,-2.18858196085565));
#13793=CARTESIAN_POINT('Ctrl Pts',(91.8698156889843,0.196125422550429,-2.19654013746261));
#13794=CARTESIAN_POINT('Ctrl Pts',(91.8657486049827,0.121153953181855,-2.20066756227023));
#13795=CARTESIAN_POINT('Ctrl Pts',(91.8616862794022,0.0462701991927912,
-2.20479015805908));
#13796=CARTESIAN_POINT('Ctrl Pts',(91.8576239538217,-0.0289085930146785,
-2.20509088047959));
#13797=CARTESIAN_POINT('Ctrl Pts',(91.8535616282411,-0.103961487225625,
-2.20154673109018));
#13798=CARTESIAN_POINT('Ctrl Pts',(91.8495018808824,-0.178966747880666,
-2.19800483105357));
#13799=CARTESIAN_POINT('Ctrl Pts',(91.8454421335237,-0.253845793378832,
-2.19062292400726));
#13800=CARTESIAN_POINT('Ctrl Pts',(91.8413823861651,-0.328177499460303,
-2.17943009267285));
#13801=CARTESIAN_POINT('Ctrl Pts',(91.8373239034875,-0.402486049936229,
-2.168240748098));
#13802=CARTESIAN_POINT('Ctrl Pts',(91.83326542081,-0.47624712769799,-2.15324290735523));
#13803=CARTESIAN_POINT('Ctrl Pts',(91.8292069381325,-0.54904615410687,-2.13451735075179));
#13804=CARTESIAN_POINT('Ctrl Pts',(91.8251484082791,-0.621846026731769,
-2.11579157648245));
#13805=CARTESIAN_POINT('Ctrl Pts',(91.8210898784258,-0.693683363838802,
-2.09333812099535));
#13806=CARTESIAN_POINT('Ctrl Pts',(91.8170313485725,-0.764156756421241,
-2.06728818784798));
#13807=CARTESIAN_POINT('Ctrl Pts',(91.8129686683913,-0.834702216401371,
-2.04121161555605));
#13808=CARTESIAN_POINT('Ctrl Pts',(91.8089059882101,-0.903880497692544,
-2.01153138710734));
#13809=CARTESIAN_POINT('Ctrl Pts',(91.8048433080289,-0.971308976230853,
-1.97842737362112));
#13810=CARTESIAN_POINT('Ctrl Pts',(91.8007785058645,-1.03877267341609,-1.94530606953918));
#13811=CARTESIAN_POINT('Ctrl Pts',(91.7967137037001,-1.1044843301727,-1.9087576515262));
#13812=CARTESIAN_POINT('Ctrl Pts',(91.7926489015357,-1.16808715750088,-1.86900732809733));
#13813=CARTESIAN_POINT('Ctrl Pts',(91.788576838157,-1.23180360259935,-1.82918599614092));
#13814=CARTESIAN_POINT('Ctrl Pts',(91.7845047747783,-1.2934033017218,-1.78615160782476));
#13815=CARTESIAN_POINT('Ctrl Pts',(91.7804327113996,-1.35255998707582,-1.74017168157669));
#13816=CARTESIAN_POINT('Ctrl Pts',(91.7772945893679,-1.3981488889097,-1.70473740510383));
#13817=CARTESIAN_POINT('Ctrl Pts',(91.7741564673362,-1.44228751156915,-1.66755466486185));
#13818=CARTESIAN_POINT('Ctrl Pts',(91.7710183453045,-1.48484162758654,-1.62876067639975));
#13819=CARTESIAN_POINT('Ctrl Pts',(91.7669452899945,-1.54007379078977,-1.57840888666531));
#13820=CARTESIAN_POINT('Ctrl Pts',(91.7628722346845,-1.59284838009649,-1.52514738068764));
#13821=CARTESIAN_POINT('Ctrl Pts',(91.7587991793745,-1.64284314659156,-1.46924551920268));
#13822=CARTESIAN_POINT('Ctrl Pts',(91.7547321082011,-1.69276446072964,-1.41342578878411));
#13823=CARTESIAN_POINT('Ctrl Pts',(91.7506650370278,-1.73991374504865,-1.35497375761978));
#13824=CARTESIAN_POINT('Ctrl Pts',(91.7465979658544,-1.78400381349604,-1.29419720036461));
#13825=CARTESIAN_POINT('Ctrl Pts',(91.7425356530804,-1.82804229736444,-1.23349175057714));
#13826=CARTESIAN_POINT('Ctrl Pts',(91.7384733403064,-1.86902839750786,-1.17046756256348));
#13827=CARTESIAN_POINT('Ctrl Pts',(91.7344110275324,-1.90671471248638,-1.10546596744901));
#13828=CARTESIAN_POINT('Ctrl Pts',(91.7303512929608,-1.944377109329,-1.04050562648706));
#13829=CARTESIAN_POINT('Ctrl Pts',(91.7262915583892,-1.97874363795094,-0.973570780826892));
#13830=CARTESIAN_POINT('Ctrl Pts',(91.7222318238177,-2.00961056888026,-0.905031138384061));
#13831=CARTESIAN_POINT('Ctrl Pts',(91.7181733538899,-2.0404678844829,-0.8365128466565));
#13832=CARTESIAN_POINT('Ctrl Pts',(91.7141148839622,-2.06782757091763,-0.766391185760943));
#13833=CARTESIAN_POINT('Ctrl Pts',(91.7100564140345,-2.09153289675691,-0.695058372932542));
#13834=CARTESIAN_POINT('Ctrl Pts',(91.7059978968757,-2.11523849847037,-0.623724729958193));
#13835=CARTESIAN_POINT('Ctrl Pts',(91.701939379717,-2.13528950627479,-0.551180360729292));
#13836=CARTESIAN_POINT('Ctrl Pts',(91.6978808625582,-2.15157870476266,-0.477833733857121));
#13837=CARTESIAN_POINT('Ctrl Pts',(91.6938181948983,-2.16788456163447,-0.404412097998338));
#13838=CARTESIAN_POINT('Ctrl Pts',(91.6897555272384,-2.18042082306836,-0.330187033266231));
#13839=CARTESIAN_POINT('Ctrl Pts',(91.6856928595785,-2.18913135652916,-0.255577588729571));
#13840=CARTESIAN_POINT('Ctrl Pts',(91.681628069859,-2.19784643977656,-0.180929173324751));
#13841=CARTESIAN_POINT('Ctrl Pts',(91.6775632801395,-2.20273178458476,-0.105896455191822));
#13842=CARTESIAN_POINT('Ctrl Pts',(91.6734984904201,-2.20378336221302,-0.0309013338396533));
#13843=CARTESIAN_POINT('Ctrl Pts',(91.6694264392199,-2.20483681841586,0.0442277613854869));
#13844=CARTESIAN_POINT('Ctrl Pts',(91.6653543880198,-2.20204284532493,0.119318647833614));
#13845=CARTESIAN_POINT('Ctrl Pts',(91.6612823368197,-2.19544951245386,0.193952154579663));
#13846=CARTESIAN_POINT('Ctrl Pts',(91.658144100975,-2.19036818303649,0.251470475096262));
#13847=CARTESIAN_POINT('Ctrl Pts',(91.6550058651302,-2.18303132525941,0.308717180314805));
#13848=CARTESIAN_POINT('Ctrl Pts',(91.6518676292855,-2.1734815463362,0.365505085786788));
#13849=CARTESIAN_POINT('Ctrl Pts',(91.6477945561724,-2.16108701970002,0.43920932675874));
#13850=CARTESIAN_POINT('Ctrl Pts',(91.6437214830593,-2.14491530015174,0.512424525006328));
#13851=CARTESIAN_POINT('Ctrl Pts',(91.6396484099462,-2.12501818452048,0.584733884307464));
#13852=CARTESIAN_POINT('Ctrl Pts',(91.6355813210328,-2.10515030193009,0.656937005976228));
#13853=CARTESIAN_POINT('Ctrl Pts',(91.6315142321194,-2.08156801578952,0.728236474486894));
#13854=CARTESIAN_POINT('Ctrl Pts',(91.6274471432059,-2.054374407353,0.798224150482185));
#13855=CARTESIAN_POINT('Ctrl Pts',(91.6233848128683,-2.02721261598494,0.868129939489815));
#13856=CARTESIAN_POINT('Ctrl Pts',(91.6193224825306,-1.9964480691207,0.936726542518279));
#13857=CARTESIAN_POINT('Ctrl Pts',(91.615260152193,-1.96223360810615,1.0036210775082));
#13858=CARTESIAN_POINT('Ctrl Pts',(91.611200400174,-1.92804086265294,1.07047315523488));
#13859=CARTESIAN_POINT('Ctrl Pts',(91.607140648155,-1.89040276498942,1.13562488462496));
#13860=CARTESIAN_POINT('Ctrl Pts',(91.603080896136,-1.84951966932641,1.19870471458768));
#13861=CARTESIAN_POINT('Ctrl Pts',(91.5990224089008,-1.80864931046897,1.26176489252755));
#13862=CARTESIAN_POINT('Ctrl Pts',(91.5949639216654,-1.76453622032653,1.32275405221568));
#13863=CARTESIAN_POINT('Ctrl Pts',(91.5909054344301,-1.71742513656064,1.38132794813891));
#13864=CARTESIAN_POINT('Ctrl Pts',(91.5868469001273,-1.67031350643343,1.43990252336113));
#13865=CARTESIAN_POINT('Ctrl Pts',(91.5827883658245,-1.62020411428653,1.49606140827559));
#13866=CARTESIAN_POINT('Ctrl Pts',(91.5787298315217,-1.5673821857963,1.54949316992636));
#13867=CARTESIAN_POINT('Ctrl Pts',(91.5746671470881,-1.514506243246,1.6029795692336));
#13868=CARTESIAN_POINT('Ctrl Pts',(91.5706044626544,-1.45891256173779,1.65373293615841));
#13869=CARTESIAN_POINT('Ctrl Pts',(91.5665417782208,-1.40092293754828,1.70147903985065));
#13870=CARTESIAN_POINT('Ctrl Pts',(91.5624769719064,-1.34290302622578,1.74925008063488));
#13871=CARTESIAN_POINT('Ctrl Pts',(91.5584121655921,-1.28248506425117,1.79401044590272));
#13872=CARTESIAN_POINT('Ctrl Pts',(91.5543473592777,-1.22002147472927,1.83552815320262));
#13873=CARTESIAN_POINT('Ctrl Pts',(91.5502752919629,-1.15744630592912,1.87712002396079));
#13874=CARTESIAN_POINT('Ctrl Pts',(91.5462032246481,-1.09281862200705,1.9154574229452));
#13875=CARTESIAN_POINT('Ctrl Pts',(91.5421311573332,-1.0265167807496,1.95035363430314));
#13876=CARTESIAN_POINT('Ctrl Pts',(91.5389930759776,-0.975422200083803,
1.97724590836889));
#13877=CARTESIAN_POINT('Ctrl Pts',(91.5358549946219,-0.923333918039295,
2.00209545679016));
#13878=CARTESIAN_POINT('Ctrl Pts',(91.5327169132663,-0.870432319660632,
2.0248366790658));
#13879=CARTESIAN_POINT('Ctrl Pts',(91.5282130966559,-0.794507233441178,
2.0574751874461));
#13880=CARTESIAN_POINT('Ctrl Pts',(91.5237092800456,-0.716656622068216,
2.0858771805404));
#13881=CARTESIAN_POINT('Ctrl Pts',(91.5192054634353,-0.637345146763546,
2.10983581444077));
#13882=CARTESIAN_POINT('Ctrl Pts',(91.5147154542498,-0.558276817957318,
2.13372099796189));
#13883=CARTESIAN_POINT('Ctrl Pts',(91.5102254450644,-0.477756831322773,
2.15318986501427));
#13884=CARTESIAN_POINT('Ctrl Pts',(91.505735435879,-0.396268453458691,2.16808378823178));
#13885=CARTESIAN_POINT('Ctrl Pts',(91.5012685484843,-0.315199708861933,
2.1829010135713));
#13886=CARTESIAN_POINT('Ctrl Pts',(91.4968016610897,-0.233172802184434,
2.19319016597525));
#13887=CARTESIAN_POINT('Ctrl Pts',(91.492334773695,-0.150682170051668,2.19884307844569));
#13888=CARTESIAN_POINT('Ctrl Pts',(91.4896414649494,-0.100944462040351,
2.20225150074286));
#13889=CARTESIAN_POINT('Ctrl Pts',(91.4869481562038,-0.0510385083173603,
2.2039753609567));
#13890=CARTESIAN_POINT('Ctrl Pts',(91.4842548474582,-0.0010753174540001,
2.20399973767974));
#13891=CARTESIAN_POINT('',(90.7342548473723,0.00189326485402309,2.2039991868302));
#13892=CARTESIAN_POINT('Ctrl Pts',(91.48425484741,-0.00107531656039788,
2.20399973768018));
#13893=CARTESIAN_POINT('Ctrl Pts',(91.4801345475516,0.0753597852745452,
2.20403702984923));
#13894=CARTESIAN_POINT('Ctrl Pts',(91.4760142476932,0.151787090692672,2.20009380347946));
#13895=CARTESIAN_POINT('Ctrl Pts',(91.4718939478347,0.22777218684923,2.19219885751679));
#13896=CARTESIAN_POINT('Ctrl Pts',(91.4677719624903,0.303788366135591,2.18430068197829));
#13897=CARTESIAN_POINT('Ctrl Pts',(91.4636499771459,0.379361522226958,2.17244762155421));
#13898=CARTESIAN_POINT('Ctrl Pts',(91.4595279918015,0.45406412797954,2.15672014125203));
#13899=CARTESIAN_POINT('Ctrl Pts',(91.4553998074611,0.528879077931765,2.14096900861311));
#13900=CARTESIAN_POINT('Ctrl Pts',(91.4512716231209,0.60282041544042,2.12133191698089));
#13901=CARTESIAN_POINT('Ctrl Pts',(91.4471434387806,0.675472845712013,2.09794004554604));
#13902=CARTESIAN_POINT('Ctrl Pts',(91.4430119747139,0.74818299629565,2.07452958992737));
#13903=CARTESIAN_POINT('Ctrl Pts',(91.4388805106473,0.819601773231825,2.04735857617575));
#13904=CARTESIAN_POINT('Ctrl Pts',(91.4347490465807,0.889333527039305,2.01660652525073));
#13905=CARTESIAN_POINT('Ctrl Pts',(91.4306090428813,0.959209414635745,1.98579091060651));
#13906=CARTESIAN_POINT('Ctrl Pts',(91.4264690391819,1.02739090475845,1.95137967828839));
#13907=CARTESIAN_POINT('Ctrl Pts',(91.4223290354825,1.09350671021836,1.91359846224526));
#13908=CARTESIAN_POINT('Ctrl Pts',(91.419408089404,1.14015418126097,1.88694223127194));
#13909=CARTESIAN_POINT('Ctrl Pts',(91.4164871433255,1.18577393310765,1.85860941038486));
#13910=CARTESIAN_POINT('Ctrl Pts',(91.4135661972471,1.23024510906643,1.82869160101372));
#13911=CARTESIAN_POINT('Ctrl Pts',(91.4094932090485,1.292256036344,1.78697399267035));
#13912=CARTESIAN_POINT('Ctrl Pts',(91.40542022085,1.3522622016404,1.74201815661329));
#13913=CARTESIAN_POINT('Ctrl Pts',(91.4013472326515,1.40990538202678,1.69404333289675));
#13914=CARTESIAN_POINT('Ctrl Pts',(91.3972802286801,1.46746387032373,1.64613899606233));
#13915=CARTESIAN_POINT('Ctrl Pts',(91.3932132247086,1.52266590270625,1.59522478102214));
#13916=CARTESIAN_POINT('Ctrl Pts',(91.3891462207372,1.57518231321275,1.54156306395222));
#13917=CARTESIAN_POINT('Ctrl Pts',(91.3850839749833,1.62763728180575,1.48796412875459));
#13918=CARTESIAN_POINT('Ctrl Pts',(91.3810217292294,1.67741253878216,1.4316244174492));
#13919=CARTESIAN_POINT('Ctrl Pts',(91.3769594834755,1.72421335770118,1.3728453289154));
#13920=CARTESIAN_POINT('Ctrl Pts',(91.3728998157806,1.7709844750023,1.31410354387476));
#13921=CARTESIAN_POINT('Ctrl Pts',(91.3688401480857,1.81478460350243,1.25292582627685));
#13922=CARTESIAN_POINT('Ctrl Pts',(91.3647804803908,1.85535806068537,1.18964804318329));
#13923=CARTESIAN_POINT('Ctrl Pts',(91.3607220771031,1.89591888102782,1.12638996832528));
#13924=CARTESIAN_POINT('Ctrl Pts',(91.3566636738155,1.93325476780625,1.06103352830072));
#13925=CARTESIAN_POINT('Ctrl Pts',(91.3526052705278,1.96715323228298,0.993943741224126));
#13926=CARTESIAN_POINT('Ctrl Pts',(91.3485468196791,2.0010520940205,0.926853167913054));
#13927=CARTESIAN_POINT('Ctrl Pts',(91.3444883688305,2.03151323974132,0.858029634195111));
#13928=CARTESIAN_POINT('Ctrl Pts',(91.3404299179818,2.05837078210288,0.7878614874362));
#13929=CARTESIAN_POINT('Ctrl Pts',(91.3363673156635,2.08525579757623,0.717621564290818));
#13930=CARTESIAN_POINT('Ctrl Pts',(91.3323047133451,2.10852967750412,0.646034728369659));
#13931=CARTESIAN_POINT('Ctrl Pts',(91.3282421110267,2.12807551660858,0.573507275987955));
#13932=CARTESIAN_POINT('Ctrl Pts',(91.3241773862146,2.14763156737461,0.500941931869087));
#13933=CARTESIAN_POINT('Ctrl Pts',(91.3201126614026,2.16345559808519,0.427435459893576));
#13934=CARTESIAN_POINT('Ctrl Pts',(91.3160479365905,2.17548182781943,0.353404607818623));
#13935=CARTESIAN_POINT('Ctrl Pts',(91.3119759488505,2.18752954625082,0.279241476002225));
#13936=CARTESIAN_POINT('Ctrl Pts',(91.3079039611105,2.19576585682346,0.204552567865129));
#13937=CARTESIAN_POINT('Ctrl Pts',(91.3038319733704,2.20017691466317,0.129759562974175));
#13938=CARTESIAN_POINT('Ctrl Pts',(91.3006931426563,2.2035771124813,0.0721064962309344));
#13939=CARTESIAN_POINT('Ctrl Pts',(91.2975543119422,2.20470546515236,0.0143916924216315));
#13940=CARTESIAN_POINT('Ctrl Pts',(91.294415481228,2.20357671439982,-0.0431933299815596));
#13941=CARTESIAN_POINT('Ctrl Pts',(91.2903423321053,2.20211197464282,-0.117919368065657));
#13942=CARTESIAN_POINT('Ctrl Pts',(91.2862691829825,2.19683902233028,-0.192714898337843));
#13943=CARTESIAN_POINT('Ctrl Pts',(91.2821960338598,2.18774804839455,-0.267160020859897));
#13944=CARTESIAN_POINT('Ctrl Pts',(91.2781288693383,2.17867043165546,-0.341495762566669));
#13945=CARTESIAN_POINT('Ctrl Pts',(91.2740617048168,2.16578598833572,-0.415481648720905));
#13946=CARTESIAN_POINT('Ctrl Pts',(91.2699945402953,2.14913690866279,-0.488698831411888));
#13947=CARTESIAN_POINT('Ctrl Pts',(91.2659321352976,2.13250731226656,-0.561830333052806));
#13948=CARTESIAN_POINT('Ctrl Pts',(91.2618697303,2.11212193757829,-0.63419445523976));
#13949=CARTESIAN_POINT('Ctrl Pts',(91.2578073253023,2.08807443297473,-0.705380154496332));
#13950=CARTESIAN_POINT('Ctrl Pts',(91.2537474992385,2.0640421944325,-0.776520662982861));
#13951=CARTESIAN_POINT('Ctrl Pts',(91.2496876731747,2.03635259176569,-0.846483781878596));
#13952=CARTESIAN_POINT('Ctrl Pts',(91.2456278471109,2.00514939821203,-0.914872609082792));
#13953=CARTESIAN_POINT('Ctrl Pts',(91.2415692865451,1.97395593107933,-0.983240118644564));
#13954=CARTESIAN_POINT('Ctrl Pts',(91.2375107259792,1.93925124564859,-1.05003387675144));
#13955=CARTESIAN_POINT('Ctrl Pts',(91.2334521654133,1.90122701960133,-1.11487749099972));
#13956=CARTESIAN_POINT('Ctrl Pts',(91.229393558594,1.86320236021025,-1.1797218442395));
#13957=CARTESIAN_POINT('Ctrl Pts',(91.2253349517747,1.82185832814373,-1.24261559854748));
#13958=CARTESIAN_POINT('Ctrl Pts',(91.2212763449554,1.77743145891488,-1.30320888918842));
#13959=CARTESIAN_POINT('Ctrl Pts',(91.2172135897585,1.73295918015641,-1.3638641133591));
#13960=CARTESIAN_POINT('Ctrl Pts',(91.2131508345617,1.68539805474719,-1.42221379246401));
#13961=CARTESIAN_POINT('Ctrl Pts',(91.2090880793648,1.6350262438774,-1.4779395054711));
#13962=CARTESIAN_POINT('Ctrl Pts',(91.205023203148,1.58462813567742,-1.5336943108902));
#13963=CARTESIAN_POINT('Ctrl Pts',(91.2009583269312,1.53141675808621,-1.58682208457118));
#13964=CARTESIAN_POINT('Ctrl Pts',(91.1968934507144,1.47570675792028,-1.63704171132821));
#13965=CARTESIAN_POINT('Ctrl Pts',(91.1928213156935,1.41989727428702,-1.68735101718385));
#13966=CARTESIAN_POINT('Ctrl Pts',(91.1887491806725,1.36158062687592,-1.73474150156833));
#13967=CARTESIAN_POINT('Ctrl Pts',(91.1846770456516,1.30110374867889,-1.7789730282311));
#13968=CARTESIAN_POINT('Ctrl Pts',(91.1815396188373,1.25450858954928,-1.81305175525604));
#13969=CARTESIAN_POINT('Ctrl Pts',(91.1784021920231,1.20663176737054,-1.84525612230047));
#13970=CARTESIAN_POINT('Ctrl Pts',(91.1752647652088,1.15764200097884,-1.87549486738026));
#13971=CARTESIAN_POINT('Ctrl Pts',(91.1711915775716,1.0940406733218,-1.91475254251144));
#13972=CARTESIAN_POINT('Ctrl Pts',(91.1671183899345,1.0283175516707,-1.95084696681253));
#13973=CARTESIAN_POINT('Ctrl Pts',(91.1630452022973,0.960820261995865,-1.98354239282608));
#13974=CARTESIAN_POINT('Ctrl Pts',(91.1589779973941,0.893422112936246,-2.01618979550913));
#13975=CARTESIAN_POINT('Ctrl Pts',(91.154910792491,0.824255395773518,-2.04544790562825));
#13976=CARTESIAN_POINT('Ctrl Pts',(91.1508435875878,0.753695024608214,-2.07112525209868));
#13977=CARTESIAN_POINT('Ctrl Pts',(91.1467811396405,0.683217180037177,-2.09677256664157));
#13978=CARTESIAN_POINT('Ctrl Pts',(91.1427186916931,0.611349366301141,-2.11884727574468));
#13979=CARTESIAN_POINT('Ctrl Pts',(91.1386562437458,0.53848781731309,-2.13720538802554));
#13980=CARTESIAN_POINT('Ctrl Pts',(91.1345963731848,0.465672494730524,-2.15555185315431));
#13981=CARTESIAN_POINT('Ctrl Pts',(91.1305365026239,0.391865149778248,-2.17018628424562));
#13982=CARTESIAN_POINT('Ctrl Pts',(91.126476632063,0.317477287424272,-2.18101448229252));
#13983=CARTESIAN_POINT('Ctrl Pts',(91.1224180255295,0.243112585488015,-2.19183930901537));
#13984=CARTESIAN_POINT('Ctrl Pts',(91.1183594189959,0.168168197146597,-2.19886018685535));
#13985=CARTESIAN_POINT('Ctrl Pts',(91.1143008124624,0.0930643429279588,
-2.20203429311975));
#13986=CARTESIAN_POINT('Ctrl Pts',(91.1102421582803,0.0179596069796596,
-2.2052084366486));
#13987=CARTESIAN_POINT('Ctrl Pts',(91.1061835040982,-0.0573041214864556,
-2.20453570056347));
#13988=CARTESIAN_POINT('Ctrl Pts',(91.1021248499161,-0.132304615016989,
-2.200025338228));
#13989=CARTESIAN_POINT('Ctrl Pts',(91.0980620455509,-0.207381800418263,
-2.19551036381453));
#13990=CARTESIAN_POINT('Ctrl Pts',(91.0939992411856,-0.282194735740037,
-2.1871499555293));
#13991=CARTESIAN_POINT('Ctrl Pts',(91.0899364368204,-0.356325069411539,
-2.17500538962754));
#13992=CARTESIAN_POINT('Ctrl Pts',(91.0858715103569,-0.430494123099852,
-2.16285448033338));
#13993=CARTESIAN_POINT('Ctrl Pts',(91.0818065838934,-0.50397939811163,-2.14691557859187));
#13994=CARTESIAN_POINT('Ctrl Pts',(91.0777416574299,-0.576374130845831,
-2.12730083939525));
#13995=CARTESIAN_POINT('Ctrl Pts',(91.0736694709889,-0.648898160908092,
-2.10765106818355));
#13996=CARTESIAN_POINT('Ctrl Pts',(91.0695972845479,-0.720327303794025,
-2.08431249480676));
#13997=CARTESIAN_POINT('Ctrl Pts',(91.0655250981069,-0.790271746160557,
-2.0574466134557));
#13998=CARTESIAN_POINT('Ctrl Pts',(91.0623880818012,-0.844153575830507,
-2.0367504324024));
#13999=CARTESIAN_POINT('Ctrl Pts',(91.0592510654954,-0.897154658303896,
-2.01396202043894));
#14000=CARTESIAN_POINT('Ctrl Pts',(91.0561140491897,-0.94910694297007,-1.98917370051135));
#14001=CARTESIAN_POINT('Ctrl Pts',(91.0520415827155,-1.01655126488137,-1.95699356753781));
#14002=CARTESIAN_POINT('Ctrl Pts',(91.0479691162412,-1.08248738225664,-1.92131726115899));
#14003=CARTESIAN_POINT('Ctrl Pts',(91.0438966497669,-1.14652888156507,-1.88230909357023));
#14004=CARTESIAN_POINT('Ctrl Pts',(91.0398301685679,-1.21047625953367,-1.84335825601023));
#14005=CARTESIAN_POINT('Ctrl Pts',(91.0357636873689,-1.27253414325808,-1.80108552571422));
#14006=CARTESIAN_POINT('Ctrl Pts',(91.0316972061699,-1.33233853679501,-1.7557021454025));
#14007=CARTESIAN_POINT('Ctrl Pts',(91.0276354822864,-1.39207296606744,-1.71037185842785));
#14008=CARTESIAN_POINT('Ctrl Pts',(91.0235737584028,-1.44955876432225,-1.66193843870085));
#14009=CARTESIAN_POINT('Ctrl Pts',(91.0195120345193,-1.50446028197339,-1.61065677907012));
#14010=CARTESIAN_POINT('Ctrl Pts',(91.0154528878933,-1.55932696334508,-1.55940765883543));
#14011=CARTESIAN_POINT('Ctrl Pts',(91.0113937412672,-1.61161226990499,-1.50531421019386));
#14012=CARTESIAN_POINT('Ctrl Pts',(91.0073345946412,-1.66101412244257,-1.44867114454811));
#14013=CARTESIAN_POINT('Ctrl Pts',(91.003276710894,-1.7104006051109,-1.39204570165269));
#14014=CARTESIAN_POINT('Ctrl Pts',(90.9992188271467,-1.7569051011597,-1.33287257638486));
#14015=CARTESIAN_POINT('Ctrl Pts',(90.9951609433995,-1.8002639873571,-1.27148164588606));
#14016=CARTESIAN_POINT('Ctrl Pts',(90.9911030098348,-1.84362340585925,-1.21008996170821));
#14017=CARTESIAN_POINT('Ctrl Pts',(90.9870450762701,-1.88383686376207,-1.14648080939786));
#14018=CARTESIAN_POINT('Ctrl Pts',(90.9829871427054,-1.92068341877735,-1.08101397069314));
#14019=CARTESIAN_POINT('Ctrl Pts',(90.9789250506036,-1.95756773384043,-1.0154800421083));
#14020=CARTESIAN_POINT('Ctrl Pts',(90.9748629585018,-1.99107802105361,-0.948085042622554));
#14021=CARTESIAN_POINT('Ctrl Pts',(90.9708008664,-2.02103916263345,-0.87921368455108));
#14022=CARTESIAN_POINT('Ctrl Pts',(90.9667366486916,-2.0510159822424,-0.810306287560541));
#14023=CARTESIAN_POINT('Ctrl Pts',(90.9626724309833,-2.07743978984685,-0.739921441117149));
#14024=CARTESIAN_POINT('Ctrl Pts',(90.958608213275,-2.10018451078152,-0.668461682277608));
#14025=CARTESIAN_POINT('Ctrl Pts',(90.9545367217817,-2.1229699382485,-0.596874030948583));
#14026=CARTESIAN_POINT('Ctrl Pts',(90.9504652302884,-2.14206300549317,-0.524208087245253));
#14027=CARTESIAN_POINT('Ctrl Pts',(90.9463937387951,-2.15738829210057,-0.450878871879563));
#14028=CARTESIAN_POINT('Ctrl Pts',(90.9432502702536,-2.16922045641158,-0.394263726777795));
#14029=CARTESIAN_POINT('Ctrl Pts',(90.9401068017121,-2.17880772658627,-0.337253484604036));
#14030=CARTESIAN_POINT('Ctrl Pts',(90.9369633331706,-2.18613660174063,-0.280040637283147));
#14031=CARTESIAN_POINT('Ctrl Pts',(90.932889462496,-2.1956346734329,-0.205893962093828));
#14032=CARTESIAN_POINT('Ctrl Pts',(90.9288155918213,-2.20137453506395,-0.131120765785595));
#14033=CARTESIAN_POINT('Ctrl Pts',(90.9247417211466,-2.20328501326668,-0.056135107681679));
#14034=CARTESIAN_POINT('Ctrl Pts',(90.9206738376651,-2.20519268372146,0.018740347213517));
#14035=CARTESIAN_POINT('Ctrl Pts',(90.9166059541837,-2.20328213245543,0.0938271708094514));
#14036=CARTESIAN_POINT('Ctrl Pts',(90.9125380707022,-2.19753377957874,0.168704734996868));
#14037=CARTESIAN_POINT('Ctrl Pts',(90.9084749539541,-2.19179216260434,0.243494557884093));
#14038=CARTESIAN_POINT('Ctrl Pts',(90.904411837206,-2.18222171526202,0.318075135074735));
#14039=CARTESIAN_POINT('Ctrl Pts',(90.900348720458,-2.16885490383549,0.392026027335872));
#14040=CARTESIAN_POINT('Ctrl Pts',(90.8962881873953,-2.15549659219831,0.465929895143214));
#14041=CARTESIAN_POINT('Ctrl Pts',(90.8922276543327,-2.13834679166121,0.539204404142618));
#14042=CARTESIAN_POINT('Ctrl Pts',(90.8881671212701,-2.11748962360874,0.611435764336152));
#14043=CARTESIAN_POINT('Ctrl Pts',(90.8841078594163,-2.09663898519549,0.683644511453837));
#14044=CARTESIAN_POINT('Ctrl Pts',(90.8800485975625,-2.07208341602311,0.75481029994527));
#14045=CARTESIAN_POINT('Ctrl Pts',(90.8759893357087,-2.04395742924475,0.824532611504955));
#14046=CARTESIAN_POINT('Ctrl Pts',(90.8719300342768,-2.01583116823547,0.894255602863506));
#14047=CARTESIAN_POINT('Ctrl Pts',(90.8678707328448,-1.98413460070982,0.962534647413805));
#14048=CARTESIAN_POINT('Ctrl Pts',(90.8638114314128,-1.94905050029505,1.02898889561532));
#14049=CARTESIAN_POINT('Ctrl Pts',(90.859747996683,-1.91393067623649,1.09551080945062));
#14050=CARTESIAN_POINT('Ctrl Pts',(90.8556845619531,-1.87541665453586,1.16020379348521));
#14051=CARTESIAN_POINT('Ctrl Pts',(90.8516211272232,-1.83373699234912,1.22271200324951));
#14052=CARTESIAN_POINT('Ctrl Pts',(90.847555578769,-1.79203564916534,1.28525272863988));
#14053=CARTESIAN_POINT('Ctrl Pts',(90.8434900303148,-1.7471656711554,1.34560603313343));
#14054=CARTESIAN_POINT('Ctrl Pts',(90.8394244818606,-1.69939717640751,1.4034476252494));
#14055=CARTESIAN_POINT('Ctrl Pts',(90.835351694127,-1.65154362315281,1.4613922124353));
#14056=CARTESIAN_POINT('Ctrl Pts',(90.8312789063934,-1.6007815667975,1.51681580132527));
#14057=CARTESIAN_POINT('Ctrl Pts',(90.8272061186598,-1.54741907026956,1.56942990317061));
#14058=CARTESIAN_POINT('Ctrl Pts',(90.8240749514903,-1.50639387864707,1.60987972749844));
#14059=CARTESIAN_POINT('Ctrl Pts',(90.8209437843209,-1.46383247197762,1.64866971655217));
#14060=CARTESIAN_POINT('Ctrl Pts',(90.8178126171514,-1.41988740623812,1.68568554410554));
#14061=CARTESIAN_POINT('Ctrl Pts',(90.8137657639652,-1.36309094035839,1.73352636880945));
#14062=CARTESIAN_POINT('Ctrl Pts',(90.8097189107791,-1.30375598984691,1.77859266049886));
#14063=CARTESIAN_POINT('Ctrl Pts',(90.8056720575929,-1.24218642093431,1.82060124564562));
#14064=CARTESIAN_POINT('Ctrl Pts',(90.8016308065827,-1.18070208455728,1.86255167709258));
#14065=CARTESIAN_POINT('Ctrl Pts',(90.7975895555724,-1.1169896612247,1.90145252786528));
#14066=CARTESIAN_POINT('Ctrl Pts',(90.7935483045622,-1.05138688805472,1.93706004337155));
#14067=CARTESIAN_POINT('Ctrl Pts',(90.7895113008791,-0.985853062949274,
1.97263013562332));
#14068=CARTESIAN_POINT('Ctrl Pts',(90.7854742971959,-0.918433253117161,
2.00491353132598));
#14069=CARTESIAN_POINT('Ctrl Pts',(90.7814372935128,-0.849493646490407,
2.03371004437025));
#14070=CARTESIAN_POINT('Ctrl Pts',(90.7774025713876,-0.780593001856861,
2.06249028274165));
#14071=CARTESIAN_POINT('Ctrl Pts',(90.7733678492625,-0.710174707678702,
2.08778735697564));
#14072=CARTESIAN_POINT('Ctrl Pts',(90.7693331271373,-0.638627650683483,
2.10944796659754));
#14073=CARTESIAN_POINT('Ctrl Pts',(90.7652999118247,-0.567107313745175,
2.13110048682001));
#14074=CARTESIAN_POINT('Ctrl Pts',(90.7612666965122,-0.494459514900456,
2.14911910202913));
#14075=CARTESIAN_POINT('Ctrl Pts',(90.7572334811996,-0.421089349198961,
2.1634000462215));
#14076=CARTESIAN_POINT('Ctrl Pts',(90.7531984374294,-0.347685921144087,
2.17768746467774));
#14077=CARTESIAN_POINT('Ctrl Pts',(90.7491633936593,-0.27355994683826,2.1882337298734));
#14078=CARTESIAN_POINT('Ctrl Pts',(90.7451283498892,-0.199126722959242,
2.19498622961592));
#14079=CARTESIAN_POINT('Ctrl Pts',(90.7415038490628,-0.132266659765372,
2.20105170059747));
#14080=CARTESIAN_POINT('Ctrl Pts',(90.7378793482364,-0.0651590566933283,
2.20405678565228));
#14081=CARTESIAN_POINT('Ctrl Pts',(90.73425484741,0.00189326415692431,2.2039991868308));
#14082=CARTESIAN_POINT('',(90.3498699627424,-0.173992556915814,-2.19712143272462));
#14083=CARTESIAN_POINT('Ctrl Pts',(90.7342548473723,0.00189326485402265,
2.2039991868302));
#14084=CARTESIAN_POINT('Ctrl Pts',(90.7293515116983,0.0926036971570066,
2.20392126535256));
#14085=CARTESIAN_POINT('Ctrl Pts',(90.7244481760243,0.183069156407198,2.19823945073773));
#14086=CARTESIAN_POINT('Ctrl Pts',(90.7195448403504,0.272680382344514,2.18706685062082));
#14087=CARTESIAN_POINT('Ctrl Pts',(90.7145706549739,0.363586426567747,2.17573281440277));
#14088=CARTESIAN_POINT('Ctrl Pts',(90.7095964695975,0.453613385733587,2.15874824234606));
#14089=CARTESIAN_POINT('Ctrl Pts',(90.7046222842211,0.542147312526976,2.13628001243278));
#14090=CARTESIAN_POINT('Ctrl Pts',(90.7026354898581,0.577509626829502,2.12730572837251));
#14091=CARTESIAN_POINT('Ctrl Pts',(90.7006486954952,0.612633990132352,2.1174571311083));
#14092=CARTESIAN_POINT('Ctrl Pts',(90.6986619011323,0.647482235274794,2.10674696036414));
#14093=CARTESIAN_POINT('Ctrl Pts',(90.69459339391,0.718843589872206,2.08481494372605));
#14094=CARTESIAN_POINT('Ctrl Pts',(90.6905248866878,0.789228822454979,2.05921012796652));
#14095=CARTESIAN_POINT('Ctrl Pts',(90.6864563794656,0.858232167974168,2.03003781882367));
#14096=CARTESIAN_POINT('Ctrl Pts',(90.6823938680067,0.927133823190694,2.0009085009434));
#14097=CARTESIAN_POINT('Ctrl Pts',(90.6783313565478,0.994657197189147,1.96822231187987));
#14098=CARTESIAN_POINT('Ctrl Pts',(90.6742688450889,1.06041176445151,1.93213428358715));
#14099=CARTESIAN_POINT('Ctrl Pts',(90.6702110880305,1.12608937844223,1.89608848949899));
#14100=CARTESIAN_POINT('Ctrl Pts',(90.6661533309721,1.19000188064749,1.85664899444771));
#14101=CARTESIAN_POINT('Ctrl Pts',(90.6620955739137,1.25178034377629,1.81401818373888));
#14102=CARTESIAN_POINT('Ctrl Pts',(90.6580403905352,1.31351962319224,1.77141441212039));
#14103=CARTESIAN_POINT('Ctrl Pts',(90.6539852071567,1.37312715631856,1.72562361233344));
#14104=CARTESIAN_POINT('Ctrl Pts',(90.6499300237782,1.43026135950486,1.67689249610919));
#14105=CARTESIAN_POINT('Ctrl Pts',(90.6458760942468,1.48737789701539,1.62817644735856));
#14106=CARTESIAN_POINT('Ctrl Pts',(90.6418221647154,1.54202225889323,1.5765221974819));
#14107=CARTESIAN_POINT('Ctrl Pts',(90.637768235184,1.59388573328848,1.52221689296218));
#14108=CARTESIAN_POINT('Ctrl Pts',(90.6337142413437,1.64575003041188,1.46791072697873));
#14109=CARTESIAN_POINT('Ctrl Pts',(90.6296602475034,1.69483302317828,1.41095377023961));
#14110=CARTESIAN_POINT('Ctrl Pts',(90.6256062536631,1.74086383325701,1.3516690105413));
#14111=CARTESIAN_POINT('Ctrl Pts',(90.6215480517177,1.78694242399259,1.2923227123918));
#14112=CARTESIAN_POINT('Ctrl Pts',(90.6174898497722,1.82996221123045,1.23064416509488));
#14113=CARTESIAN_POINT('Ctrl Pts',(90.6134316478268,1.86969399292404,1.1669877346501));
#14114=CARTESIAN_POINT('Ctrl Pts',(90.6093712990548,1.9094467931002,1.10329762936072));
#14115=CARTESIAN_POINT('Ctrl Pts',(90.6053109502827,1.94590789183945,1.03762797640211));
#14116=CARTESIAN_POINT('Ctrl Pts',(90.6012506015106,1.97889400045801,0.970357941664474));
#14117=CARTESIAN_POINT('Ctrl Pts',(90.5971829001436,2.01193984125961,0.902966092435923));
#14118=CARTESIAN_POINT('Ctrl Pts',(90.5931151987766,2.04149793453685,0.833968513628197));
#14119=CARTESIAN_POINT('Ctrl Pts',(90.5890474974096,2.06743327901196,0.763764123819556));
#14120=CARTESIAN_POINT('Ctrl Pts',(90.5858687266441,2.08770087178042,0.708901772383852));
#14121=CARTESIAN_POINT('Ctrl Pts',(90.5826899558786,2.10575706487792,0.65330285978906));
#14122=CARTESIAN_POINT('Ctrl Pts',(90.5795111851131,2.12155908224672,0.597162507644661));
#14123=CARTESIAN_POINT('Ctrl Pts',(90.5754307648268,2.14184329806247,0.525098100152149));
#14124=CARTESIAN_POINT('Ctrl Pts',(90.5713503445405,2.15849006587881,0.451862267806355));
#14125=CARTESIAN_POINT('Ctrl Pts',(90.5672699242542,2.17136853336895,0.377855385425647));
#14126=CARTESIAN_POINT('Ctrl Pts',(90.5631955068217,2.18422805488017,0.303957377244081));
#14127=CARTESIAN_POINT('Ctrl Pts',(90.5591210893891,2.1933302027879,0.229291036095995));
#14128=CARTESIAN_POINT('Ctrl Pts',(90.5550466719565,2.19859422016187,0.154270720069698));
#14129=CARTESIAN_POINT('Ctrl Pts',(90.5509770756259,2.203852008826,0.0793391727055896));
#14130=CARTESIAN_POINT('Ctrl Pts',(90.5469074792952,2.20528065798668,0.00405495480358915));
#14131=CARTESIAN_POINT('Ctrl Pts',(90.5428378829645,2.20285093137833,-0.0711602004328078));
#14132=CARTESIAN_POINT('Ctrl Pts',(90.5387709070012,2.20042276924367,-0.146326925474719));
#14133=CARTESIAN_POINT('Ctrl Pts',(90.5347039310379,2.19414117723868,-0.221424201966485));
#14134=CARTESIAN_POINT('Ctrl Pts',(90.5306369550746,2.18402899022925,-0.296029339488884));
#14135=CARTESIAN_POINT('Ctrl Pts',(90.5265712960636,2.17392007770856,-0.370610318668107));
#14136=CARTESIAN_POINT('Ctrl Pts',(90.5225056370525,2.1599830970921,-0.444699004357614));
#14137=CARTESIAN_POINT('Ctrl Pts',(90.5184399780414,2.14229267328171,-0.517878462579325));
#14138=CARTESIAN_POINT('Ctrl Pts',(90.5143743342984,2.12460231590537,-0.59105764598521));
#14139=CARTESIAN_POINT('Ctrl Pts',(90.5103086905554,2.10315865683447,-0.663327146850329));
#14140=CARTESIAN_POINT('Ctrl Pts',(90.5062430468124,2.07808694434501,-0.734282405987527));
#14141=CARTESIAN_POINT('Ctrl Pts',(90.502173398398,2.05299053614314,-0.805307556268941));
#14142=CARTESIAN_POINT('Ctrl Pts',(90.4981037499836,2.02425909656417,-0.87501543016943));
#14143=CARTESIAN_POINT('Ctrl Pts',(90.4940341015693,1.99206683038161,-0.943019481926743));
#14144=CARTESIAN_POINT('Ctrl Pts',(90.4899624013569,1.95985833379771,-1.01105781934278));
#14145=CARTESIAN_POINT('Ctrl Pts',(90.4858907011445,1.92418576047148,-1.07739020419027));
#14146=CARTESIAN_POINT('Ctrl Pts',(90.4818190009322,1.88526907726728,-1.14165516085189));
#14147=CARTESIAN_POINT('Ctrl Pts',(90.4777402319407,1.84628483176121,-1.20603168633299));
#14148=CARTESIAN_POINT('Ctrl Pts',(90.4736614629492,1.80404549352595,-1.26833321975903));
#14149=CARTESIAN_POINT('Ctrl Pts',(90.4695826939577,1.75881383871552,-1.3282280981604));
#14150=CARTESIAN_POINT('Ctrl Pts',(90.4665086190031,1.72472377441067,-1.37336949890708));
#14151=CARTESIAN_POINT('Ctrl Pts',(90.4634345440486,1.68893488061178,-1.41714447270139));
#14152=CARTESIAN_POINT('Ctrl Pts',(90.460360469094,1.65157360542284,-1.45942475855064));
#14153=CARTESIAN_POINT('Ctrl Pts',(90.4563285283101,1.60257075044973,-1.51487936242095));
#14154=CARTESIAN_POINT('Ctrl Pts',(90.4522965875262,1.55066908945272,-1.56797917703271));
#14155=CARTESIAN_POINT('Ctrl Pts',(90.4482646467423,1.49612610620718,-1.61840127110842));
#14156=CARTESIAN_POINT('Ctrl Pts',(90.4441648682423,1.44066543304279,-1.66967172082342));
#14157=CARTESIAN_POINT('Ctrl Pts',(90.4400650897423,1.38247400094061,-1.7181730728207));
#14158=CARTESIAN_POINT('Ctrl Pts',(90.4359653112423,1.32186546120693,-1.76360077751973));
#14159=CARTESIAN_POINT('Ctrl Pts',(90.4319438182175,1.26241424456713,-1.80816103792821));
#14160=CARTESIAN_POINT('Ctrl Pts',(90.4279223251928,1.20063782125386,-1.84976368663127));
#14161=CARTESIAN_POINT('Ctrl Pts',(90.4239008321681,1.13686783732387,-1.88815982386517));
#14162=CARTESIAN_POINT('Ctrl Pts',(90.4198816825718,1.07313501382011,-1.92653358667247));
#14163=CARTESIAN_POINT('Ctrl Pts',(90.4158625329755,1.00741135105409,-1.96170429303847));
#14164=CARTESIAN_POINT('Ctrl Pts',(90.4118433833792,0.940057517603746,-1.99346629356924));
#14165=CARTESIAN_POINT('Ctrl Pts',(90.4078252133142,0.872720099363314,-2.02522055319086));
#14166=CARTESIAN_POINT('Ctrl Pts',(90.4038070432492,0.803753740473402,-2.05356754842303));
#14167=CARTESIAN_POINT('Ctrl Pts',(90.3997888731841,0.73354218103753,-2.07834835112854));
#14168=CARTESIAN_POINT('Ctrl Pts',(90.3956289639807,0.660853940480139,-2.10400328548316));
#14169=CARTESIAN_POINT('Ctrl Pts',(90.3914690547772,0.586831519709844,-2.12583550938633));
#14170=CARTESIAN_POINT('Ctrl Pts',(90.3873091455737,0.511919365077974,-2.1437244607594));
#14171=CARTESIAN_POINT('Ctrl Pts',(90.3832864722748,0.439478571430073,-2.16102325347684));
#14172=CARTESIAN_POINT('Ctrl Pts',(90.3792637989758,0.366206342913574,-2.17463487349386));
#14173=CARTESIAN_POINT('Ctrl Pts',(90.3752411256769,0.292514097319783,-2.18450257561514));
#14174=CARTESIAN_POINT('Ctrl Pts',(90.3710125985211,0.21505076920307,-2.19487524157232));
#14175=CARTESIAN_POINT('Ctrl Pts',(90.3667840713654,0.137123900085511,-2.20111050061073));
#14176=CARTESIAN_POINT('Ctrl Pts',(90.3625555442096,0.0592135968959411,
-2.20320442763323));
#14177=CARTESIAN_POINT('Ctrl Pts',(90.3583270170539,-0.018696706293629,
-2.20529835465572));
#14178=CARTESIAN_POINT('Ctrl Pts',(90.3540984898981,-0.0965898279897558,
-2.20325104327665));
#14179=CARTESIAN_POINT('Ctrl Pts',(90.3498699627424,-0.173992556915814,
-2.19712143272462));
#14180=CARTESIAN_POINT('Ctrl Pts',(90.3498698986825,-0.173992556915814,
-2.19712143272462));
#14181=CARTESIAN_POINT('Ctrl Pts',(90.3498698986825,-0.18736228019796,-2.19593968129474));
#14182=CARTESIAN_POINT('Ctrl Pts',(90.3498698986825,-0.200732003480107,
-2.19475792986486));
#14183=CARTESIAN_POINT('Ctrl Pts',(90.3498698986825,-0.214101726762253,
-2.19357617843498));
#14184=CARTESIAN_POINT('Origin',(88.3562164250559,0.,0.));
#14185=CARTESIAN_POINT('',(99.9812164250558,-0.00144200395415034,1.77624941467256));
#14186=CARTESIAN_POINT('Ctrl Pts',(99.7906304259995,1.77562736014833,-0.0475451276259355));
#14187=CARTESIAN_POINT('Ctrl Pts',(99.8210626774041,1.7831651598518,0.405131671463454));
#14188=CARTESIAN_POINT('Ctrl Pts',(99.8845910813172,1.43986119934285,1.36540427831042));
#14189=CARTESIAN_POINT('Ctrl Pts',(99.9481194852301,0.490085748425745,1.77315870757737));
#14190=CARTESIAN_POINT('Ctrl Pts',(99.9812156377384,-0.00143133121117253,
1.77750555846212));
#14191=CARTESIAN_POINT('',(100.349866562796,-0.0937295438502085,-1.77377530569958));
#14192=CARTESIAN_POINT('Ctrl Pts',(99.9812164250558,-0.00144200395415034,
1.77624941467256));
#14193=CARTESIAN_POINT('Ctrl Pts',(99.9878369154481,-0.0996938618182821,
1.77616965134294));
#14194=CARTESIAN_POINT('Ctrl Pts',(99.9944574058404,-0.197622103560606,
1.7679352862269));
#14195=CARTESIAN_POINT('Ctrl Pts',(100.001077896233,-0.294176170481509,
1.75172042381792));
#14196=CARTESIAN_POINT('Ctrl Pts',(100.005371895501,-0.356800397409599,
1.74120358847903));
#14197=CARTESIAN_POINT('Ctrl Pts',(100.009665894769,-0.418989179132037,
1.72730256288422));
#14198=CARTESIAN_POINT('Ctrl Pts',(100.013959894037,-0.480348386519703,
1.71006710104251));
#14199=CARTESIAN_POINT('Ctrl Pts',(100.018387757296,-0.543620446671693,
1.69229432944351));
#14200=CARTESIAN_POINT('Ctrl Pts',(100.022815620555,-0.606009799062529,
1.67097574429));
#14201=CARTESIAN_POINT('Ctrl Pts',(100.027243483814,-0.667092358067373,
1.6462235110422));
#14202=CARTESIAN_POINT('Ctrl Pts',(100.031525654997,-0.726165088785864,
1.62228571221467));
#14203=CARTESIAN_POINT('Ctrl Pts',(100.03580782618,-0.784015179020576,1.59513692650705));
#14204=CARTESIAN_POINT('Ctrl Pts',(100.040089997363,-0.840273973818524,
1.5649292991772));
#14205=CARTESIAN_POINT('Ctrl Pts',(100.044369556558,-0.896498452547865,
1.53474009753555));
#14206=CARTESIAN_POINT('Ctrl Pts',(100.048649115754,-0.951133116423197,
1.50149599247278));
#14207=CARTESIAN_POINT('Ctrl Pts',(100.052928674949,-1.00383183752556,1.46539609132482));
#14208=CARTESIAN_POINT('Ctrl Pts',(100.057207173385,-1.05651749638528,1.42930513812965));
#14209=CARTESIAN_POINT('Ctrl Pts',(100.061485671822,-1.10726774841054,1.39036007930979));
#14210=CARTESIAN_POINT('Ctrl Pts',(100.065764170258,-1.1557652101126,1.34880348516504));
#14211=CARTESIAN_POINT('Ctrl Pts',(100.070043157405,-1.20426821143078,1.30724214422387));
#14212=CARTESIAN_POINT('Ctrl Pts',(100.074322144552,-1.25051753036019,1.26306900710094));
#14213=CARTESIAN_POINT('Ctrl Pts',(100.0786011317,-1.29423019245069,1.2165657694712));
#14214=CARTESIAN_POINT('Ctrl Pts',(100.082884940889,-1.3379921148689,1.17001012678042));
#14215=CARTESIAN_POINT('Ctrl Pts',(100.087168750079,-1.37921133261949,1.12111951512464));
#14216=CARTESIAN_POINT('Ctrl Pts',(100.091452559268,-1.41764381670143,1.07021029310514));
#14217=CARTESIAN_POINT('Ctrl Pts',(100.095739280734,-1.45610242845962,1.0192664613095));
#14218=CARTESIAN_POINT('Ctrl Pts',(100.100026002199,-1.49177025680286,0.966301708503973));
#14219=CARTESIAN_POINT('Ctrl Pts',(100.104312723664,-1.52444711914087,0.911660596627439));
#14220=CARTESIAN_POINT('Ctrl Pts',(100.108606769025,-1.55717981014966,0.856926129990768));
#14221=CARTESIAN_POINT('Ctrl Pts',(100.112900814387,-1.58691110996872,0.800510038579124));
#14222=CARTESIAN_POINT('Ctrl Pts',(100.117194859749,-1.61348773066646,0.74277951337445));
#14223=CARTESIAN_POINT('Ctrl Pts',(100.118206110583,-1.61974654434729,0.729183932316125));
#14224=CARTESIAN_POINT('Ctrl Pts',(100.119217361417,-1.62583061331469,0.715515525215639));
#14225=CARTESIAN_POINT('Ctrl Pts',(100.120228612252,-1.63173833712494,0.701779211473773));
#14226=CARTESIAN_POINT('Ctrl Pts',(100.124535184851,-1.65689731907099,0.643280933535056));
#14227=CARTESIAN_POINT('Ctrl Pts',(100.12884175745,-1.67895697168689,0.58331082626553));
#14228=CARTESIAN_POINT('Ctrl Pts',(100.13314833005,-1.69774574538958,0.522229304531615));
#14229=CARTESIAN_POINT('Ctrl Pts',(100.137574621642,-1.71705683074985,0.459449769325994));
#14230=CARTESIAN_POINT('Ctrl Pts',(100.142000913235,-1.73291216433171,0.395496553854958));
#14231=CARTESIAN_POINT('Ctrl Pts',(100.146427204827,-1.74517774248642,0.330784990031285));
#14232=CARTESIAN_POINT('Ctrl Pts',(100.150721876997,-1.75707859358033,0.267997677814478));
#14233=CARTESIAN_POINT('Ctrl Pts',(100.155016549166,-1.76560009894012,0.204497020559692));
#14234=CARTESIAN_POINT('Ctrl Pts',(100.159311221335,-1.7706704910092,0.140677200602032));
#14235=CARTESIAN_POINT('Ctrl Pts',(100.163603221152,-1.77573772803597,0.0768970924121892));
#14236=CARTESIAN_POINT('Ctrl Pts',(100.16789522097,-1.77735807128689,0.0127987147216979));
#14237=CARTESIAN_POINT('Ctrl Pts',(100.172187220787,-1.7755114340142,-0.0512172840440753));
#14238=CARTESIAN_POINT('Ctrl Pts',(100.176478080179,-1.77366528741048,-0.115216273153953));
#14239=CARTESIAN_POINT('Ctrl Pts',(100.180768939572,-1.7683540036489,-0.179132425294061));
#14240=CARTESIAN_POINT('Ctrl Pts',(100.185059798964,-1.75960959918077,-0.242565704440833));
#14241=CARTESIAN_POINT('Ctrl Pts',(100.189351048018,-1.75086440061465,-0.306004744098857));
#14242=CARTESIAN_POINT('Ctrl Pts',(100.193642297073,-1.73868553421696,-0.36896032699504));
#14243=CARTESIAN_POINT('Ctrl Pts',(100.197933546127,-1.72315655021774,-0.431040097835106));
#14244=CARTESIAN_POINT('Ctrl Pts',(100.202229394063,-1.7076109239893,-0.493186398834279));
#14245=CARTESIAN_POINT('Ctrl Pts',(100.206525241998,-1.68870814086263,-0.554454527962565));
#14246=CARTESIAN_POINT('Ctrl Pts',(100.210821089934,-1.66658200046735,-0.614466026903244));
#14247=CARTESIAN_POINT('Ctrl Pts',(100.215119733224,-1.6444414623536,-0.674516575974281));
#14248=CARTESIAN_POINT('Ctrl Pts',(100.219418376514,-1.61907359253653,-0.733308407332166));
#14249=CARTESIAN_POINT('Ctrl Pts',(100.223717019804,-1.5906597058994,-0.790484511251187));
#14250=CARTESIAN_POINT('Ctrl Pts',(100.228022711847,-1.56219922724194,-0.847754370390336));
#14251=CARTESIAN_POINT('Ctrl Pts',(100.232328403891,-1.5306830169525,-0.903402782285414));
#14252=CARTESIAN_POINT('Ctrl Pts',(100.236634095934,-1.49633689103465,-0.957099770676374));
#14253=CARTESIAN_POINT('Ctrl Pts',(100.23754917338,-1.48903739890877,-0.968511850888292));
#14254=CARTESIAN_POINT('Ctrl Pts',(100.238464250825,-1.48161023276245,-0.979835905416706));
#14255=CARTESIAN_POINT('Ctrl Pts',(100.239379328271,-1.47405779327266,-0.991068960563359));
#14256=CARTESIAN_POINT('Ctrl Pts',(100.243634734529,-1.43893650552586,-1.04330630223483));
#14257=CARTESIAN_POINT('Ctrl Pts',(100.247890140788,-1.400957248599,-1.09378977273184));
#14258=CARTESIAN_POINT('Ctrl Pts',(100.252145547047,-1.36032286525451,-1.14218464565313));
#14259=CARTESIAN_POINT('Ctrl Pts',(100.256393671885,-1.31975801135417,-1.19049671016595));
#14260=CARTESIAN_POINT('Ctrl Pts',(100.260641796723,-1.27654737586528,-1.23672687879013));
#14261=CARTESIAN_POINT('Ctrl Pts',(100.264889921561,-1.23093680649601,-1.28056965484639));
#14262=CARTESIAN_POINT('Ctrl Pts',(100.269134011856,-1.18536955455418,-1.32437079238998));
#14263=CARTESIAN_POINT('Ctrl Pts',(100.27337810215,-1.13740725348595,-1.36578867404023));
#14264=CARTESIAN_POINT('Ctrl Pts',(100.277622192445,-1.08733459704232,-1.40455243283219));
#14265=CARTESIAN_POINT('Ctrl Pts',(100.281863854929,-1.03729058441089,-1.44329401701018));
#14266=CARTESIAN_POINT('Ctrl Pts',(100.286105517412,-0.985139015793631,
-1.47938417314215));
#14267=CARTESIAN_POINT('Ctrl Pts',(100.290347179896,-0.931198259671605,
-1.5125917703348));
#14268=CARTESIAN_POINT('Ctrl Pts',(100.294588017752,-0.877267990261508,
-1.54579291158337));
#14269=CARTESIAN_POINT('Ctrl Pts',(100.298828855607,-0.82154966262879,-1.57611233701221));
#14270=CARTESIAN_POINT('Ctrl Pts',(100.303069693462,-0.764389468949105,
-1.60336296647381));
#14271=CARTESIAN_POINT('Ctrl Pts',(100.307314102526,-0.707181140686356,
-1.63063654368285));
#14272=CARTESIAN_POINT('Ctrl Pts',(100.311558511589,-0.648528986995092,
-1.65483594102652));
#14273=CARTESIAN_POINT('Ctrl Pts',(100.315802920653,-0.588801348259254,
-1.67582130156771));
#14274=CARTESIAN_POINT('Ctrl Pts',(100.320049173466,-0.529047764143368,
-1.69681577804193));
#14275=CARTESIAN_POINT('Ctrl Pts',(100.324295426279,-0.468218259647601,
-1.71459329296513));
#14276=CARTESIAN_POINT('Ctrl Pts',(100.328541679092,-0.406695647801983,
-1.72906411464669));
#14277=CARTESIAN_POINT('Ctrl Pts',(100.332795245003,-0.345067078799047,
-1.74355985866303));
#14278=CARTESIAN_POINT('Ctrl Pts',(100.337048810914,-0.282743526677385,
-1.75473744840853));
#14279=CARTESIAN_POINT('Ctrl Pts',(100.341302376825,-0.22011620541515,-1.76255862841882));
#14280=CARTESIAN_POINT('Ctrl Pts',(100.344157105482,-0.178084645905708,
-1.76780771757689));
#14281=CARTESIAN_POINT('Ctrl Pts',(100.347011834139,-0.135916384823446,
-1.77154607556643));
#14282=CARTESIAN_POINT('Ctrl Pts',(100.349866562796,-0.0937295438502085,
-1.77377530569958));
#14283=CARTESIAN_POINT('',(100.349869898682,-1.70764710160359,-0.4888818250711));
#14284=CARTESIAN_POINT('Origin',(100.349869898682,0.,0.));
#14285=CARTESIAN_POINT('',(100.129086863397,0.00137170632050479,1.77624947035088));
#14286=CARTESIAN_POINT('Ctrl Pts',(100.129086863397,0.0013717063205048,
1.77624947035088));
#14287=CARTESIAN_POINT('Ctrl Pts',(100.133321543366,-0.0614516234439551,
1.77629798558477));
#14288=CARTESIAN_POINT('Ctrl Pts',(100.137556223336,-0.124412816603254,
1.77300913712713));
#14289=CARTESIAN_POINT('Ctrl Pts',(100.141790903305,-0.187116606352544,
1.76636673375806));
#14290=CARTESIAN_POINT('Ctrl Pts',(100.145973038684,-0.249042357382847,
1.75980675039947));
#14291=CARTESIAN_POINT('Ctrl Pts',(100.150155174062,-0.310716513623133,
1.7499760021445));
#14292=CARTESIAN_POINT('Ctrl Pts',(100.154337309441,-0.371757544232495,
1.73691116376349));
#14293=CARTESIAN_POINT('Ctrl Pts',(100.15851669033,-0.432758371246943,1.72385493030713));
#14294=CARTESIAN_POINT('Ctrl Pts',(100.162696071219,-0.493126381012677,
1.70756893339161));
#14295=CARTESIAN_POINT('Ctrl Pts',(100.166875452108,-0.55248794642649,1.68814132452039));
#14296=CARTESIAN_POINT('Ctrl Pts',(100.171053739036,-0.611833973827677,
1.66871880086599));
#14297=CARTESIAN_POINT('Ctrl Pts',(100.175232025963,-0.670173575397997,
1.64615646001032));
#14298=CARTESIAN_POINT('Ctrl Pts',(100.179410312891,-0.727148330130597,
1.62059228940788));
#14299=CARTESIAN_POINT('Ctrl Pts',(100.183686052038,-0.78545193480656,1.59443187320832));
#14300=CARTESIAN_POINT('Ctrl Pts',(100.187961791186,-0.84232567474615,1.56512802426334));
#14301=CARTESIAN_POINT('Ctrl Pts',(100.192237530334,-0.897409713425917,
1.53287960021289));
#14302=CARTESIAN_POINT('Ctrl Pts',(100.196421458131,-0.951310953100947,
1.50132363453668));
#14303=CARTESIAN_POINT('Ctrl Pts',(100.200605385927,-1.00349818563022,1.4669486694603));
#14304=CARTESIAN_POINT('Ctrl Pts',(100.204789313724,-1.05366400520113,1.42998469454869));
#14305=CARTESIAN_POINT('Ctrl Pts',(100.209110958547,-1.10548106920959,1.39180402351839));
#14306=CARTESIAN_POINT('Ctrl Pts',(100.213432603371,-1.15514082602271,1.35086129312065));
#14307=CARTESIAN_POINT('Ctrl Pts',(100.217754248194,-1.20234438202791,1.3074525037285));
#14308=CARTESIAN_POINT('Ctrl Pts',(100.222075893017,-1.24954793803311,1.26404371433635));
#14309=CARTESIAN_POINT('Ctrl Pts',(100.22639753784,-1.29429493562015,1.21816937064235));
#14310=CARTESIAN_POINT('Ctrl Pts',(100.230719182663,-1.33633294203061,1.17016166855004));
#14311=CARTESIAN_POINT('Ctrl Pts',(100.235133769944,-1.37927502912348,1.12112149989295));
#14312=CARTESIAN_POINT('Ctrl Pts',(100.239548357224,-1.41958668769332,1.06963211146007));
#14313=CARTESIAN_POINT('Ctrl Pts',(100.243962944504,-1.45698615668822,1.01599970557028));
#14314=CARTESIAN_POINT('Ctrl Pts',(100.248375734261,-1.49437039744277,0.962389137615333));
#14315=CARTESIAN_POINT('Ctrl Pts',(100.252788524019,-1.52884448547413,0.906637633133585));
#14316=CARTESIAN_POINT('Ctrl Pts',(100.257201313776,-1.5601656568966,0.849086088415297));
#14317=CARTESIAN_POINT('Ctrl Pts',(100.2616010349,-1.59139406955399,0.791704984647155));
#14318=CARTESIAN_POINT('Ctrl Pts',(100.266000756023,-1.61948795076751,0.732534878825622));
#14319=CARTESIAN_POINT('Ctrl Pts',(100.270400477146,-1.64424956134948,0.671943035161504));
#14320=CARTESIAN_POINT('Ctrl Pts',(100.274795966228,-1.66898735401991,0.611409474102507));
#14321=CARTESIAN_POINT('Ctrl Pts',(100.27919145531,-1.69039906627075,0.549457326576857));
#14322=CARTESIAN_POINT('Ctrl Pts',(100.283586944391,-1.70833399824872,0.48647611753049));
#14323=CARTESIAN_POINT('Ctrl Pts',(100.287979471106,-1.72625684286847,0.423537355059128));
#14324=CARTESIAN_POINT('Ctrl Pts',(100.292371997821,-1.74070743551343,0.359571361705321));
#14325=CARTESIAN_POINT('Ctrl Pts',(100.296764524535,-1.75158461763224,0.294983711031818));
#14326=CARTESIAN_POINT('Ctrl Pts',(100.301189972381,-1.76254332210949,0.229911988514088));
#14327=CARTESIAN_POINT('Ctrl Pts',(100.305615420226,-1.76987468773199,0.164209716463454));
#14328=CARTESIAN_POINT('Ctrl Pts',(100.310040868072,-1.77352778075399,0.098301950101844));
#14329=CARTESIAN_POINT('Ctrl Pts',(100.314432487141,-1.77715294899391,0.0328979924311582));
#14330=CARTESIAN_POINT('Ctrl Pts',(100.31882410621,-1.77715590345277,-0.0327078499729776));
#14331=CARTESIAN_POINT('Ctrl Pts',(100.32321572528,-1.77353911854442,-0.098097183918244));
#14332=CARTESIAN_POINT('Ctrl Pts',(100.327658087513,-1.76988054332853,-0.164242061929393));
#14333=CARTESIAN_POINT('Ctrl Pts',(100.332100449747,-1.76251803703616,-0.230164902592036));
#14334=CARTESIAN_POINT('Ctrl Pts',(100.336542811981,-1.75150823419927,-0.295436910409244));
#14335=CARTESIAN_POINT('Ctrl Pts',(100.340985174215,-1.74049843136238,-0.360708918226453));
#14336=CARTESIAN_POINT('Ctrl Pts',(100.345427536448,-1.72584144827217,-0.42532960905316));
#14337=CARTESIAN_POINT('Ctrl Pts',(100.349869898682,-1.7076471016036,-0.488881825071076));
#14338=CARTESIAN_POINT('Ctrl Pts',(99.9383713772532,1.77277786422444,-0.0474589613121508));
#14339=CARTESIAN_POINT('Ctrl Pts',(99.9563868350438,1.78061088145064,0.221455662094678));
#14340=CARTESIAN_POINT('Ctrl Pts',(100.014119198174,1.61989353132562,1.08753612952137));
#14341=CARTESIAN_POINT('Ctrl Pts',(100.077691015475,0.763768868856085,1.73402760988346));
#14342=CARTESIAN_POINT('Ctrl Pts',(100.123247374986,0.0880846415247775,
1.77868931994825));
#14343=CARTESIAN_POINT('Ctrl Pts',(100.129086829157,0.00137347567789877,
1.77788227080619));
#14344=CARTESIAN_POINT('Origin',(25.4947388265965,0.,-6.40787078036307));
#14345=CARTESIAN_POINT('',(25.4947388265965,-7.48009298981943E-16,6.107959450045));
#14346=CARTESIAN_POINT('Origin',(25.4947388265965,0.,0.));
#14347=CARTESIAN_POINT('',(25.4947388265965,-7.47987577963046E-16,6.10778208446569));
#14348=CARTESIAN_POINT('Origin',(25.4947388265965,0.,0.));
#14349=CARTESIAN_POINT('Origin',(27.4542764744824,0.,0.));
#14350=CARTESIAN_POINT('',(27.7542764744824,-7.48069377062962E-16,6.10845002480549));
#14351=CARTESIAN_POINT('Origin',(27.7542764744824,0.,0.));
#14352=CARTESIAN_POINT('',(27.4541877916966,-7.84808779432149E-16,6.40845001169777));
#14353=CARTESIAN_POINT('Origin',(27.4542764744824,-7.48069377062961E-16,
6.10845002480549));
#14354=CARTESIAN_POINT('Origin',(27.4541877916966,-7.84808779432149E-16,
0.));
#14355=CARTESIAN_POINT('Origin',(26.6245076505395,0.,0.));
#14356=CARTESIAN_POINT('',(25.7946501438108,-7.8474870135113E-16,6.40795943693727));
#14357=CARTESIAN_POINT('',(26.6245076505395,-7.84778743602106E-16,6.40820475053297));
#14358=CARTESIAN_POINT('Origin',(25.7946501438108,-7.8474870135113E-16,
0.));
#14359=CARTESIAN_POINT('Origin',(25.7947388265966,0.,0.));
#14360=CARTESIAN_POINT('Origin',(25.7947388265966,-7.48009298981944E-16,
6.107959450045));
#14361=CARTESIAN_POINT('Origin',(27.7542764744824,0.,-6.40853872070288));
#14362=CARTESIAN_POINT('',(27.7542764744824,-7.4809109808186E-16,6.1086273903848));
#14363=CARTESIAN_POINT('Origin',(27.7542764744824,0.,0.));
#14364=CARTESIAN_POINT('Ctrl Pts',(90.1010424233136,1.30583205915545,-1.19933150781794));
#14365=CARTESIAN_POINT('Ctrl Pts',(90.1407593286533,1.70488751242686,-0.764839959096196));
#14366=CARTESIAN_POINT('Ctrl Pts',(90.2201931393327,2.02794301306985,0.526632618699088));
#14367=CARTESIAN_POINT('Ctrl Pts',(90.3393438553519,0.654151350163486,1.99272616320641));
#14368=CARTESIAN_POINT('Ctrl Pts',(90.4584945713711,-1.31950283566344,1.628071155055));
#14369=CARTESIAN_POINT('Ctrl Pts',(90.5776452873901,-2.08378435372669,-0.226191237424723));
#14370=CARTESIAN_POINT('Ctrl Pts',(90.6967960034093,-0.938691037125564,
-1.8743255371654));
#14371=CARTESIAN_POINT('Ctrl Pts',(90.8159467194284,1.06664039468703,-1.80433079412335));
#14372=CARTESIAN_POINT('Ctrl Pts',(90.9350974354475,2.09451613140419,-0.0812095856050628));
#14373=CARTESIAN_POINT('Ctrl Pts',(91.0542481514668,1.20307845886324,1.71647344469004));
#14374=CARTESIAN_POINT('Ctrl Pts',(91.1733988674858,-0.790818539461979,
1.94117803796467));
#14375=CARTESIAN_POINT('Ctrl Pts',(91.292549583505,-2.06003807063084,0.387103249808451));
#14376=CARTESIAN_POINT('Ctrl Pts',(91.4117002995241,-1.44152521409774,-1.52171537550226));
#14377=CARTESIAN_POINT('Ctrl Pts',(91.5308510155432,0.49794312834491,-2.03608731373934));
#14378=CARTESIAN_POINT('Ctrl Pts',(91.6500017315624,1.9811163478004,-0.68467704960091));
#14379=CARTESIAN_POINT('Ctrl Pts',(91.7691524475815,1.64887612811511,1.29414546959417));
#14380=CARTESIAN_POINT('Ctrl Pts',(91.8883031636006,-0.194326599410635,
2.08706505065828));
#14381=CARTESIAN_POINT('Ctrl Pts',(92.0074538796198,-1.8594563484299,0.967484492317832));
#14382=CARTESIAN_POINT('Ctrl Pts',(92.1266045956389,-1.82065667436397,-1.0386594260208));
#14383=CARTESIAN_POINT('Ctrl Pts',(92.2457553116581,-0.113481959304491,
-2.09301834340466));
#14384=CARTESIAN_POINT('Ctrl Pts',(92.3649060276773,1.69768295626714,-1.22942125805054));
#14385=CARTESIAN_POINT('Ctrl Pts',(92.4840567436963,1.95316091651168,0.760767028860157));
#14386=CARTESIAN_POINT('Ctrl Pts',(92.6032074597155,0.418842401989782,2.05381962675591));
#14387=CARTESIAN_POINT('Ctrl Pts',(92.7223581757346,-1.49928609228867,1.46483625188328));
#14388=CARTESIAN_POINT('Ctrl Pts',(92.8415088917537,-2.04353036839276,-0.466462927017294));
#14389=CARTESIAN_POINT('Ctrl Pts',(92.9606596077729,-0.715167316040089,
-1.97031462884506));
#14390=CARTESIAN_POINT('Ctrl Pts',(93.0798103237921,1.26854570192717,-1.66865090134507));
#14391=CARTESIAN_POINT('Ctrl Pts',(93.1989610398111,2.08981552149063,0.162096002811901));
#14392=CARTESIAN_POINT('Ctrl Pts',(93.3181117558304,0.99606419884773,1.84430478488173));
#14393=CARTESIAN_POINT('Ctrl Pts',(93.4372624718494,-1.01043946011796,1.83646838400132));
#14394=CARTESIAN_POINT('Ctrl Pts',(93.5564131878686,-2.09101788353122,0.145767755972613));
#14395=CARTESIAN_POINT('Ctrl Pts',(93.6755639038877,-1.25547336955694,-1.67850845879349));
#14396=CARTESIAN_POINT('Ctrl Pts',(93.7947146199069,0.730535394209225,-1.96466843659299));
#14397=CARTESIAN_POINT('Ctrl Pts',(93.9138653359261,2.04711151637174,-0.450486922634485));
#14398=CARTESIAN_POINT('Ctrl Pts',(94.033016051945,1.48779869334798,1.47650231154474));
#14399=CARTESIAN_POINT('Ctrl Pts',(94.1521667679643,-0.434871767592548,
2.0504854482974));
#14400=CARTESIAN_POINT('Ctrl Pts',(94.2713174839834,-1.95904359527549,0.745487907170205));
#14401=CARTESIAN_POINT('Ctrl Pts',(94.3904682000025,-1.6880283048537,-1.24264414453198));
#14402=CARTESIAN_POINT('Ctrl Pts',(94.5096189160217,0.129826818626143,-2.09206812152299));
#14403=CARTESIAN_POINT('Ctrl Pts',(94.6287696320409,1.82871397582683,-1.0244067661543));
#14404=CARTESIAN_POINT('Ctrl Pts',(94.74792034806,1.85184272723222,0.981978890569559));
#14405=CARTESIAN_POINT('Ctrl Pts',(94.8670710640791,0.178018834653386,2.08851940915947));
#14406=CARTESIAN_POINT('Ctrl Pts',(94.9862217800982,-1.65893420906864,1.28122648969999));
#14407=CARTESIAN_POINT('Ctrl Pts',(95.1053724961174,-1.97570805459144,-0.700129781504567));
#14408=CARTESIAN_POINT('Ctrl Pts',(95.2245232121365,-0.48202415568645,-2.03991586622143));
#14409=CARTESIAN_POINT('Ctrl Pts',(95.3436739281557,1.45336688898623,-1.51040680411788));
#14410=CARTESIAN_POINT('Ctrl Pts',(95.4628246441747,2.05695218758971,0.403177040389243));
#14411=CARTESIAN_POINT('Ctrl Pts',(95.5819753601939,0.775630953932477,1.94730599835489));
#14412=CARTESIAN_POINT('Ctrl Pts',(95.7011260762131,-1.21644664076787,1.70700369012245));
#14413=CARTESIAN_POINT('Ctrl Pts',(95.8202767922322,-2.0938224776132,-0.0975267151544407));
#14414=CARTESIAN_POINT('Ctrl Pts',(95.9394275082513,-1.05250536220669,-1.81268764282583));
#14415=CARTESIAN_POINT('Ctrl Pts',(96.0585782242705,0.953284454331289,-1.86677603826951));
#14416=CARTESIAN_POINT('Ctrl Pts',(96.1777289402896,2.08552353599421,-0.210227516612779));
#14417=CARTESIAN_POINT('Ctrl Pts',(96.2968796563088,1.30667447477482,1.63896486994091));
#14418=CARTESIAN_POINT('Ctrl Pts',(96.4160303723279,-0.669557426892749,
1.98627714078819));
#14419=CARTESIAN_POINT('Ctrl Pts',(96.5351810883469,-2.03223439262648,0.513446590555013));
#14420=CARTESIAN_POINT('Ctrl Pts',(96.6543318043663,-1.53265519856506,-1.42988533465054));
#14421=CARTESIAN_POINT('Ctrl Pts',(96.7734825203852,0.371386293120647,-2.06292904608715));
#14422=CARTESIAN_POINT('Ctrl Pts',(96.8926332364044,1.9351046338199,-0.805589277546201));
#14423=CARTESIAN_POINT('Ctrl Pts',(97.0117839524236,1.72557253784195,1.18995942983182));
#14424=CARTESIAN_POINT('Ctrl Pts',(97.1309346684427,-0.065203384874652,
2.09507817189829));
#14425=CARTESIAN_POINT('Ctrl Pts',(97.2500853844619,-1.79622960269954,1.08035329516627));
#14426=CARTESIAN_POINT('Ctrl Pts',(97.3692361004811,-1.88126476065518,-0.924362985387572));
#14427=CARTESIAN_POINT('Ctrl Pts',(97.4883868165,-0.242386130970125,-2.0820309772158));
#14428=CARTESIAN_POINT('Ctrl Pts',(97.6075375325194,1.61860519705063,-1.33181126474651));
#14429=CARTESIAN_POINT('Ctrl Pts',(97.7266882485383,1.99637317852867,0.638825612677669));
#14430=CARTESIAN_POINT('Ctrl Pts',(97.8458389645576,0.544746742790172,2.02406892253496));
#14431=CARTESIAN_POINT('Ctrl Pts',(97.9649896805767,-1.40606323902093,1.55453858294462));
#14432=CARTESIAN_POINT('Ctrl Pts',(98.0841403965958,-2.0684146040356,-0.339507106786872));
#14433=CARTESIAN_POINT('Ctrl Pts',(98.203291112615,-0.835355735837929,-1.9224423880883));
#14434=CARTESIAN_POINT('Ctrl Pts',(98.3224418286341,1.16318880525659,-1.74373046440489));
#14435=CARTESIAN_POINT('Ctrl Pts',(98.4415925446532,2.09583493445023,0.03286460299083));
#14436=CARTESIAN_POINT('Ctrl Pts',(98.5607432606724,1.10794387479709,1.77934362145635));
#14437=CARTESIAN_POINT('Ctrl Pts',(98.6798939766915,-0.895221256089004,
1.89530574973682));
#14438=CARTESIAN_POINT('Ctrl Pts',(98.7990446927107,-2.07804279474277,0.274486409481149));
#14439=CARTESIAN_POINT('Ctrl Pts',(98.9181954087297,-1.35663041470257,-1.59785882547245));
#14440=CARTESIAN_POINT('Ctrl Pts',(99.0373461247489,0.607940744949202,-2.00599618084136));
#14441=CARTESIAN_POINT('Ctrl Pts',(99.156496840768,2.01542321899274,-0.575912342987758));
#14442=CARTESIAN_POINT('Ctrl Pts',(99.2756475567872,1.57604812382197,1.38189668529539));
#14443=CARTESIAN_POINT('Ctrl Pts',(99.3947982728063,-0.307539860164324,
2.07342665626661));
#14444=CARTESIAN_POINT('Ctrl Pts',(99.5139489888255,-1.9093366442722,0.864885194893485));
#14445=CARTESIAN_POINT('Ctrl Pts',(99.6330997048446,-1.76144452875313,-1.13606536710066));
#14446=CARTESIAN_POINT('Ctrl Pts',(99.7522504208638,0.000461070801624738,
-2.09624351397064));
#14447=CARTESIAN_POINT('Ctrl Pts',(99.8714011368828,1.76214729717201,-1.13496987263683));
#14448=CARTESIAN_POINT('Ctrl Pts',(99.990551852902,1.90866885759355,0.865266786198645));
#14449=CARTESIAN_POINT('Ctrl Pts',(100.109702568921,0.306980077402089,2.07476137965942));
#14450=CARTESIAN_POINT('Ctrl Pts',(100.228868133282,-1.57796936803118,1.37855338932855));
#14451=CARTESIAN_POINT('Ctrl Pts',(100.308316792305,-1.86701861863313,0.0786761327033587));
#14452=CARTESIAN_POINT('Ctrl Pts',(100.348048545986,-1.70435785524601,-0.488628385190746));
#14453=CARTESIAN_POINT('Ctrl Pts',(90.1845168795555,1.41231704226503,-1.29713182942698));
#14454=CARTESIAN_POINT('Ctrl Pts',(90.2242337848953,1.84391374990636,-0.827209365295778));
#14455=CARTESIAN_POINT('Ctrl Pts',(90.3036675955747,2.19331303594521,0.569577241718508));
#14456=CARTESIAN_POINT('Ctrl Pts',(90.4228183115938,0.707494576794279,2.15522440357605));
#14457=CARTESIAN_POINT('Ctrl Pts',(90.541969027613,-1.4271026117476,1.76083334926806));
#14458=CARTESIAN_POINT('Ctrl Pts',(90.6611197436321,-2.25370799754816,-0.244636159134078));
#14459=CARTESIAN_POINT('Ctrl Pts',(90.7802704596512,-1.01523725034848,-2.02716871616958));
#14460=CARTESIAN_POINT('Ctrl Pts',(90.8994211756703,1.15362032722573,-1.95146620314416));
#14461=CARTESIAN_POINT('Ctrl Pts',(91.0185718916896,2.26531490549736,-0.0878318777220926));
#14462=CARTESIAN_POINT('Ctrl Pts',(91.1377226077086,1.30118432820023,1.85644446507076));
#14463=CARTESIAN_POINT('Ctrl Pts',(91.2568733237279,-0.855306387058394,
2.099472750624));
#14464=CARTESIAN_POINT('Ctrl Pts',(91.3760240397469,-2.22802530728827,0.418669853437552));
#14465=CARTESIAN_POINT('Ctrl Pts',(91.4951747557661,-1.55907538986423,-1.64580471373058));
#14466=CARTESIAN_POINT('Ctrl Pts',(91.6143254717852,0.538548246927779,-2.20212146927492));
#14467=CARTESIAN_POINT('Ctrl Pts',(91.7334761878043,2.14266785770134,-0.740509515614525));
#14468=CARTESIAN_POINT('Ctrl Pts',(91.8526269038236,1.78333487832047,1.39967746163317));
#14469=CARTESIAN_POINT('Ctrl Pts',(91.9717776198425,-0.210173097060069,
2.25725622119186));
#14470=CARTESIAN_POINT('Ctrl Pts',(92.0909283358618,-2.01108700910122,1.0463786878623));
#14471=CARTESIAN_POINT('Ctrl Pts',(92.2100790518808,-1.96912338863914,-1.12335763101657));
#14472=CARTESIAN_POINT('Ctrl Pts',(92.3292297679001,-0.12273592457137,-2.2636949793341));
#14473=CARTESIAN_POINT('Ctrl Pts',(92.4483804839192,1.83612169320582,-1.3296752692614));
#14474=CARTESIAN_POINT('Ctrl Pts',(92.5675311999383,2.11243278133292,0.822804305132014));
#14475=CARTESIAN_POINT('Ctrl Pts',(92.6866819159575,0.452997196849331,2.22129977608434));
#14476=CARTESIAN_POINT('Ctrl Pts',(92.8058326319765,-1.62154641902396,1.58428734243238));
#14477=CARTESIAN_POINT('Ctrl Pts',(92.9249833479958,-2.21017147299464,-0.504500970697111));
#14478=CARTESIAN_POINT('Ctrl Pts',(93.0441340640148,-0.773486132028051,
-2.13098530506418));
#14479=CARTESIAN_POINT('Ctrl Pts',(93.163284780034,1.37199014311418,-1.80472219918136));
#14480=CARTESIAN_POINT('Ctrl Pts',(93.2824354960531,2.26023098108043,0.175314234054207));
#14481=CARTESIAN_POINT('Ctrl Pts',(93.4015862120723,1.07728894643049,1.99469990076979));
#14482=CARTESIAN_POINT('Ctrl Pts',(93.5207369280913,-1.09283644837499,1.98622447513156));
#14483=CARTESIAN_POINT('Ctrl Pts',(93.6398876441106,-2.26153139056953,0.157654488974653));
#14484=CARTESIAN_POINT('Ctrl Pts',(93.7590383601297,-1.35785181831264,-1.8153835980051));
#14485=CARTESIAN_POINT('Ctrl Pts',(93.8781890761489,0.790107410815714,-2.12487869013955));
#14486=CARTESIAN_POINT('Ctrl Pts',(93.9973397921678,2.21404464817526,-0.487222191930033));
#14487=CARTESIAN_POINT('Ctrl Pts',(94.1164905081872,1.60912227215037,1.59690471903944));
#14488=CARTESIAN_POINT('Ctrl Pts',(94.2356412242062,-0.470333688214142,
2.21769370972545));
#14489=CARTESIAN_POINT('Ctrl Pts',(94.3547919402254,-2.11879516722628,0.80627923684147));
#14490=CARTESIAN_POINT('Ctrl Pts',(94.4739426562444,-1.82567974653074,-1.34397642521381));
#14491=CARTESIAN_POINT('Ctrl Pts',(94.5930933722636,0.140413636809712,-2.26266727094848));
#14492=CARTESIAN_POINT('Ctrl Pts',(94.7122440882828,1.9778377283514,-1.10794272809251));
#14493=CARTESIAN_POINT('Ctrl Pts',(94.8313948043019,2.00285252986982,1.0620550418963));
#14494=CARTESIAN_POINT('Ctrl Pts',(94.9505455203211,0.192535504288173,2.25882917636812));
#14495=CARTESIAN_POINT('Ctrl Pts',(95.0696962363401,-1.79421315247794,1.38570499454195));
#14496=CARTESIAN_POINT('Ctrl Pts',(95.1888469523594,-2.13681854146269,-0.757222351284346));
#14497=CARTESIAN_POINT('Ctrl Pts',(95.3079976683784,-0.521331150576662,
-2.20626222373084));
#14498=CARTESIAN_POINT('Ctrl Pts',(95.4271483843976,1.57188270236409,-1.6335739770307));
#14499=CARTESIAN_POINT('Ctrl Pts',(95.5462991004167,2.22468778376917,0.436054392446108));
#14500=CARTESIAN_POINT('Ctrl Pts',(95.6654498164359,0.838880319308144,2.10610041980454));
#14501=CARTESIAN_POINT('Ctrl Pts',(95.784600532455,-1.31564262779213,1.84620249278336));
#14502=CARTESIAN_POINT('Ctrl Pts',(95.9037512484742,-2.26456468722573,-0.105479598944601));
#14503=CARTESIAN_POINT('Ctrl Pts',(96.0229019644932,-1.1383326436948,-1.96050451688395));
#14504=CARTESIAN_POINT('Ctrl Pts',(96.1420526805125,1.03102069790592,-2.01900358813764));
#14505=CARTESIAN_POINT('Ctrl Pts',(96.2612033965315,2.25558900264279,-0.227370665610191));
#14506=CARTESIAN_POINT('Ctrl Pts',(96.3803541125507,1.41322815325176,1.77261539970789));
#14507=CARTESIAN_POINT('Ctrl Pts',(96.4995048285698,-0.724156952761073,
2.14824949114124));
#14508=CARTESIAN_POINT('Ctrl Pts',(96.618655544589,-2.19795435903126,0.555315949742211));
#14509=CARTESIAN_POINT('Ctrl Pts',(96.737806260608,-1.65763663227069,-1.54648632835516));
#14510=CARTESIAN_POINT('Ctrl Pts',(96.8569569766272,0.401671246589807,-2.23115202934803));
#14511=CARTESIAN_POINT('Ctrl Pts',(96.9761076926464,2.09290408651586,-0.871281615248694));
#14512=CARTESIAN_POINT('Ctrl Pts',(97.0952584086655,1.86628555009966,1.28699549882576));
#14513=CARTESIAN_POINT('Ctrl Pts',(97.2144091246847,-0.0705204402251945,
2.2659227779743));
#14514=CARTESIAN_POINT('Ctrl Pts',(97.3335598407038,-1.94270439443354,1.16845145570812));
#14515=CARTESIAN_POINT('Ctrl Pts',(97.452710556723,-2.03467380346316,-0.99974080767029));
#14516=CARTESIAN_POINT('Ctrl Pts',(97.571861272742,-0.262151676532748,-2.25181164073069));
#14517=CARTESIAN_POINT('Ctrl Pts',(97.6910119887613,1.75059548313724,-1.44041474023738));
#14518=CARTESIAN_POINT('Ctrl Pts',(97.8101627047803,2.15916881729827,0.690919091390331));
#14519=CARTESIAN_POINT('Ctrl Pts',(97.9293134207995,0.589168494652002,2.18912303000429));
#14520=CARTESIAN_POINT('Ctrl Pts',(98.0484641368186,-1.52072164337573,1.68130451244333));
#14521=CARTESIAN_POINT('Ctrl Pts',(98.1676148528378,-2.23708491093308,-0.36719244984327));
#14522=CARTESIAN_POINT('Ctrl Pts',(98.2867655688569,-0.903475400076174,
-2.07920928915298));
#14523=CARTESIAN_POINT('Ctrl Pts',(98.405916284876,1.25804184505795,-1.885924177408));
#14524=CARTESIAN_POINT('Ctrl Pts',(98.5250670008952,2.26674125125465,0.0355445698899612));
#14525=CARTESIAN_POINT('Ctrl Pts',(98.6442177169143,1.19829192833657,1.92444143411032));
#14526=CARTESIAN_POINT('Ctrl Pts',(98.7633684329336,-0.968222695796038,
2.0498597747611));
#14527=CARTESIAN_POINT('Ctrl Pts',(98.8825191489526,-2.24749823914522,0.296869594571833));
#14528=CARTESIAN_POINT('Ctrl Pts',(99.0016698649718,-1.46725778503147,-1.72815733426533));
#14529=CARTESIAN_POINT('Ctrl Pts',(99.1208205809907,0.657515695651045,-2.16957653402469));
#14530=CARTESIAN_POINT('Ctrl Pts',(99.2399712970101,2.17977230655602,-0.622875515384769));
#14531=CARTESIAN_POINT('Ctrl Pts',(99.359122013029,1.70456806378548,1.49458441122548));
#14532=CARTESIAN_POINT('Ctrl Pts',(99.4782727290483,-0.332618411870491,
2.24250567444778));
#14533=CARTESIAN_POINT('Ctrl Pts',(99.5974234450674,-2.06503482834595,0.935412859400004));
#14534=CARTESIAN_POINT('Ctrl Pts',(99.7165741610866,-1.90508274744876,-1.22870660728074));
#14535=CARTESIAN_POINT('Ctrl Pts',(99.8357248771057,0.000498669140674738,
-2.2671831486761));
#14536=CARTESIAN_POINT('Ctrl Pts',(99.9548755931249,1.90584282360693,-1.22752177995927));
#14537=CARTESIAN_POINT('Ctrl Pts',(100.074026309144,2.06431258653835,0.935825567833403));
#14538=CARTESIAN_POINT('Ctrl Pts',(100.193177025163,0.332012981233764,2.24394923878758));
#14539=CARTESIAN_POINT('Ctrl Pts',(100.312342589524,-1.70664597718939,1.49096848386471));
#14540=CARTESIAN_POINT('Ctrl Pts',(100.391791248547,-2.01926594988565,0.0850918326422001));
#14541=CARTESIAN_POINT('Ctrl Pts',(100.431523002228,-1.84334090146247,-0.528473926567276));
#14542=CARTESIAN_POINT('Ctrl Pts',(90.2679913357975,1.51880202537459,-1.394932151036));
#14543=CARTESIAN_POINT('Ctrl Pts',(90.3077082411372,1.98293998738585,-0.889578771495359));
#14544=CARTESIAN_POINT('Ctrl Pts',(90.3871420518166,2.35868305882058,0.612521864737925));
#14545=CARTESIAN_POINT('Ctrl Pts',(90.5062927678359,0.76083780342507,2.3177226439457));
#14546=CARTESIAN_POINT('Ctrl Pts',(90.6254434838548,-1.53470238783176,1.89359554348111));
#14547=CARTESIAN_POINT('Ctrl Pts',(90.7445941998742,-2.42363164136963,-0.263081080843427));
#14548=CARTESIAN_POINT('Ctrl Pts',(90.8637449158931,-1.09178346357141,-2.18001189517376));
#14549=CARTESIAN_POINT('Ctrl Pts',(90.9828956319124,1.24060025976444,-2.09860161216497));
#14550=CARTESIAN_POINT('Ctrl Pts',(91.1020463479315,2.43611367959052,-0.0944541698391232));
#14551=CARTESIAN_POINT('Ctrl Pts',(91.2211970639506,1.39929019753722,1.99641548545147));
#14552=CARTESIAN_POINT('Ctrl Pts',(91.3403477799699,-0.919794234654806,
2.25776746328333));
#14553=CARTESIAN_POINT('Ctrl Pts',(91.4594984959889,-2.39601254394569,0.450236457066652));
#14554=CARTESIAN_POINT('Ctrl Pts',(91.578649212008,-1.67662556563072,-1.7698940519589));
#14555=CARTESIAN_POINT('Ctrl Pts',(91.6977999280273,0.579153365510643,-2.3681556248105));
#14556=CARTESIAN_POINT('Ctrl Pts',(91.8169506440462,2.30421936760228,-0.796341981628139));
#14557=CARTESIAN_POINT('Ctrl Pts',(91.9361013600655,1.91779362852583,1.50520945367216));
#14558=CARTESIAN_POINT('Ctrl Pts',(92.0552520760845,-0.226019594709503,
2.42744739172543));
#14559=CARTESIAN_POINT('Ctrl Pts',(92.1744027921037,-2.16271766977255,1.12527288340679));
#14560=CARTESIAN_POINT('Ctrl Pts',(92.293553508123,-2.11759010291431,-1.20805583601235));
#14561=CARTESIAN_POINT('Ctrl Pts',(92.412704224142,-0.131989889838248,-2.43437161526355));
#14562=CARTESIAN_POINT('Ctrl Pts',(92.5318549401611,1.97456043014449,-1.42992928047227));
#14563=CARTESIAN_POINT('Ctrl Pts',(92.6510056561803,2.27170464615415,0.884841581403872));
#14564=CARTESIAN_POINT('Ctrl Pts',(92.7701563721993,0.487151991708878,2.38877992541277));
#14565=CARTESIAN_POINT('Ctrl Pts',(92.8893070882187,-1.74380674575924,1.70373843298149));
#14566=CARTESIAN_POINT('Ctrl Pts',(93.0084578042377,-2.37681257759652,-0.542539014376926));
#14567=CARTESIAN_POINT('Ctrl Pts',(93.1276085202568,-0.831804948016011,
-2.29165598128329));
#14568=CARTESIAN_POINT('Ctrl Pts',(93.2467592362759,1.47543458430119,-1.94079349701765));
#14569=CARTESIAN_POINT('Ctrl Pts',(93.3659099522951,2.43064644067022,0.188532465296514));
#14570=CARTESIAN_POINT('Ctrl Pts',(93.4850606683143,1.15851369401324,2.14509501665785));
#14571=CARTESIAN_POINT('Ctrl Pts',(93.6042113843334,-1.17523343663204,2.13598056626179));
#14572=CARTESIAN_POINT('Ctrl Pts',(93.7233621003525,-2.43204489760782,0.169541221976694));
#14573=CARTESIAN_POINT('Ctrl Pts',(93.8425128163716,-1.46023026706835,-1.95225873721671));
#14574=CARTESIAN_POINT('Ctrl Pts',(93.9616635323908,0.849679427422205,-2.28508894368612));
#14575=CARTESIAN_POINT('Ctrl Pts',(94.0808142484098,2.38097777997878,-0.523957461225582));
#14576=CARTESIAN_POINT('Ctrl Pts',(94.1999649644292,1.73044585095274,1.71730712653414));
#14577=CARTESIAN_POINT('Ctrl Pts',(94.3191156804481,-0.505795608835735,
2.38490197115348));
#14578=CARTESIAN_POINT('Ctrl Pts',(94.4382663964674,-2.27854673917708,0.867070566512739));
#14579=CARTESIAN_POINT('Ctrl Pts',(94.5574171124865,-1.96333118820778,-1.44530870589565));
#14580=CARTESIAN_POINT('Ctrl Pts',(94.6765678285056,0.151000454993279,-2.43326642037397));
#14581=CARTESIAN_POINT('Ctrl Pts',(94.7957185445247,2.12696148087597,-1.19147869003071));
#14582=CARTESIAN_POINT('Ctrl Pts',(94.9148692605438,2.15386233250742,1.14213119322304));
#14583=CARTESIAN_POINT('Ctrl Pts',(95.034019976563,0.207052173922958,2.42913894357677));
#14584=CARTESIAN_POINT('Ctrl Pts',(95.1531706925822,-1.92949209588725,1.49018349938391));
#14585=CARTESIAN_POINT('Ctrl Pts',(95.2723214086013,-2.29792902833395,-0.814314921064122));
#14586=CARTESIAN_POINT('Ctrl Pts',(95.3914721246205,-0.560638145466874,
-2.37260858124027));
#14587=CARTESIAN_POINT('Ctrl Pts',(95.5106228406395,1.69039851574195,-1.75674114994351));
#14588=CARTESIAN_POINT('Ctrl Pts',(95.6297735566587,2.39242337994864,0.468931744502973));
#14589=CARTESIAN_POINT('Ctrl Pts',(95.7489242726778,0.90212968468381,2.26489484125418));
#14590=CARTESIAN_POINT('Ctrl Pts',(95.868074988697,-1.4148386148164,1.98540129544429));
#14591=CARTESIAN_POINT('Ctrl Pts',(95.9872257047161,-2.43530689683827,-0.113432482734765));
#14592=CARTESIAN_POINT('Ctrl Pts',(96.1063764207353,-1.22415992518291,-2.10832139094206));
#14593=CARTESIAN_POINT('Ctrl Pts',(96.2255271367545,1.10875694148055,-2.17123113800578));
#14594=CARTESIAN_POINT('Ctrl Pts',(96.3446778527735,2.42565446929138,-0.244513814607605));
#14595=CARTESIAN_POINT('Ctrl Pts',(96.4638285687928,1.51978183172869,1.90626592947487));
#14596=CARTESIAN_POINT('Ctrl Pts',(96.5829792848118,-0.778756478629395,
2.31022184149429));
#14597=CARTESIAN_POINT('Ctrl Pts',(96.7021300008311,-2.36367432543604,0.597185308929409));
#14598=CARTESIAN_POINT('Ctrl Pts',(96.8212807168501,-1.7826180659763,-1.66308732205977));
#14599=CARTESIAN_POINT('Ctrl Pts',(96.9404314328693,0.431956200058963,-2.39937501260893));
#14600=CARTESIAN_POINT('Ctrl Pts',(97.0595821488882,2.25070353921181,-0.936973952951183));
#14601=CARTESIAN_POINT('Ctrl Pts',(97.1787328649075,2.00699856235737,1.38403156781969));
#14602=CARTESIAN_POINT('Ctrl Pts',(97.2978835809267,-0.0758374955757388,
2.4367673840503));
#14603=CARTESIAN_POINT('Ctrl Pts',(97.4170342969457,-2.08917918616753,1.25654961624997));
#14604=CARTESIAN_POINT('Ctrl Pts',(97.536185012965,-2.18808284627115,-1.075118629953));
#14605=CARTESIAN_POINT('Ctrl Pts',(97.6553357289841,-0.281917222095369,
-2.42159230424558));
#14606=CARTESIAN_POINT('Ctrl Pts',(97.7744864450031,1.88258576922385,-1.54901821572826));
#14607=CARTESIAN_POINT('Ctrl Pts',(97.8936371610223,2.32196445606787,0.743012570102993));
#14608=CARTESIAN_POINT('Ctrl Pts',(98.0127878770415,0.633590246513833,2.35417713747362));
#14609=CARTESIAN_POINT('Ctrl Pts',(98.1319385930606,-1.63538004773054,1.80807044194204));
#14610=CARTESIAN_POINT('Ctrl Pts',(98.2510893090799,-2.40575521783057,-0.394877792899667));
#14611=CARTESIAN_POINT('Ctrl Pts',(98.370240025099,-0.971595064314421,-2.23597619021765));
#14612=CARTESIAN_POINT('Ctrl Pts',(98.489390741118,1.35289488485932,-2.02811789041112));
#14613=CARTESIAN_POINT('Ctrl Pts',(98.6085414571373,2.43764756805906,0.0382245367890935));
#14614=CARTESIAN_POINT('Ctrl Pts',(98.7276921731562,1.28863998187605,2.06953924676429));
#14615=CARTESIAN_POINT('Ctrl Pts',(98.8468428891755,-1.04122413550308,2.20441379978537));
#14616=CARTESIAN_POINT('Ctrl Pts',(98.9659936051947,-2.41695368354768,0.319252779662519));
#14617=CARTESIAN_POINT('Ctrl Pts',(99.0851443212136,-1.57788515536039,-1.85845584305822));
#14618=CARTESIAN_POINT('Ctrl Pts',(99.204295037233,0.70709064635289,-2.33315688720802));
#14619=CARTESIAN_POINT('Ctrl Pts',(99.323445753252,2.3441213941193,-0.669838687781786));
#14620=CARTESIAN_POINT('Ctrl Pts',(99.4425964692711,1.83308800374897,1.60727213715557));
#14621=CARTESIAN_POINT('Ctrl Pts',(99.5617471852904,-0.357696963576656,
2.41158469262895));
#14622=CARTESIAN_POINT('Ctrl Pts',(99.6808979013095,-2.22073301241972,1.00594052390652));
#14623=CARTESIAN_POINT('Ctrl Pts',(99.8000486173285,-2.0487209661444,-1.32134784746082));
#14624=CARTESIAN_POINT('Ctrl Pts',(99.9191993333478,0.00053626747972391,
-2.43812278338156));
#14625=CARTESIAN_POINT('Ctrl Pts',(100.038350049367,2.04953835004185,-1.32007368728171));
#14626=CARTESIAN_POINT('Ctrl Pts',(100.157500765386,2.21995631548315,1.00638434946817));
#14627=CARTESIAN_POINT('Ctrl Pts',(100.276651481405,0.357045885065439,2.41313709791574));
#14628=CARTESIAN_POINT('Ctrl Pts',(100.395817045766,-1.8353225863476,1.60338357840087));
#14629=CARTESIAN_POINT('Ctrl Pts',(100.475265704789,-2.17151328113818,0.0915075325810447));
#14630=CARTESIAN_POINT('Ctrl Pts',(100.51499745847,-1.98232394767894,-0.568319467943805));
#14631=CARTESIAN_POINT('Ctrl Pts',(90.3514657920395,1.62528700848416,-1.49273247264503));
#14632=CARTESIAN_POINT('Ctrl Pts',(90.3911826973793,2.12196622486536,-0.951948177694941));
#14633=CARTESIAN_POINT('Ctrl Pts',(90.4706165080587,2.52405308169595,0.655466487757345));
#14634=CARTESIAN_POINT('Ctrl Pts',(90.5897672240778,0.814181030055862,2.48022088431535));
#14635=CARTESIAN_POINT('Ctrl Pts',(90.708917940097,-1.64230216391592,2.02635773769416));
#14636=CARTESIAN_POINT('Ctrl Pts',(90.828068656116,-2.5935552851911,-0.281526002552781));
#14637=CARTESIAN_POINT('Ctrl Pts',(90.9472193721352,-1.16832967679433,-2.33285507417793));
#14638=CARTESIAN_POINT('Ctrl Pts',(91.0663700881543,1.32758019230315,-2.24573702118577));
#14639=CARTESIAN_POINT('Ctrl Pts',(91.1855208041735,2.60691245368369,-0.101076461956154));
#14640=CARTESIAN_POINT('Ctrl Pts',(91.3046715201927,1.49739606687422,2.13638650583218));
#14641=CARTESIAN_POINT('Ctrl Pts',(91.4238222362116,-0.98428208225122,2.41606217594266));
#14642=CARTESIAN_POINT('Ctrl Pts',(91.5429729522309,-2.56399978060312,0.481803060695756));
#14643=CARTESIAN_POINT('Ctrl Pts',(91.6621236682501,-1.79417574139721,-1.89398339018722));
#14644=CARTESIAN_POINT('Ctrl Pts',(91.7812743842692,0.61975848409351,-2.53418978034607));
#14645=CARTESIAN_POINT('Ctrl Pts',(91.9004251002883,2.46577087750323,-0.852174447641754));
#14646=CARTESIAN_POINT('Ctrl Pts',(92.0195758163074,2.05225237873119,1.61074144571115));
#14647=CARTESIAN_POINT('Ctrl Pts',(92.1387265323266,-0.241866092358935,
2.597638562259));
#14648=CARTESIAN_POINT('Ctrl Pts',(92.2578772483458,-2.31434833044387,1.20416707895126));
#14649=CARTESIAN_POINT('Ctrl Pts',(92.3770279643649,-2.26605681718948,-1.29275404100813));
#14650=CARTESIAN_POINT('Ctrl Pts',(92.4961786803841,-0.141243855105126,
-2.605048251193));
#14651=CARTESIAN_POINT('Ctrl Pts',(92.6153293964031,2.11299916708316,-1.53018329168314));
#14652=CARTESIAN_POINT('Ctrl Pts',(92.7344801124224,2.43097651097537,0.946878857675728));
#14653=CARTESIAN_POINT('Ctrl Pts',(92.8536308284414,0.521306786568425,2.55626007474121));
#14654=CARTESIAN_POINT('Ctrl Pts',(92.9727815444605,-1.86606707249453,1.82318952353058));
#14655=CARTESIAN_POINT('Ctrl Pts',(93.0919322604797,-2.5434536821984,-0.580577058056743));
#14656=CARTESIAN_POINT('Ctrl Pts',(93.2110829764989,-0.890123764003973,
-2.45232665750241));
#14657=CARTESIAN_POINT('Ctrl Pts',(93.3302336925179,1.5788790254882,-2.07686479485395));
#14658=CARTESIAN_POINT('Ctrl Pts',(93.4493844085372,2.60106190026,0.201750696538821));
#14659=CARTESIAN_POINT('Ctrl Pts',(93.5685351245561,1.23973844159599,2.29549013254591));
#14660=CARTESIAN_POINT('Ctrl Pts',(93.6876858405755,-1.25763042488907,2.28573665739201));
#14661=CARTESIAN_POINT('Ctrl Pts',(93.8068365565945,-2.60255840464611,0.181427954978733));
#14662=CARTESIAN_POINT('Ctrl Pts',(93.9259872726136,-1.56260871582405,-2.08913387642833));
#14663=CARTESIAN_POINT('Ctrl Pts',(94.0451379886329,0.909251444028696,-2.44529919723268));
#14664=CARTESIAN_POINT('Ctrl Pts',(94.1642887046518,2.54791091178229,-0.560692730521131));
#14665=CARTESIAN_POINT('Ctrl Pts',(94.2834394206712,1.85176942975512,1.83770953402883));
#14666=CARTESIAN_POINT('Ctrl Pts',(94.4025901366902,-0.541257529457329,
2.55211023258152));
#14667=CARTESIAN_POINT('Ctrl Pts',(94.5217408527093,-2.43829831112787,0.927861896184007));
#14668=CARTESIAN_POINT('Ctrl Pts',(94.6408915687285,-2.10098262988481,-1.54664098657749));
#14669=CARTESIAN_POINT('Ctrl Pts',(94.7600422847476,0.161587273176848,-2.60386556979946));
#14670=CARTESIAN_POINT('Ctrl Pts',(94.8791930007667,2.27608523340055,-1.27501465196891));
#14671=CARTESIAN_POINT('Ctrl Pts',(94.9983437167859,2.30487213514503,1.22220734454978));
#14672=CARTESIAN_POINT('Ctrl Pts',(95.1174944328051,0.221568843557745,2.59944871078543));
#14673=CARTESIAN_POINT('Ctrl Pts',(95.2366451488242,-2.06477103929656,1.59466200422586));
#14674=CARTESIAN_POINT('Ctrl Pts',(95.3557958648434,-2.45903951520519,-0.871407490843901));
#14675=CARTESIAN_POINT('Ctrl Pts',(95.4749465808624,-0.599945140357085,
-2.53895493874968));
#14676=CARTESIAN_POINT('Ctrl Pts',(95.5940972968817,1.80891432911982,-1.87990832285632));
#14677=CARTESIAN_POINT('Ctrl Pts',(95.7132480129007,2.5601589761281,0.501809096559839));
#14678=CARTESIAN_POINT('Ctrl Pts',(95.8323987289199,0.965379050059475,2.42368926270382));
#14679=CARTESIAN_POINT('Ctrl Pts',(95.951549444939,-1.51403460184066,2.1246000981052));
#14680=CARTESIAN_POINT('Ctrl Pts',(96.0707001609581,-2.60604910645081,-0.121385366524927));
#14681=CARTESIAN_POINT('Ctrl Pts',(96.1898508769773,-1.30998720667102,-2.25613826500018));
#14682=CARTESIAN_POINT('Ctrl Pts',(96.3090015929964,1.18649318505518,-2.32345868787391));
#14683=CARTESIAN_POINT('Ctrl Pts',(96.4281523090155,2.59571993593996,-0.261656963605017));
#14684=CARTESIAN_POINT('Ctrl Pts',(96.5473030250347,1.62633551020562,2.03991645924184));
#14685=CARTESIAN_POINT('Ctrl Pts',(96.6664537410539,-0.833356004497719,
2.47219419184734));
#14686=CARTESIAN_POINT('Ctrl Pts',(96.7856044570729,-2.52939429184081,0.639054668116608));
#14687=CARTESIAN_POINT('Ctrl Pts',(96.9047551730922,-1.90759949968193,-1.77968831576439));
#14688=CARTESIAN_POINT('Ctrl Pts',(97.0239058891112,0.462241153528123,-2.56759799586982));
#14689=CARTESIAN_POINT('Ctrl Pts',(97.1430566051304,2.40850299190777,-1.00266629065368));
#14690=CARTESIAN_POINT('Ctrl Pts',(97.2622073211496,2.14771157461508,1.48106763681363));
#14691=CARTESIAN_POINT('Ctrl Pts',(97.3813580371687,-0.0811545509262814,
2.60761199012629));
#14692=CARTESIAN_POINT('Ctrl Pts',(97.5005087531878,-2.23565397790152,1.34464777679182));
#14693=CARTESIAN_POINT('Ctrl Pts',(97.6196594692069,-2.34149188907913,-1.15049645223572));
#14694=CARTESIAN_POINT('Ctrl Pts',(97.738810185226,-0.301682767657992,-2.59137296776048));
#14695=CARTESIAN_POINT('Ctrl Pts',(97.8579609012452,2.01457605531046,-1.65762169121913));
#14696=CARTESIAN_POINT('Ctrl Pts',(97.9771116172644,2.48476009483747,0.795106048815653));
#14697=CARTESIAN_POINT('Ctrl Pts',(98.0962623332834,0.678011998375664,2.51923124494296));
#14698=CARTESIAN_POINT('Ctrl Pts',(98.2154130493027,-1.75003845208536,1.93483637144075));
#14699=CARTESIAN_POINT('Ctrl Pts',(98.3345637653216,-2.57442552472806,-0.422563135956064));
#14700=CARTESIAN_POINT('Ctrl Pts',(98.453714481341,-1.03971472855267,-2.39274309128233));
#14701=CARTESIAN_POINT('Ctrl Pts',(98.57286519736,1.44774792466069,-2.17031160341423));
#14702=CARTESIAN_POINT('Ctrl Pts',(98.6920159133792,2.60855388486348,0.0409045036882235));
#14703=CARTESIAN_POINT('Ctrl Pts',(98.8111666293983,1.37898803541552,2.21463705941828));
#14704=CARTESIAN_POINT('Ctrl Pts',(98.9303173454174,-1.11422557521011,2.35896782480965));
#14705=CARTESIAN_POINT('Ctrl Pts',(99.0494680614366,-2.58640912795013,0.341635964753205));
#14706=CARTESIAN_POINT('Ctrl Pts',(99.1686187774558,-1.68851252568929,-1.98875435185111));
#14707=CARTESIAN_POINT('Ctrl Pts',(99.2877694934747,0.756665597054732,-2.49673724039136));
#14708=CARTESIAN_POINT('Ctrl Pts',(99.4069202094941,2.50847048168259,-0.7168018601788));
#14709=CARTESIAN_POINT('Ctrl Pts',(99.5260709255131,1.96160794371247,1.71995986308567));
#14710=CARTESIAN_POINT('Ctrl Pts',(99.6452216415324,-0.382775515282821,
2.58066371081011));
#14711=CARTESIAN_POINT('Ctrl Pts',(99.7643723575514,-2.37643119649348,1.07646818841304));
#14712=CARTESIAN_POINT('Ctrl Pts',(99.8835230735704,-2.19235918484003,-1.4139890876409));
#14713=CARTESIAN_POINT('Ctrl Pts',(100.00267378959,0.000573865818775353,
-2.60906241808703));
#14714=CARTESIAN_POINT('Ctrl Pts',(100.121824505609,2.19323387647676,-1.41262559460416));
#14715=CARTESIAN_POINT('Ctrl Pts',(100.240975221628,2.37560004442796,1.07694313110293));
#14716=CARTESIAN_POINT('Ctrl Pts',(100.360125937647,0.382078788897115,2.58232495704388));
#14717=CARTESIAN_POINT('Ctrl Pts',(100.479291502008,-1.96399919550581,1.71579867293704));
#14718=CARTESIAN_POINT('Ctrl Pts',(100.558740161031,-2.3237606123907,0.0979232325198861));
#14719=CARTESIAN_POINT('Ctrl Pts',(100.598471914712,-2.12130699389541,-0.608165009320335));
#14720=CARTESIAN_POINT('Ctrl Pts',(100.349869898682,0.479414994925344,2.1549256777475));
#14721=CARTESIAN_POINT('Ctrl Pts',(100.349869898682,0.426652918711055,2.16183856744942));
#14722=CARTESIAN_POINT('Ctrl Pts',(100.349869898682,0.373742092670611,2.16669187525483));
#14723=CARTESIAN_POINT('Ctrl Pts',(100.349869898682,0.320765011501748,2.16941984999741));
#14724=CARTESIAN_POINT('Ctrl Pts',(100.349869898682,0.243016014531923,2.173423417112));
#14725=CARTESIAN_POINT('Ctrl Pts',(100.349869898682,0.165123647545959,2.17285169457002));
#14726=CARTESIAN_POINT('Ctrl Pts',(100.349869898682,0.0874187568974411,
2.16789484102177));
#14727=CARTESIAN_POINT('Ctrl Pts',(100.349869898682,0.00882392244760108,
2.1628812172876));
#14728=CARTESIAN_POINT('Ctrl Pts',(100.349869898682,-0.0695801138469986,
2.1533809621849));
#14729=CARTESIAN_POINT('Ctrl Pts',(100.349869898682,-0.147434733752325,
2.13954043578746));
#14730=CARTESIAN_POINT('Ctrl Pts',(100.349869898682,-0.214042289520903,
2.12769934485407));
#14731=CARTESIAN_POINT('Ctrl Pts',(100.349869898682,-0.280247772593053,
2.11268039049434));
#14732=CARTESIAN_POINT('Ctrl Pts',(100.349869898682,-0.345809014350891,
2.09455055013339));
#14733=CARTESIAN_POINT('Ctrl Pts',(100.349869898682,-0.357788807056832,
2.09123774330587));
#14734=CARTESIAN_POINT('Ctrl Pts',(100.349869898682,-0.369741677068317,
2.08782245032933));
#14735=CARTESIAN_POINT('Ctrl Pts',(100.349869898682,-0.381659087973615,
2.08430749424005));
#14736=CARTESIAN_POINT('Ctrl Pts',(100.349869898682,-0.455832595007861,
2.06243054275413));
#14737=CARTESIAN_POINT('Ctrl Pts',(100.349869898682,-0.528720372107131,
2.03667310777151));
#14738=CARTESIAN_POINT('Ctrl Pts',(100.349869898682,-0.599998286878196,
2.00720683894348));
#14739=CARTESIAN_POINT('Ctrl Pts',(100.349869898682,-0.67107164032602,1.97782513570582));
#14740=CARTESIAN_POINT('Ctrl Pts',(100.349869898682,-0.74054525402381,1.94475525164764));
#14741=CARTESIAN_POINT('Ctrl Pts',(100.349869898682,-0.808069062026671,
1.90812458172216));
#14742=CARTESIAN_POINT('Ctrl Pts',(100.349869898682,-0.875592870029532,
1.87149391179667));
#14743=CARTESIAN_POINT('Ctrl Pts',(100.349869898682,-0.941167756187684,
1.83130189691578));
#14744=CARTESIAN_POINT('Ctrl Pts',(100.349869898682,-1.00440156213994,1.78764176103566));
#14745=CARTESIAN_POINT('Ctrl Pts',(100.349869898682,-1.02779687561394,1.77148833566689));
#14746=CARTESIAN_POINT('Ctrl Pts',(100.349869898682,-1.05087124668119,1.75485987879237));
#14747=CARTESIAN_POINT('Ctrl Pts',(100.349869898682,-1.07360298298094,1.73776016033235));
#14748=CARTESIAN_POINT('Ctrl Pts',(100.349869898682,-1.08344175669883,1.73035904242613));
#14749=CARTESIAN_POINT('Ctrl Pts',(100.349869898682,-1.09320813055687,1.72287579541148));
#14750=CARTESIAN_POINT('Ctrl Pts',(100.349869898682,-1.10289990339264,1.71531171169833));
#14751=CARTESIAN_POINT('Ctrl Pts',(100.349869898682,-1.16103677699879,1.6699379512698));
#14752=CARTESIAN_POINT('Ctrl Pts',(100.349869898682,-1.2165025157906,1.62165059609133));
#14753=CARTESIAN_POINT('Ctrl Pts',(100.349869898682,-1.26898476684194,1.57056955349251));
#14754=CARTESIAN_POINT('Ctrl Pts',(100.349869898682,-1.31991541638646,1.52099868664032));
#14755=CARTESIAN_POINT('Ctrl Pts',(100.349869898682,-1.36803686611545,1.46879626038254));
#14756=CARTESIAN_POINT('Ctrl Pts',(100.349869898682,-1.41302321703878,1.41404528435321));
#14757=CARTESIAN_POINT('Ctrl Pts',(100.349869898682,-1.44122551224844,1.37972146930035));
#14758=CARTESIAN_POINT('Ctrl Pts',(100.349869898682,-1.46819484161769,1.34439554642142));
#14759=CARTESIAN_POINT('Ctrl Pts',(100.349869898682,-1.4938411634309,1.30808394627534));
#14760=CARTESIAN_POINT('Ctrl Pts',(100.349869898682,-1.51638234254341,1.27616879334555));
#14761=CARTESIAN_POINT('Ctrl Pts',(100.349869898682,-1.53790129532058,1.24349204802205));
#14762=CARTESIAN_POINT('Ctrl Pts',(100.349869898682,-1.55838417110218,1.21010641100884));
#14763=CARTESIAN_POINT('Ctrl Pts',(100.349869898682,-1.56666347577931,1.19661173069051));
#14764=CARTESIAN_POINT('Ctrl Pts',(100.349869898682,-1.57477345721915,1.18300122799903));
#14765=CARTESIAN_POINT('Ctrl Pts',(100.349869898682,-1.58271301197484,1.16927838686893));
#14766=CARTESIAN_POINT('Ctrl Pts',(100.349869898682,-1.58818639734872,1.15981810852325));
#14767=CARTESIAN_POINT('Ctrl Pts',(100.349869898682,-1.59357707452811,1.15030730513012));
#14768=CARTESIAN_POINT('Ctrl Pts',(100.349869898682,-1.59888102457648,1.14075431016918));
#14769=CARTESIAN_POINT('Ctrl Pts',(100.349869898682,-1.63352381179489,1.07835885608061));
#14770=CARTESIAN_POINT('Ctrl Pts',(100.349869898682,-1.66452248560101,1.01407626559023));
#14771=CARTESIAN_POINT('Ctrl Pts',(100.349869898682,-1.69186815495165,0.948254794836713));
#14772=CARTESIAN_POINT('Ctrl Pts',(100.349869898682,-1.71949907166491,0.881746729043388));
#14773=CARTESIAN_POINT('Ctrl Pts',(100.349869898682,-1.74340046295035,0.813666407902212));
#14774=CARTESIAN_POINT('Ctrl Pts',(100.349869898682,-1.76351145670095,0.744362695384729));
#14775=CARTESIAN_POINT('Ctrl Pts',(100.349869898682,-1.7781837869541,0.693800949384702));
#14776=CARTESIAN_POINT('Ctrl Pts',(100.349869898682,-1.79083752896901,0.642587752416721));
#14777=CARTESIAN_POINT('Ctrl Pts',(100.349869898682,-1.8014315909638,0.59086023556729));
#14778=CARTESIAN_POINT('Ctrl Pts',(100.349869898682,-1.80788893402677,0.559331033429673));
#14779=CARTESIAN_POINT('Ctrl Pts',(100.349869898682,-1.81358077732546,0.527610800354083));
#14780=CARTESIAN_POINT('Ctrl Pts',(100.349869898682,-1.81849513035574,0.495731460558739));
#14781=CARTESIAN_POINT('Ctrl Pts',(100.349869898682,-1.8204466171093,0.483072193115112));
#14782=CARTESIAN_POINT('Ctrl Pts',(100.349869898682,-1.82227577945555,0.470385589327682));
#14783=CARTESIAN_POINT('Ctrl Pts',(100.349869898682,-1.82398080210467,0.457681045001224));
#14784=CARTESIAN_POINT('Ctrl Pts',(100.349869898682,-1.83331587287951,0.388123130031295));
#14785=CARTESIAN_POINT('Ctrl Pts',(100.349869898682,-1.83891415245773,0.31818414364734));
#14786=CARTESIAN_POINT('Ctrl Pts',(100.349869898682,-1.84071131029323,0.248192856383627));
#14787=CARTESIAN_POINT('Ctrl Pts',(100.349869898682,-1.84233496365157,0.184958795148171));
#14788=CARTESIAN_POINT('Ctrl Pts',(100.349869898682,-1.84085536620268,0.121681523415235));
#14789=CARTESIAN_POINT('Ctrl Pts',(100.349869898682,-1.83619001506039,0.0586141186189351));
#14790=CARTESIAN_POINT('Ctrl Pts',(100.349869898682,-1.83446389372289,0.0352799708131937));
#14791=CARTESIAN_POINT('Ctrl Pts',(100.349869898682,-1.83230134629332,0.0119746999217489));
#14792=CARTESIAN_POINT('Ctrl Pts',(100.349869898682,-1.82969704876561,-0.0112882622057297));
#14793=CARTESIAN_POINT('Ctrl Pts',(100.349869898682,-1.82803245302949,-0.0261573112120898));
#14794=CARTESIAN_POINT('Ctrl Pts',(100.349869898682,-1.82618711014688,-0.0410101441524755));
#14795=CARTESIAN_POINT('Ctrl Pts',(100.349869898682,-1.8241621629289,-0.0558261756737762));
#14796=CARTESIAN_POINT('Ctrl Pts',(100.349869898682,-1.81512268037633,-0.121965805016011));
#14797=CARTESIAN_POINT('Ctrl Pts',(100.349869898682,-1.80249961741287,-0.187453075266988));
#14798=CARTESIAN_POINT('Ctrl Pts',(100.349869898682,-1.78620616216217,-0.251987814719906));
#14799=CARTESIAN_POINT('Ctrl Pts',(100.349869898682,-1.77003269803824,-0.316047296102442));
#14800=CARTESIAN_POINT('Ctrl Pts',(100.349869898682,-1.75024259013915,-0.379169001454444));
#14801=CARTESIAN_POINT('Ctrl Pts',(100.349869898682,-1.72670765863932,-0.441032704914043));
#14802=CARTESIAN_POINT('Ctrl Pts',(100.349869898682,-1.72060689789584,-0.457069108228638));
#14803=CARTESIAN_POINT('Ctrl Pts',(100.349869898682,-1.71425427817139,-0.473020805173385));
#14804=CARTESIAN_POINT('Ctrl Pts',(100.349869898682,-1.7076471016036,-0.488881825071076));
#14805=CARTESIAN_POINT('Ctrl Pts',(90.3498698986825,0.431841315399936,1.72595542684201));
#14806=CARTESIAN_POINT('Ctrl Pts',(90.3498698986825,0.474841144465498,1.72062771663674));
#14807=CARTESIAN_POINT('Ctrl Pts',(90.3498698986825,0.517549233669023,1.71363307981672));
#14808=CARTESIAN_POINT('Ctrl Pts',(90.3498698986825,0.559872741940156,1.70495472032253));
#14809=CARTESIAN_POINT('Ctrl Pts',(90.3498698986825,0.624504400694465,1.69170211456541));
#14810=CARTESIAN_POINT('Ctrl Pts',(90.3498698986825,0.688239505726174,1.67452610531829));
#14811=CARTESIAN_POINT('Ctrl Pts',(90.3498698986825,0.750879107325786,1.65371126257901));
#14812=CARTESIAN_POINT('Ctrl Pts',(90.3498698986825,0.785762674423698,1.64211961855852));
#14813=CARTESIAN_POINT('Ctrl Pts',(90.3498698986825,0.820306563194663,1.62939848267447));
#14814=CARTESIAN_POINT('Ctrl Pts',(90.3498698986825,0.85447616357889,1.61559006912156));
#14815=CARTESIAN_POINT('Ctrl Pts',(90.3498698986825,0.867794193387564,1.61020806695471));
#14816=CARTESIAN_POINT('Ctrl Pts',(90.3498698986825,0.881057426269837,1.60465994112489));
#14817=CARTESIAN_POINT('Ctrl Pts',(90.3498698986825,0.894257109673279,1.59895090028477));
#14818=CARTESIAN_POINT('Ctrl Pts',(90.3498698986825,0.956519137646987,1.5720217346657));
#14819=CARTESIAN_POINT('Ctrl Pts',(90.3498698986825,1.0172384297205,1.54157364190433));
#14820=CARTESIAN_POINT('Ctrl Pts',(90.3498698986825,1.076208979192,1.50790448231969));
#14821=CARTESIAN_POINT('Ctrl Pts',(90.3498698986825,1.13685273154978,1.47328000969319));
#14822=CARTESIAN_POINT('Ctrl Pts',(90.3498698986825,1.19564793846948,1.43524882235765));
#14823=CARTESIAN_POINT('Ctrl Pts',(90.3498698986825,1.25236316356456,1.39408084780544));
#14824=CARTESIAN_POINT('Ctrl Pts',(90.3498698986825,1.26444032963692,1.38531437522781));
#14825=CARTESIAN_POINT('Ctrl Pts',(90.3498698986825,1.27642312556602,1.37640548370778));
#14826=CARTESIAN_POINT('Ctrl Pts',(90.3498698986825,1.2883092163036,1.36735649508758));
#14827=CARTESIAN_POINT('Ctrl Pts',(90.3498698986825,1.30329584009537,1.3559470425484));
#14828=CARTESIAN_POINT('Ctrl Pts',(90.3498698986825,1.31813332928754,1.34431096898487));
#14829=CARTESIAN_POINT('Ctrl Pts',(90.3498698986825,1.3327907185954,1.33247444330209));
#14830=CARTESIAN_POINT('Ctrl Pts',(90.3498698986825,1.38844900248271,1.28752778241633));
#14831=CARTESIAN_POINT('Ctrl Pts',(90.3498698986825,1.44157223405924,1.23965136935539));
#14832=CARTESIAN_POINT('Ctrl Pts',(90.3498698986825,1.49193815705566,1.18915424604306));
#14833=CARTESIAN_POINT('Ctrl Pts',(90.3498698986825,1.54319438475154,1.13776449883903));
#14834=CARTESIAN_POINT('Ctrl Pts',(90.3498698986825,1.59159590601355,1.08366009580108));
#14835=CARTESIAN_POINT('Ctrl Pts',(90.3498698986825,1.63689108900039,1.0271159092752));
#14836=CARTESIAN_POINT('Ctrl Pts',(90.3498698986825,1.66837534617324,0.987812575171713));
#14837=CARTESIAN_POINT('Ctrl Pts',(90.3498698986825,1.69835842343872,0.947329379839982));
#14838=CARTESIAN_POINT('Ctrl Pts',(90.3498698986825,1.72674724367579,0.905746523557564));
#14839=CARTESIAN_POINT('Ctrl Pts',(90.3498698986825,1.74998131073704,0.871714152243922));
#14840=CARTESIAN_POINT('Ctrl Pts',(90.3498698986825,1.77214742214936,0.836945004136101));
#14841=CARTESIAN_POINT('Ctrl Pts',(90.3498698986825,1.79318980004415,0.801478956440622));
#14842=CARTESIAN_POINT('Ctrl Pts',(90.3498698986825,1.79955534257003,0.790750100797062));
#14843=CARTESIAN_POINT('Ctrl Pts',(90.3498698986825,1.80581833349576,0.779956701588121));
#14844=CARTESIAN_POINT('Ctrl Pts',(90.3498698986825,1.81196923948669,0.76911428545529));
#14845=CARTESIAN_POINT('Ctrl Pts',(90.3498698986825,1.84875184073078,0.704276313663116));
#14846=CARTESIAN_POINT('Ctrl Pts',(90.3498698986825,1.88159981518027,0.637570922779393));
#14847=CARTESIAN_POINT('Ctrl Pts',(90.3498698986825,1.91026209575641,0.569292558053354));
#14848=CARTESIAN_POINT('Ctrl Pts',(90.3498698986825,1.91921179749468,0.547972865858888));
#14849=CARTESIAN_POINT('Ctrl Pts',(90.3498698986825,1.92775318680489,0.526499495860395));
#14850=CARTESIAN_POINT('Ctrl Pts',(90.3498698986825,1.93587796203386,0.504880604295509));
#14851=CARTESIAN_POINT('Ctrl Pts',(90.3498698986825,1.96125429222846,0.437357735621538));
#14852=CARTESIAN_POINT('Ctrl Pts',(90.3498698986825,1.98257013429095,0.368417422671431));
#14853=CARTESIAN_POINT('Ctrl Pts',(90.3498698986825,1.99995022625151,0.298378990239349));
#14854=CARTESIAN_POINT('Ctrl Pts',(90.3498698986825,2.01733031821208,0.228340557807268));
#14855=CARTESIAN_POINT('Ctrl Pts',(90.3498698986825,2.03077467779787,0.157203167161219));
#14856=CARTESIAN_POINT('Ctrl Pts',(90.3498698986825,2.04036047300214,0.0852645536046794));
#14857=CARTESIAN_POINT('Ctrl Pts',(90.3498698986825,2.04251882481325,0.0690667490876812));
#14858=CARTESIAN_POINT('Ctrl Pts',(90.3498698986825,2.04448173438142,0.0528237008312664));
#14859=CARTESIAN_POINT('Ctrl Pts',(90.3498698986825,2.04624695875265,0.0365679053387175));
#14860=CARTESIAN_POINT('Ctrl Pts',(90.3498698986825,2.05428355565145,-0.0374404064496148));
#14861=CARTESIAN_POINT('Ctrl Pts',(90.3498698986825,2.05824267691487,-0.111815486997948));
#14862=CARTESIAN_POINT('Ctrl Pts',(90.3498698986825,2.05827617422769,-0.186215580692539));
#14863=CARTESIAN_POINT('Ctrl Pts',(90.3498698986825,2.05831029294706,-0.261995865846831));
#14864=CARTESIAN_POINT('Ctrl Pts',(90.3498698986825,2.05427191440473,-0.337802955333537));
#14865=CARTESIAN_POINT('Ctrl Pts',(90.3498698986825,2.04627147701347,-0.413297832907415));
#14866=CARTESIAN_POINT('Ctrl Pts',(90.3498698986825,2.03818548362252,-0.489600046306389));
#14867=CARTESIAN_POINT('Ctrl Pts',(90.3498698986825,2.02605230738084,-0.565584325900605));
#14868=CARTESIAN_POINT('Ctrl Pts',(90.3498698986825,2.00993395345466,-0.640908956253526));
#14869=CARTESIAN_POINT('Ctrl Pts',(90.3498698986825,2.00386961328568,-0.669248958195093));
#14870=CARTESIAN_POINT('Ctrl Pts',(90.3498698986825,1.9972406228178,-0.697495589008317));
#14871=CARTESIAN_POINT('Ctrl Pts',(90.3498698986825,1.99004837701446,-0.725630494083073));
#14872=CARTESIAN_POINT('Ctrl Pts',(90.3498698986825,1.98683004789391,-0.738220078307771));
#14873=CARTESIAN_POINT('Ctrl Pts',(90.3498698986825,1.98349864718324,-0.750787978975287));
#14874=CARTESIAN_POINT('Ctrl Pts',(90.3498698986825,1.98005882552643,-0.763316755998211));
#14875=CARTESIAN_POINT('Ctrl Pts',(90.3498698986825,1.95909233732488,-0.839682475456528));
#14876=CARTESIAN_POINT('Ctrl Pts',(90.3498698986825,1.93406748684242,-0.914733173091299));
#14877=CARTESIAN_POINT('Ctrl Pts',(90.3498698986825,1.90511090692207,-0.988108398984206));
#14878=CARTESIAN_POINT('Ctrl Pts',(90.3498698986825,1.87610067909659,-1.06161956728362));
#14879=CARTESIAN_POINT('Ctrl Pts',(90.3498698986825,1.84314408917545,-1.13345011151776));
#14880=CARTESIAN_POINT('Ctrl Pts',(90.3498698986825,1.80631634283528,-1.20323986437882));
#14881=CARTESIAN_POINT('Ctrl Pts',(90.3498698986825,1.77027623606683,-1.27153701515267));
#14882=CARTESIAN_POINT('Ctrl Pts',(90.3498698986825,1.73052856007642,-1.33788070102088));
#14883=CARTESIAN_POINT('Ctrl Pts',(90.3498698986825,1.68709628885172,-1.40192061396105));
#14884=CARTESIAN_POINT('Ctrl Pts',(90.3498698986825,1.66663353523406,-1.43209248670082));
#14885=CARTESIAN_POINT('Ctrl Pts',(90.3498698986825,1.6453522241745,-1.46175270636413));
#14886=CARTESIAN_POINT('Ctrl Pts',(90.3498698986825,1.62325119196239,-1.49086269246791));
#14887=CARTESIAN_POINT('Origin',(90.3498698986825,-2.40291074888303E-16,
0.));
#14888=CARTESIAN_POINT('Ctrl Pts',(90.3498698986825,-0.214101726762246,
-2.19357617843498));
#14889=CARTESIAN_POINT('Ctrl Pts',(90.3498698986825,-0.253065554508825,
-2.18618780244257));
#14890=CARTESIAN_POINT('Ctrl Pts',(90.3498698986825,-0.291777125231032,
-2.17767057969178));
#14891=CARTESIAN_POINT('Ctrl Pts',(90.3498698986825,-0.330194078040925,
-2.16800471972977));
#14892=CARTESIAN_POINT('Ctrl Pts',(90.3498698986825,-0.406738639552015,
-2.14874579994817));
#14893=CARTESIAN_POINT('Ctrl Pts',(90.3498698986825,-0.482115441140247,
-2.12492954084353));
#14894=CARTESIAN_POINT('Ctrl Pts',(90.3498698986825,-0.556039436073237,
-2.09682490939037));
#14895=CARTESIAN_POINT('Ctrl Pts',(90.3498698986825,-0.591892015170574,
-2.08319437544683));
#14896=CARTESIAN_POINT('Ctrl Pts',(90.3498698986825,-0.627402453816474,
-2.06855445598174));
#14897=CARTESIAN_POINT('Ctrl Pts',(90.3498698986825,-0.662535477352669,
-2.05293241695311));
#14898=CARTESIAN_POINT('Ctrl Pts',(90.3498698986825,-0.679780447079454,
-2.0452643723898));
#14899=CARTESIAN_POINT('Ctrl Pts',(90.3498698986825,-0.696934454724005,
-2.03735967383535));
#14900=CARTESIAN_POINT('Ctrl Pts',(90.3498698986825,-0.713993138554701,
-2.02922138301724));
#14901=CARTESIAN_POINT('Ctrl Pts',(90.3498698986825,-0.726153529799593,
-2.02341995065616));
#14902=CARTESIAN_POINT('Ctrl Pts',(90.3498698986825,-0.738263467090767,
-2.01750071137784));
#14903=CARTESIAN_POINT('Ctrl Pts',(90.3498698986825,-0.750313634121258,
-2.01146892060574));
#14904=CARTESIAN_POINT('Ctrl Pts',(90.3498698986825,-0.82032062923626,-1.9764264563769));
#14905=CARTESIAN_POINT('Ctrl Pts',(90.3498698986825,-0.888389925919542,
-1.93755209171669));
#14906=CARTESIAN_POINT('Ctrl Pts',(90.3498698986825,-0.954242008533983,
-1.89510921263127));
#14907=CARTESIAN_POINT('Ctrl Pts',(90.3498698986825,-1.00375379709209,-1.86319795376679));
#14908=CARTESIAN_POINT('Ctrl Pts',(90.3498698986825,-1.05201168240331,-1.82926838600246));
#14909=CARTESIAN_POINT('Ctrl Pts',(90.3498698986825,-1.09888241457234,-1.79341950884159));
#14910=CARTESIAN_POINT('Ctrl Pts',(90.3498698986825,-1.12145931356828,-1.7761516651079));
#14911=CARTESIAN_POINT('Ctrl Pts',(90.3498698986825,-1.14371416086655,-1.75843836186296));
#14912=CARTESIAN_POINT('Ctrl Pts',(90.3498698986825,-1.16563083104683,-1.7402899773242));
#14913=CARTESIAN_POINT('Ctrl Pts',(90.3498698986825,-1.17633935367306,-1.73142264552315));
#14914=CARTESIAN_POINT('Ctrl Pts',(90.3498698986825,-1.18696862372855,-1.72245015180797));
#14915=CARTESIAN_POINT('Ctrl Pts',(90.3498698986825,-1.19751194217376,-1.7133777644169));
#14916=CARTESIAN_POINT('Ctrl Pts',(90.3498698986825,-1.25555020267444,-1.66343660163185));
#14917=CARTESIAN_POINT('Ctrl Pts',(90.3498698986825,-1.31081695979071,-1.61061924093467));
#14918=CARTESIAN_POINT('Ctrl Pts',(90.3498698986825,-1.36305428432945,-1.55517048740135));
#14919=CARTESIAN_POINT('Ctrl Pts',(90.3498698986825,-1.41423592356646,-1.50084232024226));
#14920=CARTESIAN_POINT('Ctrl Pts',(90.3498698986825,-1.46250982432993,-1.44398719082985));
#14921=CARTESIAN_POINT('Ctrl Pts',(90.3498698986825,-1.50759196670537,-1.38480940415008));
#14922=CARTESIAN_POINT('Ctrl Pts',(90.3498698986825,-1.55169882705472,-1.32691183683546));
#14923=CARTESIAN_POINT('Ctrl Pts',(90.3498698986825,-1.5927509135165,-1.26679030648339));
#14924=CARTESIAN_POINT('Ctrl Pts',(90.3498698986825,-1.63043591394233,-1.20462243846731));
#14925=CARTESIAN_POINT('Ctrl Pts',(90.3498698986825,-1.64313694391478,-1.18366991236745));
#14926=CARTESIAN_POINT('Ctrl Pts',(90.3498698986825,-1.6554550854017,-1.16248487188985));
#14927=CARTESIAN_POINT('Ctrl Pts',(90.3498698986825,-1.66737704460729,-1.14107396752518));
#14928=CARTESIAN_POINT('Ctrl Pts',(90.3498698986825,-1.6741165542006,-1.12897033649619));
#14929=CARTESIAN_POINT('Ctrl Pts',(90.3498698986825,-1.6807294444079,-1.11679452622328));
#14930=CARTESIAN_POINT('Ctrl Pts',(90.3498698986825,-1.68721321125448,-1.10454773595022));
#14931=CARTESIAN_POINT('Ctrl Pts',(90.3498698986825,-1.69280679091001,-1.09398236576683));
#14932=CARTESIAN_POINT('Ctrl Pts',(90.3498698986825,-1.69830255810943,-1.08336726810866));
#14933=CARTESIAN_POINT('Ctrl Pts',(90.3498698986825,-1.7036947776161,-1.07271211575908));
#14934=CARTESIAN_POINT('Ctrl Pts',(90.3498698986825,-1.73609336480919,-1.00869174677624));
#14935=CARTESIAN_POINT('Ctrl Pts',(90.3498698986825,-1.76480709242939,-0.943133950083889));
#14936=CARTESIAN_POINT('Ctrl Pts',(90.3498698986825,-1.78957581065152,-0.87622659827583));
#14937=CARTESIAN_POINT('Ctrl Pts',(90.3498698986825,-1.79745850834223,-0.854933190080087));
#14938=CARTESIAN_POINT('Ctrl Pts',(90.3498698986825,-1.80494126151048,-0.833502987156274));
#14939=CARTESIAN_POINT('Ctrl Pts',(90.3498698986825,-1.81201458800381,-0.811941804694479));
#14940=CARTESIAN_POINT('Ctrl Pts',(90.3498698986825,-1.83480258848545,-0.742478556138484));
#14941=CARTESIAN_POINT('Ctrl Pts',(90.3498698986825,-1.85334501760416,-0.671655559771788));
#14942=CARTESIAN_POINT('Ctrl Pts',(90.3498698986825,-1.86769676550017,-0.59983269942607));
#14943=CARTESIAN_POINT('Ctrl Pts',(90.3498698986825,-1.88119220525599,-0.532295205602301));
#14944=CARTESIAN_POINT('Ctrl Pts',(90.3498698986825,-1.89098144653587,-0.463872822082176));
#14945=CARTESIAN_POINT('Ctrl Pts',(90.3498698986825,-1.89706925925139,-0.394874641297999));
#14946=CARTESIAN_POINT('Ctrl Pts',(90.3498698986825,-1.89846100872211,-0.379100801649089));
#14947=CARTESIAN_POINT('Ctrl Pts',(90.3498698986825,-1.89965930467989,-0.363292543085898));
#14948=CARTESIAN_POINT('Ctrl Pts',(90.3498698986825,-1.90066249818027,-0.347482308863445));
#14949=CARTESIAN_POINT('Ctrl Pts',(90.3498698986825,-1.90518355320199,-0.276230911402284));
#14950=CARTESIAN_POINT('Ctrl Pts',(90.3498698986825,-1.90575774275495,-0.204834546578483));
#14951=CARTESIAN_POINT('Ctrl Pts',(90.3498698986825,-1.90246416417068,-0.13362783011485));
#14952=CARTESIAN_POINT('Ctrl Pts',(90.3498698986825,-1.89918981651357,-0.0628368836537749));
#14953=CARTESIAN_POINT('Ctrl Pts',(90.3498698986825,-1.89209235575437,0.00776763404536897));
#14954=CARTESIAN_POINT('Ctrl Pts',(90.3498698986825,-1.88120052059324,0.0778439104102741));
#14955=CARTESIAN_POINT('Ctrl Pts',(90.3498698986825,-1.87040101395053,0.147326160270228));
#14956=CARTESIAN_POINT('Ctrl Pts',(90.3498698986825,-1.85587082136304,0.216290003110817));
#14957=CARTESIAN_POINT('Ctrl Pts',(90.3498698986825,-1.83759523778481,0.284375112098316));
#14958=CARTESIAN_POINT('Ctrl Pts',(90.3498698986825,-1.83323021278473,0.300636874771509));
#14959=CARTESIAN_POINT('Ctrl Pts',(90.3498698986825,-1.82865134630036,0.316848351257569));
#14960=CARTESIAN_POINT('Ctrl Pts',(90.3498698986825,-1.82385810846295,0.333004312157768));
#14961=CARTESIAN_POINT('Ctrl Pts',(90.3498698986825,-1.81957084053952,0.347454864224923));
#14962=CARTESIAN_POINT('Ctrl Pts',(90.3498698986825,-1.81511076839976,0.361864640445972));
#14963=CARTESIAN_POINT('Ctrl Pts',(90.3498698986825,-1.81048601405767,0.376204364629576));
#14964=CARTESIAN_POINT('Ctrl Pts',(90.3498698986825,-1.78940703160402,0.441562818743621));
#14965=CARTESIAN_POINT('Ctrl Pts',(90.3498698986825,-1.76488237508185,0.505569487086397));
#14966=CARTESIAN_POINT('Ctrl Pts',(90.3498698986825,-1.73694698977818,0.567913160502579));
#14967=CARTESIAN_POINT('Ctrl Pts',(90.3498698986825,-1.70948750852825,0.629194754173614));
#14968=CARTESIAN_POINT('Ctrl Pts',(90.3498698986825,-1.67873208505158,0.68887029218068));
#14969=CARTESIAN_POINT('Ctrl Pts',(90.3498698986825,-1.64467466487717,0.746613674873613));
#14970=CARTESIAN_POINT('Ctrl Pts',(90.3498698986825,-1.61171139288394,0.802501960591362));
#14971=CARTESIAN_POINT('Ctrl Pts',(90.3498698986825,-1.57565443941957,0.856580748546144));
#14972=CARTESIAN_POINT('Ctrl Pts',(90.3498698986825,-1.53646769662718,0.908516538747599));
#14973=CARTESIAN_POINT('Ctrl Pts',(90.3498698986825,-1.52109669050737,0.928888360750091));
#14974=CARTESIAN_POINT('Ctrl Pts',(90.3498698986825,-1.50524382897348,0.948930000897413));
#14975=CARTESIAN_POINT('Ctrl Pts',(90.3498698986825,-1.48890580190332,0.968619417293828));
#14976=CARTESIAN_POINT('Ctrl Pts',(90.1012771668264,-1.84931296668343,1.20406753850538));
#14977=CARTESIAN_POINT('Ctrl Pts',(90.1410089197541,-2.25011488217789,0.588520614799742));
#14978=CARTESIAN_POINT('Ctrl Pts',(90.2204575780214,-2.38112656801824,-1.0636724344526));
#14979=CARTESIAN_POINT('Ctrl Pts',(90.3396231416286,-0.39278540449122,-2.58069915842425));
#14980=CARTESIAN_POINT('Ctrl Pts',(90.4587738576477,1.95479315758241,-1.7268362990989));
#14981=CARTESIAN_POINT('Ctrl Pts',(90.5779245736668,2.51126427646298,0.706567951536284));
#14982=CARTESIAN_POINT('Ctrl Pts',(90.697075289686,0.76642661853108,2.49393221007964));
#14983=CARTESIAN_POINT('Ctrl Pts',(90.8162260057051,-1.68068835309601,1.9952419118154));
#14984=CARTESIAN_POINT('Ctrl Pts',(90.9353767217243,-2.58771188198714,-0.331445932145255));
#14985=CARTESIAN_POINT('Ctrl Pts',(91.0545274377435,-1.12345126024935,-2.35459120720293));
#14986=CARTESIAN_POINT('Ctrl Pts',(91.1736781537624,1.37028833406634,-2.21999495043472));
#14987=CARTESIAN_POINT('Ctrl Pts',(91.2928288697817,2.60835478940657,-0.051132071917531));
#14988=CARTESIAN_POINT('Ctrl Pts',(91.4119795858008,1.45623058597522,2.16460903716915));
#14989=CARTESIAN_POINT('Ctrl Pts',(91.5311303018199,-1.03032282425427,2.39677979879221));
#14990=CARTESIAN_POINT('Ctrl Pts',(91.6502810178392,-2.57273105870856,0.432645731205606));
#14991=CARTESIAN_POINT('Ctrl Pts',(91.7694317338581,-1.75759399985632,-1.92795002038761));
#14992=CARTESIAN_POINT('Ctrl Pts',(91.8885824498775,0.668129948444457,-2.52185007357365));
#14993=CARTESIAN_POINT('Ctrl Pts',(92.0077331658964,2.48160708881929,-0.804830990088789));
#14994=CARTESIAN_POINT('Ctrl Pts',(92.1268838819157,2.02104135775696,1.64970253573836));
#14995=CARTESIAN_POINT('Ctrl Pts',(92.2460345979347,-0.291523684063095,
2.59251620548281));
#14996=CARTESIAN_POINT('Ctrl Pts',(92.3651853139538,-2.33694839666172,1.15965455820404));
#14997=CARTESIAN_POINT('Ctrl Pts',(92.4843360299731,-2.24088954394834,-1.33586696065266));
#14998=CARTESIAN_POINT('Ctrl Pts',(92.6034867459922,-0.0913715189856824,
-2.60725482022871));
#14999=CARTESIAN_POINT('Ctrl Pts',(92.7226374620113,2.141875615255,-1.48946142052775));
#15000=CARTESIAN_POINT('Ctrl Pts',(92.8417881780305,2.41239587446518,0.993213277893959));
#15001=CARTESIAN_POINT('Ctrl Pts',(92.9609388940497,0.472295600424488,2.56574810393475));
#15002=CARTESIAN_POINT('Ctrl Pts',(93.0800896100686,-1.90059697085994,1.78713671113314));
#15003=CARTESIAN_POINT('Ctrl Pts',(93.199240326088,-2.53186051096024,-0.629133389884245));
#15004=CARTESIAN_POINT('Ctrl Pts',(93.318391042107,-0.843031029634389,-2.46889148241641));
#15005=CARTESIAN_POINT('Ctrl Pts',(93.4375417581261,1.61831747486931,-2.04625878612023));
#15006=CARTESIAN_POINT('Ctrl Pts',(93.5566924741453,2.59670628878377,0.251481448464151));
#15007=CARTESIAN_POINT('Ctrl Pts',(93.6758431901645,1.19558007283248,2.31877440872209));
#15008=CARTESIAN_POINT('Ctrl Pts',(93.7949939061835,-1.30112663483962,2.26123770295275));
#15009=CARTESIAN_POINT('Ctrl Pts',(93.9141446222028,-2.60553431480175,0.131595605998399));
#15010=CARTESIAN_POINT('Ctrl Pts',(94.0332953382218,-1.52233732430562,-2.11863530135582));
#15011=CARTESIAN_POINT('Ctrl Pts',(94.152446054241,0.95586708746203,-2.42743580352548));
#15012=CARTESIAN_POINT('Ctrl Pts',(94.2715967702601,2.55815414538899,-0.511833798764109));
#15013=CARTESIAN_POINT('Ctrl Pts',(94.3907474862793,1.81625377481591,1.87279168478371));
#15014=CARTESIAN_POINT('Ctrl Pts',(94.5098982022984,-0.589986984925512,
2.54126775975048));
#15015=CARTESIAN_POINT('Ctrl Pts',(94.6290489183177,-2.45558789482286,0.881030396710455));
#15016=CARTESIAN_POINT('Ctrl Pts',(94.7481996343365,-2.07098887716839,-1.58654704934119));
#15017=CARTESIAN_POINT('Ctrl Pts',(94.8673503503559,0.211379318771256,-2.60027791836263));
#15018=CARTESIAN_POINT('Ctrl Pts',(94.9865010663749,2.30004818560611,-1.23122086280996));
#15019=CARTESIAN_POINT('Ctrl Pts',(95.1056517823941,2.28104732840938,1.26607644109069));
#15020=CARTESIAN_POINT('Ctrl Pts',(95.2248024984132,0.171788352596476,2.60319327577509));
#15021=CARTESIAN_POINT('Ctrl Pts',(95.3439532144324,-2.09489041640805,1.55485067204866));
#15022=CARTESIAN_POINT('Ctrl Pts',(95.4631039304515,-2.44189761789554,-0.918293249917765));
#15023=CARTESIAN_POINT('Ctrl Pts',(95.5822546464707,-0.551250099524635,
-2.54995094009719));
#15024=CARTESIAN_POINT('Ctrl Pts',(95.7014053624896,1.84454037733229,-1.84493828230628));
#15025=CARTESIAN_POINT('Ctrl Pts',(95.8205560785091,2.55006978384011,0.550700069615015));
#15026=CARTESIAN_POINT('Ctrl Pts',(95.939706794528,0.918819938851015,2.44169948787694));
#15027=CARTESIAN_POINT('Ctrl Pts',(96.0588575105472,-1.55439877403927,2.09522574449468));
#15028=CARTESIAN_POINT('Ctrl Pts',(96.1780082265663,-2.60323026947166,-0.171226847295238));
#15029=CARTESIAN_POINT('Ctrl Pts',(96.2971589425855,-1.26656842698869,-2.28077418629858));
#15030=CARTESIAN_POINT('Ctrl Pts',(96.4163096586046,1.23072472038826,-2.30031370290016));
#15031=CARTESIAN_POINT('Ctrl Pts',(96.5354603746238,2.6002322639617,-0.211940186326234));
#15032=CARTESIAN_POINT('Ctrl Pts',(96.6546110906428,1.58699371878083,2.07064661535818));
#15033=CARTESIAN_POINT('Ctrl Pts',(96.7737618066621,-0.880500712968156,
2.45577787341633));
#15034=CARTESIAN_POINT('Ctrl Pts',(96.8929125226811,-2.54114044213503,0.590535115362907));
#15035=CARTESIAN_POINT('Ctrl Pts',(97.0120632387003,-1.87318340193992,-1.81584977680931));
#15036=CARTESIAN_POINT('Ctrl Pts',(97.1312139547194,0.511282000374004,-2.55826448690676));
#15037=CARTESIAN_POINT('Ctrl Pts',(97.2503646707386,2.42722956925394,-0.956390656252166));
#15038=CARTESIAN_POINT('Ctrl Pts',(97.3695153867577,2.11896361589558,1.52188030555377));
#15039=CARTESIAN_POINT('Ctrl Pts',(97.4886661027769,-0.131033596758635,
2.60556263857647));
#15040=CARTESIAN_POINT('Ctrl Pts',(97.607816818796,-2.26095700091368,1.30161434785459));
#15041=CARTESIAN_POINT('Ctrl Pts',(97.7269675348151,-2.31903223828938,-1.19507989366364));
#15042=CARTESIAN_POINT('Ctrl Pts',(97.8461182508343,-0.252041544049245,
-2.59665198133307));
#15043=CARTESIAN_POINT('Ctrl Pts',(97.9652689668533,2.04590967080785,-1.61875881577068));
#15044=CARTESIAN_POINT('Ctrl Pts',(98.0844196828726,2.46907326691131,0.842498489996876));
#15045=CARTESIAN_POINT('Ctrl Pts',(98.2035703988916,0.629679485185892,2.53172472437204));
#15046=CARTESIAN_POINT('Ctrl Pts',(98.3227211149109,-1.78672670610972,1.9009824575361));
#15047=CARTESIAN_POINT('Ctrl Pts',(98.4418718309298,-2.5658499372617,-0.471742265797349));
#15048=CARTESIAN_POINT('Ctrl Pts',(98.5610225469492,-0.993733561394519,
-2.41218138425575));
#15049=CARTESIAN_POINT('Ctrl Pts',(98.6801732629682,1.48899930931111,-2.14219723795793));
#15050=CARTESIAN_POINT('Ctrl Pts',(98.7993239789874,2.60727462778386,0.0908099360674505));
#15051=CARTESIAN_POINT('Ctrl Pts',(98.9184746950065,1.33634996509571,2.24059976275692));
#15052=CARTESIAN_POINT('Ctrl Pts',(99.0376254110257,-1.15914982504648,2.33720163580698));
#15053=CARTESIAN_POINT('Ctrl Pts',(99.1567761270448,-2.59245452524983,0.292076583639263));
#15054=CARTESIAN_POINT('Ctrl Pts',(99.2759268430639,-1.65013591906561,-2.02067294410637));
#15055=CARTESIAN_POINT('Ctrl Pts',(99.3950775590831,0.804290694920273,-2.4818055857093));
#15056=CARTESIAN_POINT('Ctrl Pts',(99.5142282751021,2.52171586070367,-0.668624190400465));
#15057=CARTESIAN_POINT('Ctrl Pts',(99.6333789911213,1.9283092486174,1.75707912986123));
#15058=CARTESIAN_POINT('Ctrl Pts',(99.7525297071405,-0.432051285021002,
2.57302143737229));
#15059=CARTESIAN_POINT('Ctrl Pts',(99.8716804231596,-2.39663622909211,1.0304471465245));
#15060=CARTESIAN_POINT('Ctrl Pts',(99.9908311391787,-2.16476570723772,-1.45498086777256));
#15061=CARTESIAN_POINT('Ctrl Pts',(100.109981855198,0.0502481845584496,
-2.60993556246539));
#15062=CARTESIAN_POINT('Ctrl Pts',(100.229132571217,2.22042935661311,-1.36750819077076));
#15063=CARTESIAN_POINT('Ctrl Pts',(100.308566381897,2.30790711033604,0.287109651903352));
#15064=CARTESIAN_POINT('Ctrl Pts',(100.348283287236,1.99185752827467,0.949863530723621));
#15065=CARTESIAN_POINT('Ctrl Pts',(90.1847484975003,-1.72815398363866,1.12518224374417));
#15066=CARTESIAN_POINT('Ctrl Pts',(90.224480250428,-2.10269709202011,0.54996329082341));
#15067=CARTESIAN_POINT('Ctrl Pts',(90.3039289086954,-2.22512545913109,-0.993985219377189));
#15068=CARTESIAN_POINT('Ctrl Pts',(90.4230944723026,-0.367051804489291,
-2.41162291702421));
#15069=CARTESIAN_POINT('Ctrl Pts',(90.5422451883216,1.82672356887439,-1.61370145732095));
#15070=CARTESIAN_POINT('Ctrl Pts',(90.6613959043407,2.34673710806346,0.660276676883258));
#15071=CARTESIAN_POINT('Ctrl Pts',(90.78054662036,0.71621366304295,2.33054056366851));
#15072=CARTESIAN_POINT('Ctrl Pts',(90.899697336379,-1.57057692504417,1.86452229576392));
#15073=CARTESIAN_POINT('Ctrl Pts',(91.0188480523982,-2.41817619728542,-0.309731028937152));
#15074=CARTESIAN_POINT('Ctrl Pts',(91.1379987684174,-1.04984759518864,-2.20032858032993));
#15075=CARTESIAN_POINT('Ctrl Pts',(91.2571494844365,1.28051297206727,-2.07455048786676));
#15076=CARTESIAN_POINT('Ctrl Pts',(91.3763002004557,2.43746667073877,-0.0477821198293046));
#15077=CARTESIAN_POINT('Ctrl Pts',(91.4954509164748,1.36082465952898,2.0227932199669));
#15078=CARTESIAN_POINT('Ctrl Pts',(91.6146016324938,-0.962820531325284,
2.23975315796098));
#15079=CARTESIAN_POINT('Ctrl Pts',(91.733752348513,-2.40417685272153,0.404300655084951));
#15080=CARTESIAN_POINT('Ctrl Pts',(91.8529030645321,-1.64244404662254,-1.80163907787028));
#15081=CARTESIAN_POINT('Ctrl Pts',(91.9720537805513,0.624356965421232,-2.35662936955536));
#15082=CARTESIAN_POINT('Ctrl Pts',(92.0912044965705,2.31902293101863,-0.752101946363442));
#15083=CARTESIAN_POINT('Ctrl Pts',(92.2103552125894,1.88863147364933,1.54162116435486));
#15084=CARTESIAN_POINT('Ctrl Pts',(92.3295059286088,-0.272424313793784,
2.42266576229539));
#15085=CARTESIAN_POINT('Ctrl Pts',(92.4486566446278,-2.18384165038965,1.08367900972386));
#15086=CARTESIAN_POINT('Ctrl Pts',(92.567807360647,-2.09407615803056,-1.24834673808803));
#15087=CARTESIAN_POINT('Ctrl Pts',(92.686958076666,-0.0853852524537151,
-2.43643876678157));
#15088=CARTESIAN_POINT('Ctrl Pts',(92.8061087926853,2.00154919348222,-1.39187835360143));
#15089=CARTESIAN_POINT('Ctrl Pts',(92.9252595087044,2.2543461359313,0.928142241858348));
#15090=CARTESIAN_POINT('Ctrl Pts',(93.0444102247236,0.441352836449495,2.39765139092715));
#15091=CARTESIAN_POINT('Ctrl Pts',(93.1635609407427,-1.7760780817828,1.67005124729668));
#15092=CARTESIAN_POINT('Ctrl Pts',(93.2827116567617,-2.36598396640256,-0.587915292628069));
#15093=CARTESIAN_POINT('Ctrl Pts',(93.401862372781,-0.787799284621054,-2.30714039612304));
#15094=CARTESIAN_POINT('Ctrl Pts',(93.5210130888001,1.51229231686137,-1.91219676522963));
#15095=CARTESIAN_POINT('Ctrl Pts',(93.6401638048192,2.42658132947023,0.235005472196508));
#15096=CARTESIAN_POINT('Ctrl Pts',(93.7593145208384,1.11725084009434,2.16685834349552));
#15097=CARTESIAN_POINT('Ctrl Pts',(93.8784652368574,-1.21588244809045,2.11309119370958));
#15098=CARTESIAN_POINT('Ctrl Pts',(93.9976159528767,-2.43483098142503,0.122974031347059));
#15099=CARTESIAN_POINT('Ctrl Pts',(94.1167666688958,-1.42260037042766,-1.9798314843819));
#15100=CARTESIAN_POINT('Ctrl Pts',(94.2359173849148,0.893242812215344,-2.26840071392186));
#15101=CARTESIAN_POINT('Ctrl Pts',(94.3550681009339,2.39055495568398,-0.478300663127559));
#15102=CARTESIAN_POINT('Ctrl Pts',(94.4742188169533,1.69726068696523,1.75009447772847));
#15103=CARTESIAN_POINT('Ctrl Pts',(94.5933695329723,-0.551333590723985,
2.37477489296004));
#15104=CARTESIAN_POINT('Ctrl Pts',(94.7125202489916,-2.29470840202001,0.823309097600963));
#15105=CARTESIAN_POINT('Ctrl Pts',(94.8316709650105,-1.93530664772684,-1.48260335213368));
#15106=CARTESIAN_POINT('Ctrl Pts',(94.9508216810298,0.197530660507136,-2.4299189613346));
#15107=CARTESIAN_POINT('Ctrl Pts',(95.0699723970489,2.14935898148411,-1.15055659974088));
#15108=CARTESIAN_POINT('Ctrl Pts',(95.189123113068,2.13160297822848,1.18312859136324));
#15109=CARTESIAN_POINT('Ctrl Pts',(95.3082738290871,0.16053352311411,2.43264331714503));
#15110=CARTESIAN_POINT('Ctrl Pts',(95.4274245451062,-1.95764226154465,1.45298358432161));
#15111=CARTESIAN_POINT('Ctrl Pts',(95.5465752611255,-2.281915052795,-0.858130649913704));
#15112=CARTESIAN_POINT('Ctrl Pts',(95.6657259771446,-0.515134578428419,
-2.38288918890517));
#15113=CARTESIAN_POINT('Ctrl Pts',(95.7848766931636,1.72369407368938,-1.72406590965131));
#15114=CARTESIAN_POINT('Ctrl Pts',(95.9040274091828,2.38300024652033,0.514620584098359));
#15115=CARTESIAN_POINT('Ctrl Pts',(96.023178125202,0.858622832467166,2.28172990339787));
#15116=CARTESIAN_POINT('Ctrl Pts',(96.1423288412211,-1.45256129271431,1.95795562038611));
#15117=CARTESIAN_POINT('Ctrl Pts',(96.2614795572402,-2.43267788717467,-0.16000880521043));
#15118=CARTESIAN_POINT('Ctrl Pts',(96.3806302732593,-1.18358834447416,-2.13134773120684));
#15119=CARTESIAN_POINT('Ctrl Pts',(96.4997809892786,1.15009296242373,-2.14960710323403));
#15120=CARTESIAN_POINT('Ctrl Pts',(96.6189317052976,2.42987629801246,-0.198054782446931));
#15121=CARTESIAN_POINT('Ctrl Pts',(96.7380824213169,1.48302075772449,1.93498680942938));
#15122=CARTESIAN_POINT('Ctrl Pts',(96.8572331373359,-0.822814116445383,
2.2948859340381));
#15123=CARTESIAN_POINT('Ctrl Pts',(96.9763838533551,-2.37465591664382,0.551845810027022));
#15124=CARTESIAN_POINT('Ctrl Pts',(97.0955345693742,-1.75046053127167,-1.69688315715983));
#15125=CARTESIAN_POINT('Ctrl Pts',(97.2146852853935,0.4777850161802,-2.39065806810298));
#15126=CARTESIAN_POINT('Ctrl Pts',(97.3338360014124,2.26820799122736,-0.893732079043964));
#15127=CARTESIAN_POINT('Ctrl Pts',(97.4529867174316,1.98013828917371,1.4221732935668));
#15128=CARTESIAN_POINT('Ctrl Pts',(97.5721374334508,-0.122448842520727,
2.43485744954859));
#15129=CARTESIAN_POINT('Ctrl Pts',(97.6912881494699,-2.11282888205345,1.21633820825914));
#15130=CARTESIAN_POINT('Ctrl Pts',(97.8104388654891,-2.16709928118526,-1.11678343050024));
#15131=CARTESIAN_POINT('Ctrl Pts',(97.9295895815082,-0.235528872742544,
-2.42653058000869));
#15132=CARTESIAN_POINT('Ctrl Pts',(98.0487402975273,1.91187052244181,-1.51270474301667));
#15133=CARTESIAN_POINT('Ctrl Pts',(98.1678910135465,2.30731027088445,0.787301634676153));
#15134=CARTESIAN_POINT('Ctrl Pts',(98.2870417295656,0.588425610128645,2.36585707596402));
#15135=CARTESIAN_POINT('Ctrl Pts',(98.4061924455848,-1.66966810402821,1.77643831304004));
#15136=CARTESIAN_POINT('Ctrl Pts',(98.5253431616039,-2.39774655257518,-0.440835753912708));
#15137=CARTESIAN_POINT('Ctrl Pts',(98.644493877623,-0.928628438635352,-2.25414569819225));
#15138=CARTESIAN_POINT('Ctrl Pts',(98.7636445936422,1.39144651791202,-2.0018497448574));
#15139=CARTESIAN_POINT('Ctrl Pts',(98.8827953096614,2.43645727663141,0.0848604620181749));
#15140=CARTESIAN_POINT('Ctrl Pts',(99.0019460256804,1.24879809817007,2.09380536204883));
#15141=CARTESIAN_POINT('Ctrl Pts',(99.1210967416997,-1.08320734449868,2.18407829840195));
#15142=CARTESIAN_POINT('Ctrl Pts',(99.2402474577186,-2.42260812308438,0.272940989782257));
#15143=CARTESIAN_POINT('Ctrl Pts',(99.359398173738,-1.54202615428187,-1.8882871968669));
#15144=CARTESIAN_POINT('Ctrl Pts',(99.4785488897569,0.751597048996372,-2.31920842325136));
#15145=CARTESIAN_POINT('Ctrl Pts',(99.5976996057762,2.35650394973185,-0.624818826782988));
#15146=CARTESIAN_POINT('Ctrl Pts',(99.7168503217953,1.80197477102092,1.64196290868155));
#15147=CARTESIAN_POINT('Ctrl Pts',(99.8360010378144,-0.403745154442039,
2.40444820703176));
#15148=CARTESIAN_POINT('Ctrl Pts',(99.9551517538334,-2.23961899432637,0.962936708538316));
#15149=CARTESIAN_POINT('Ctrl Pts',(100.074302469853,-2.02293962569051,-1.35965681745507));
#15150=CARTESIAN_POINT('Ctrl Pts',(100.193453185872,0.0469561409451712,
-2.43894387838727));
#15151=CARTESIAN_POINT('Ctrl Pts',(100.312603901891,2.07495643363217,-1.27791497172988));
#15152=CARTESIAN_POINT('Ctrl Pts',(100.392037712571,2.15670302347367,0.268299469920303));
#15153=CARTESIAN_POINT('Ctrl Pts',(100.43175461791,1.86135964238754,0.887632582535241));
#15154=CARTESIAN_POINT('Ctrl Pts',(90.2682198281743,-1.60699500059389,1.04629694898296));
#15155=CARTESIAN_POINT('Ctrl Pts',(90.3079515811019,-1.95527930186235,0.511405966847078));
#15156=CARTESIAN_POINT('Ctrl Pts',(90.3874002393695,-2.06912435024394,-0.924298004301774));
#15157=CARTESIAN_POINT('Ctrl Pts',(90.5065658029763,-0.341318204487364,
-2.24254667562417));
#15158=CARTESIAN_POINT('Ctrl Pts',(90.6257165189957,1.69865398016637,-1.50056661554299));
#15159=CARTESIAN_POINT('Ctrl Pts',(90.7448672350146,2.18220993966394,0.613985402230233));
#15160=CARTESIAN_POINT('Ctrl Pts',(90.8640179510338,0.666000707554823,2.16714891725738));
#15161=CARTESIAN_POINT('Ctrl Pts',(90.983168667053,-1.46046549699233,1.73380267971244));
#15162=CARTESIAN_POINT('Ctrl Pts',(91.1023193830721,-2.2486405125837,-0.288016125729047));
#15163=CARTESIAN_POINT('Ctrl Pts',(91.2214700990913,-0.976243930127919,
-2.04606595345694));
#15164=CARTESIAN_POINT('Ctrl Pts',(91.3406208151105,1.1907376100682,-1.92910602529881));
#15165=CARTESIAN_POINT('Ctrl Pts',(91.4597715311294,2.26657855207099,-0.0444321677410789));
#15166=CARTESIAN_POINT('Ctrl Pts',(91.5789222471488,1.26541873308275,1.88097740276464));
#15167=CARTESIAN_POINT('Ctrl Pts',(91.6980729631677,-0.89531823839629,2.08272651712975));
#15168=CARTESIAN_POINT('Ctrl Pts',(91.817223679187,-2.2356226467345,0.375955578964296));
#15169=CARTESIAN_POINT('Ctrl Pts',(91.9363743952059,-1.52729409338877,-1.67532813535295));
#15170=CARTESIAN_POINT('Ctrl Pts',(92.0555251112253,0.580583982398003,-2.19140866553707));
#15171=CARTESIAN_POINT('Ctrl Pts',(92.1746758272442,2.15643877321799,-0.699372902638098));
#15172=CARTESIAN_POINT('Ctrl Pts',(92.2938265432635,1.75622158954171,1.43353979297137));
#15173=CARTESIAN_POINT('Ctrl Pts',(92.4129772592825,-0.253324943524471,
2.25281531910798));
#15174=CARTESIAN_POINT('Ctrl Pts',(92.5321279753018,-2.03073490411758,1.0077034612437));
#15175=CARTESIAN_POINT('Ctrl Pts',(92.6512786913209,-1.94726277211276,-1.16082651552341));
#15176=CARTESIAN_POINT('Ctrl Pts',(92.77042940734,-0.0793989859217509,-2.26562271333442));
#15177=CARTESIAN_POINT('Ctrl Pts',(92.8895801233591,1.86122277170944,-1.2942952866751));
#15178=CARTESIAN_POINT('Ctrl Pts',(93.0087308393784,2.09629639739743,0.863071205822738));
#15179=CARTESIAN_POINT('Ctrl Pts',(93.1278815553974,0.410410072474505,2.22955467791957));
#15180=CARTESIAN_POINT('Ctrl Pts',(93.2470322714165,-1.65155919270567,1.55296578346024));
#15181=CARTESIAN_POINT('Ctrl Pts',(93.3661829874357,-2.20010742184487,-0.546697195371894));
#15182=CARTESIAN_POINT('Ctrl Pts',(93.4853337034548,-0.732567539607717,
-2.14538930982965));
#15183=CARTESIAN_POINT('Ctrl Pts',(93.6044844194739,1.40626715885344,-1.77813474433903));
#15184=CARTESIAN_POINT('Ctrl Pts',(93.7236351354933,2.25645637015669,0.218529495928864));
#15185=CARTESIAN_POINT('Ctrl Pts',(93.8427858515121,1.0389216073562,2.01494227826896));
#15186=CARTESIAN_POINT('Ctrl Pts',(93.9619365675316,-1.13063826134128,1.96494468446641));
#15187=CARTESIAN_POINT('Ctrl Pts',(94.0810872835504,-2.2641276480483,0.11435245669572));
#15188=CARTESIAN_POINT('Ctrl Pts',(94.2002379995699,-1.32286341654972,-1.84102766740798));
#15189=CARTESIAN_POINT('Ctrl Pts',(94.3193887155888,0.830618536968657,-2.10936562431824));
#15190=CARTESIAN_POINT('Ctrl Pts',(94.4385394316082,2.22295576597898,-0.444767527491008));
#15191=CARTESIAN_POINT('Ctrl Pts',(94.5576901476269,1.57826759911456,1.62739727067323));
#15192=CARTESIAN_POINT('Ctrl Pts',(94.6768408636463,-0.512680196522462,
2.20828202616961));
#15193=CARTESIAN_POINT('Ctrl Pts',(94.7959915796653,-2.13382890921714,0.76558779849147));
#15194=CARTESIAN_POINT('Ctrl Pts',(94.9151422956845,-1.79962441828529,-1.37865965492618));
#15195=CARTESIAN_POINT('Ctrl Pts',(95.0342930117036,0.183682002243022,-2.25956000430656));
#15196=CARTESIAN_POINT('Ctrl Pts',(95.1534437277228,1.99866977736211,-1.06989233667182));
#15197=CARTESIAN_POINT('Ctrl Pts',(95.272594443742,1.9821586280476,1.1001807416358));
#15198=CARTESIAN_POINT('Ctrl Pts',(95.3917451597611,0.149278693631744,2.26209335851495));
#15199=CARTESIAN_POINT('Ctrl Pts',(95.5108958757802,-1.82039410668127,1.35111649659456));
#15200=CARTESIAN_POINT('Ctrl Pts',(95.6300465917994,-2.12193248769446,-0.797968049909645));
#15201=CARTESIAN_POINT('Ctrl Pts',(95.7491973078186,-0.479019057332203,
-2.21582743771315));
#15202=CARTESIAN_POINT('Ctrl Pts',(95.8683480238375,1.60284777004647,-1.60319353699634));
#15203=CARTESIAN_POINT('Ctrl Pts',(95.9874987398567,2.21593070920054,0.478541098581703));
#15204=CARTESIAN_POINT('Ctrl Pts',(96.1066494558759,0.798425726083314,2.12176031891879));
#15205=CARTESIAN_POINT('Ctrl Pts',(96.2258001718951,-1.35072381138935,1.82068549627755));
#15206=CARTESIAN_POINT('Ctrl Pts',(96.3449508879141,-2.26212550487769,-0.148790763125627));
#15207=CARTESIAN_POINT('Ctrl Pts',(96.4641016039334,-1.10060826195961,-1.98192127611509));
#15208=CARTESIAN_POINT('Ctrl Pts',(96.5832523199524,1.0694612044592,-1.99890050356789));
#15209=CARTESIAN_POINT('Ctrl Pts',(96.7024030359715,2.25952033206322,-0.184169378567629));
#15210=CARTESIAN_POINT('Ctrl Pts',(96.8215537519909,1.37904779666815,1.79932700350057));
#15211=CARTESIAN_POINT('Ctrl Pts',(96.9407044680099,-0.765127519922608,
2.13399399465988));
#15212=CARTESIAN_POINT('Ctrl Pts',(97.0598551840291,-2.20817139115261,0.513156504691141));
#15213=CARTESIAN_POINT('Ctrl Pts',(97.1790059000482,-1.62773766060341,-1.57791653751034));
#15214=CARTESIAN_POINT('Ctrl Pts',(97.2981566160672,0.444288031986397,-2.22305164929921));
#15215=CARTESIAN_POINT('Ctrl Pts',(97.4173073320864,2.10918641320078,-0.831073501835764));
#15216=CARTESIAN_POINT('Ctrl Pts',(97.5364580481055,1.84131296245185,1.32246628157985));
#15217=CARTESIAN_POINT('Ctrl Pts',(97.6556087641247,-0.113864088282822,
2.26415226052072));
#15218=CARTESIAN_POINT('Ctrl Pts',(97.774759480144,-1.96470076319321,1.13106206866369));
#15219=CARTESIAN_POINT('Ctrl Pts',(97.8939101961629,-2.01516632408114,-1.03848696733685));
#15220=CARTESIAN_POINT('Ctrl Pts',(98.0130609121822,-0.219016201435841,
-2.25640917868432));
#15221=CARTESIAN_POINT('Ctrl Pts',(98.1322116282013,1.77783137407576,-1.40665067026268));
#15222=CARTESIAN_POINT('Ctrl Pts',(98.2513623442205,2.1455472748576,0.732104779355433));
#15223=CARTESIAN_POINT('Ctrl Pts',(98.3705130602396,0.547171735071399,2.19998942755601));
#15224=CARTESIAN_POINT('Ctrl Pts',(98.4896637762586,-1.55260950194669,1.65189416854399));
#15225=CARTESIAN_POINT('Ctrl Pts',(98.6088144922779,-2.22964316788868,-0.409929242028069));
#15226=CARTESIAN_POINT('Ctrl Pts',(98.727965208297,-0.863523315876183,-2.09611001212873));
#15227=CARTESIAN_POINT('Ctrl Pts',(98.8471159243161,1.29389372651294,-1.86150225175686));
#15228=CARTESIAN_POINT('Ctrl Pts',(98.9662666403352,2.26563992547896,0.0789109879689021));
#15229=CARTESIAN_POINT('Ctrl Pts',(99.0854173563544,1.16124623124442,1.94701096134075));
#15230=CARTESIAN_POINT('Ctrl Pts',(99.2045680723735,-1.00726486395089,2.03095496099691));
#15231=CARTESIAN_POINT('Ctrl Pts',(99.3237187883926,-2.25276172091894,0.253805395925249));
#15232=CARTESIAN_POINT('Ctrl Pts',(99.4428695044117,-1.43391638949813,-1.75590144962745));
#15233=CARTESIAN_POINT('Ctrl Pts',(99.5620202204309,0.69890340307247,-2.15661126079343));
#15234=CARTESIAN_POINT('Ctrl Pts',(99.68117093645,2.19129203876002,-0.581013463165512));
#15235=CARTESIAN_POINT('Ctrl Pts',(99.8003216524693,1.67564029342444,1.52684668750188));
#15236=CARTESIAN_POINT('Ctrl Pts',(99.9194723684883,-0.375439023863076,
2.23587497669124));
#15237=CARTESIAN_POINT('Ctrl Pts',(100.038623084508,-2.08260175956064,0.895426270552136));
#15238=CARTESIAN_POINT('Ctrl Pts',(100.157773800527,-1.88111354414331,-1.26433276713758));
#15239=CARTESIAN_POINT('Ctrl Pts',(100.276924516546,0.0436640973318916,
-2.26795219430915));
#15240=CARTESIAN_POINT('Ctrl Pts',(100.396075232565,1.92948351065122,-1.18832175268901));
#15241=CARTESIAN_POINT('Ctrl Pts',(100.475509043245,2.00549893661128,0.249489287937253));
#15242=CARTESIAN_POINT('Ctrl Pts',(100.515225948584,1.73086175650041,0.82540163434686));
#15243=CARTESIAN_POINT('Ctrl Pts',(90.3516911588482,-1.48583601754912,0.967411654221745));
#15244=CARTESIAN_POINT('Ctrl Pts',(90.3914229117759,-1.80786151170457,0.472848642870747));
#15245=CARTESIAN_POINT('Ctrl Pts',(90.4708715700433,-1.91312324135679,-0.854610789226363));
#15246=CARTESIAN_POINT('Ctrl Pts',(90.5900371336504,-0.315584604485434,
-2.07347043422413));
#15247=CARTESIAN_POINT('Ctrl Pts',(90.7091878496695,1.57058439145835,-1.38743177376504));
#15248=CARTESIAN_POINT('Ctrl Pts',(90.8283385656886,2.01768277126442,0.567694127577208));
#15249=CARTESIAN_POINT('Ctrl Pts',(90.9474892817076,0.615787752066693,2.00375727084625));
#15250=CARTESIAN_POINT('Ctrl Pts',(91.066639997727,-1.35035406894049,1.60308306366094));
#15251=CARTESIAN_POINT('Ctrl Pts',(91.185790713746,-2.07910482788197,-0.266301222520941));
#15252=CARTESIAN_POINT('Ctrl Pts',(91.3049414297653,-0.902640265067203,
-1.89180332658395));
#15253=CARTESIAN_POINT('Ctrl Pts',(91.4240921457842,1.10096224806914,-1.78366156273085));
#15254=CARTESIAN_POINT('Ctrl Pts',(91.5432428618034,2.09569043340321,-0.0410822156528534));
#15255=CARTESIAN_POINT('Ctrl Pts',(91.6623935778227,1.17001280663651,1.73916158556239));
#15256=CARTESIAN_POINT('Ctrl Pts',(91.7815442938416,-0.827815945467298,
1.92569987629852));
#15257=CARTESIAN_POINT('Ctrl Pts',(91.9006950098609,-2.06706844074748,0.347610502843638));
#15258=CARTESIAN_POINT('Ctrl Pts',(92.0198457258799,-1.41214414015499,-1.54901719283562));
#15259=CARTESIAN_POINT('Ctrl Pts',(92.1389964418991,0.536810999374776,-2.02618796151878));
#15260=CARTESIAN_POINT('Ctrl Pts',(92.2581471579182,1.99385461541733,-0.64664385891275));
#15261=CARTESIAN_POINT('Ctrl Pts',(92.3772978739375,1.62381170543408,1.32545842158787));
#15262=CARTESIAN_POINT('Ctrl Pts',(92.4964485899565,-0.234225573255156,
2.08296487592058));
#15263=CARTESIAN_POINT('Ctrl Pts',(92.6155993059758,-1.87762815784551,0.931727912763529));
#15264=CARTESIAN_POINT('Ctrl Pts',(92.7347500219948,-1.80044938619497,-1.07330629295879));
#15265=CARTESIAN_POINT('Ctrl Pts',(92.853900738014,-0.0734127193897878,
-2.09480665988727));
#15266=CARTESIAN_POINT('Ctrl Pts',(92.9730514540332,1.72089634993666,-1.19671221974878));
#15267=CARTESIAN_POINT('Ctrl Pts',(93.0922021700523,1.93824665886355,0.798000169787126));
#15268=CARTESIAN_POINT('Ctrl Pts',(93.2113528860714,0.379467308499514,2.06145796491198));
#15269=CARTESIAN_POINT('Ctrl Pts',(93.3305036020905,-1.52704030362853,1.43588031962378));
#15270=CARTESIAN_POINT('Ctrl Pts',(93.4496543181096,-2.03423087728717,-0.505479098115718));
#15271=CARTESIAN_POINT('Ctrl Pts',(93.5688050341289,-0.67733579459438,-1.98363822353627));
#15272=CARTESIAN_POINT('Ctrl Pts',(93.6879557501479,1.3002420008455,-1.64407272344841));
#15273=CARTESIAN_POINT('Ctrl Pts',(93.8071064661672,2.08633141084316,0.202053519661223));
#15274=CARTESIAN_POINT('Ctrl Pts',(93.9262571821861,0.960592374618062,1.86302621304239));
#15275=CARTESIAN_POINT('Ctrl Pts',(94.0454078982054,-1.04539407459211,1.81679817522325));
#15276=CARTESIAN_POINT('Ctrl Pts',(94.1645586142245,-2.0934243146716,0.10573088204438));
#15277=CARTESIAN_POINT('Ctrl Pts',(94.2837093302435,-1.22312646267178,-1.70222385043407));
#15278=CARTESIAN_POINT('Ctrl Pts',(94.4028600462628,0.767994261721968,-1.95033053471462));
#15279=CARTESIAN_POINT('Ctrl Pts',(94.5220107622818,2.05535657627397,-0.411234391854458));
#15280=CARTESIAN_POINT('Ctrl Pts',(94.6411614783011,1.45927451126389,1.504700063618));
#15281=CARTESIAN_POINT('Ctrl Pts',(94.7603121943202,-0.474026802320936,
2.04178915937917));
#15282=CARTESIAN_POINT('Ctrl Pts',(94.8794629103393,-1.97294941641427,0.707866499381977));
#15283=CARTESIAN_POINT('Ctrl Pts',(94.9986136263584,-1.66394218884373,-1.27471595771868));
#15284=CARTESIAN_POINT('Ctrl Pts',(95.1177643423775,0.169833343978903,-2.08920104727853));
#15285=CARTESIAN_POINT('Ctrl Pts',(95.2369150583968,1.84798057324012,-0.989228073602758));
#15286=CARTESIAN_POINT('Ctrl Pts',(95.3560657744157,1.83271427786672,1.01723289190835));
#15287=CARTESIAN_POINT('Ctrl Pts',(95.475216490435,0.138023864149379,2.09154339988488));
#15288=CARTESIAN_POINT('Ctrl Pts',(95.5943672064542,-1.68314595181788,1.2492494088675));
#15289=CARTESIAN_POINT('Ctrl Pts',(95.7135179224733,-1.96194992259393,-0.737805449905584));
#15290=CARTESIAN_POINT('Ctrl Pts',(95.8326686384925,-0.442903536235988,
-2.04876568652113));
#15291=CARTESIAN_POINT('Ctrl Pts',(95.9518193545115,1.48200146640357,-1.48232116434138));
#15292=CARTESIAN_POINT('Ctrl Pts',(96.0709700705307,2.04886117188075,0.442461613065045));
#15293=CARTESIAN_POINT('Ctrl Pts',(96.1901207865498,0.738228619699466,1.96179073443972));
#15294=CARTESIAN_POINT('Ctrl Pts',(96.3092715025689,-1.24888633006439,1.68341537216896));
#15295=CARTESIAN_POINT('Ctrl Pts',(96.4284222185881,-2.0915731225807,-0.13757272104082));
#15296=CARTESIAN_POINT('Ctrl Pts',(96.5475729346072,-1.01762817944508,-1.83249482102335));
#15297=CARTESIAN_POINT('Ctrl Pts',(96.6667236506264,0.988829446494665,-1.84819390390174));
#15298=CARTESIAN_POINT('Ctrl Pts',(96.7858743666454,2.08916436611398,-0.170283974688326));
#15299=CARTESIAN_POINT('Ctrl Pts',(96.9050250826647,1.27507483561182,1.66366719757177));
#15300=CARTESIAN_POINT('Ctrl Pts',(97.0241757986838,-0.707440923399836,
1.97310205528165));
#15301=CARTESIAN_POINT('Ctrl Pts',(97.1433265147031,-2.0416868656614,0.474467199355257));
#15302=CARTESIAN_POINT('Ctrl Pts',(97.262477230722,-1.50501478993517,-1.45894991786086));
#15303=CARTESIAN_POINT('Ctrl Pts',(97.3816279467414,0.410791047792594,-2.05544523049543));
#15304=CARTESIAN_POINT('Ctrl Pts',(97.5007786627603,1.95016483517421,-0.768414924627563));
#15305=CARTESIAN_POINT('Ctrl Pts',(97.6199293787795,1.70248763572999,1.22275926959289));
#15306=CARTESIAN_POINT('Ctrl Pts',(97.7390800947986,-0.105279334044914,
2.09344707149284));
#15307=CARTESIAN_POINT('Ctrl Pts',(97.8582308108178,-1.81657264433298,1.04578592906823));
#15308=CARTESIAN_POINT('Ctrl Pts',(97.9773815268368,-1.86323336697702,-0.960190504173446));
#15309=CARTESIAN_POINT('Ctrl Pts',(98.0965322428562,-0.20250353012914,-2.08628777735995));
#15310=CARTESIAN_POINT('Ctrl Pts',(98.215682958875,1.64379222570971,-1.30059659750868));
#15311=CARTESIAN_POINT('Ctrl Pts',(98.3348336748945,1.98378427883073,0.676907924034713));
#15312=CARTESIAN_POINT('Ctrl Pts',(98.4539843909134,0.505917860014153,2.03412177914799));
#15313=CARTESIAN_POINT('Ctrl Pts',(98.5731351069327,-1.43555089986518,1.52735002404793));
#15314=CARTESIAN_POINT('Ctrl Pts',(98.6922858229516,-2.06153978320217,-0.379022730143428));
#15315=CARTESIAN_POINT('Ctrl Pts',(98.8114365389709,-0.798418193117015,
-1.93807432606522));
#15316=CARTESIAN_POINT('Ctrl Pts',(98.9305872549901,1.19634093511385,-1.72115475865633));
#15317=CARTESIAN_POINT('Ctrl Pts',(99.0497379710091,2.09482257432651,0.0729615139196275));
#15318=CARTESIAN_POINT('Ctrl Pts',(99.1688886870284,1.07369436431878,1.80021656063267));
#15319=CARTESIAN_POINT('Ctrl Pts',(99.2880394030473,-0.931322383403096,
1.87783162359188));
#15320=CARTESIAN_POINT('Ctrl Pts',(99.4071901190665,-2.08291531875349,0.234669802068244));
#15321=CARTESIAN_POINT('Ctrl Pts',(99.5263408350856,-1.32580662471439,-1.62351570238799));
#15322=CARTESIAN_POINT('Ctrl Pts',(99.6454915511049,0.646209757148569,-1.99401409833549));
#15323=CARTESIAN_POINT('Ctrl Pts',(99.764642267124,2.02608012778821,-0.537208099548037));
#15324=CARTESIAN_POINT('Ctrl Pts',(99.8837929831432,1.54930581582797,1.41173046632221));
#15325=CARTESIAN_POINT('Ctrl Pts',(100.002943699162,-0.347132893284113,
2.06730174635073));
#15326=CARTESIAN_POINT('Ctrl Pts',(100.122094415182,-1.92558452479489,0.827915832565954));
#15327=CARTESIAN_POINT('Ctrl Pts',(100.241245131201,-1.73928746259611,-1.1690087168201));
#15328=CARTESIAN_POINT('Ctrl Pts',(100.36039584722,0.0403720537186134,-2.09696051023103));
#15329=CARTESIAN_POINT('Ctrl Pts',(100.479546563239,1.78401058767028,-1.09872853364812));
#15330=CARTESIAN_POINT('Ctrl Pts',(100.558980373919,1.85429484974891,0.230679105954203));
#15331=CARTESIAN_POINT('Ctrl Pts',(100.598697279258,1.60036387061328,0.76317068615848));
#15332=CARTESIAN_POINT('Ctrl Pts',(100.349869898682,-0.0938337030309702,
-1.77668351508385));
#15333=CARTESIAN_POINT('Ctrl Pts',(100.349869898683,-0.0511432819576765,
-1.78421672036904));
#15334=CARTESIAN_POINT('Ctrl Pts',(100.349869898683,-0.00826292637260691,
-1.79006544278202));
#15335=CARTESIAN_POINT('Ctrl Pts',(100.349869898683,0.0347219594181995,
-1.79419129823277));
#15336=CARTESIAN_POINT('Ctrl Pts',(100.349869898683,0.0995747997289633,
-1.80041612446577));
#15337=CARTESIAN_POINT('Ctrl Pts',(100.349869898683,0.164664857862779,-1.80272216545716));
#15338=CARTESIAN_POINT('Ctrl Pts',(100.349869898683,0.229725300885462,-1.80133298954642));
#15339=CARTESIAN_POINT('Ctrl Pts',(100.349869898683,0.29658102383718,-1.79990548067153));
#15340=CARTESIAN_POINT('Ctrl Pts',(100.349869898682,0.363406212846255,-1.79457604187652));
#15341=CARTESIAN_POINT('Ctrl Pts',(100.349869898682,0.429927457817016,-1.78553511431863));
#15342=CARTESIAN_POINT('Ctrl Pts',(100.349869898682,0.461888589270306,-1.78119126485725));
#15343=CARTESIAN_POINT('Ctrl Pts',(100.349869898682,0.493779720820322,-1.77598986775753));
#15344=CARTESIAN_POINT('Ctrl Pts',(100.349869898682,0.525570989728989,-1.76994792489328));
#15345=CARTESIAN_POINT('Ctrl Pts',(100.349869898682,0.54423944949515,-1.76639997694585));
#15346=CARTESIAN_POINT('Ctrl Pts',(100.349869898682,0.562873475889208,-1.76256213670072));
#15347=CARTESIAN_POINT('Ctrl Pts',(100.349869898682,0.581467005198565,-1.75843743329546));
#15348=CARTESIAN_POINT('Ctrl Pts',(100.349869898682,0.596154585183359,-1.75517920780366));
#15349=CARTESIAN_POINT('Ctrl Pts',(100.349869898682,0.61082035890722,-1.75174098890012));
#15350=CARTESIAN_POINT('Ctrl Pts',(100.349869898682,0.62543517443403,-1.74813099328806));
#15351=CARTESIAN_POINT('Ctrl Pts',(100.349869898682,0.693180732655042,-1.73139720917252));
#15352=CARTESIAN_POINT('Ctrl Pts',(100.349869898682,0.75993966088107,-1.71095435092334));
#15353=CARTESIAN_POINT('Ctrl Pts',(100.349869898682,0.825417690190425,-1.68703869995642));
#15354=CARTESIAN_POINT('Ctrl Pts',(100.349869898682,0.893547624512638,-1.66215444875285));
#15355=CARTESIAN_POINT('Ctrl Pts',(100.349869898682,0.960291802375473,-1.63351046803854));
#15356=CARTESIAN_POINT('Ctrl Pts',(100.349869898682,1.02532499042762,-1.60131499980194));
#15357=CARTESIAN_POINT('Ctrl Pts',(100.349869898682,1.09035817847978,-1.56911953156533));
#15358=CARTESIAN_POINT('Ctrl Pts',(100.349869898682,1.15368151098642,-1.5333722334378));
#15359=CARTESIAN_POINT('Ctrl Pts',(100.349869898682,1.21495958037596,-1.49422728705875));
#15360=CARTESIAN_POINT('Ctrl Pts',(100.349869898682,1.23197877907323,-1.48335527971492));
#15361=CARTESIAN_POINT('Ctrl Pts',(100.349869898682,1.24884009337816,-1.47222088111476));
#15362=CARTESIAN_POINT('Ctrl Pts',(100.349869898682,1.26553601308461,-1.46082671008785));
#15363=CARTESIAN_POINT('Ctrl Pts',(100.349869898682,1.27472938384657,-1.45455267184274));
#15364=CARTESIAN_POINT('Ctrl Pts',(100.349869898682,1.28386964618837,-1.44820182666909));
#15365=CARTESIAN_POINT('Ctrl Pts',(100.349869898682,1.29294880238568,-1.44177972141025));
#15366=CARTESIAN_POINT('Ctrl Pts',(100.349869898682,1.35324423929895,-1.39912998237398));
#15367=CARTESIAN_POINT('Ctrl Pts',(100.349869898682,1.4109355605661,-1.35328021420338));
#15368=CARTESIAN_POINT('Ctrl Pts',(100.349869898682,1.46570284855611,-1.30444825220194));
#15369=CARTESIAN_POINT('Ctrl Pts',(100.349869898682,1.52027452518399,-1.25579070246288));
#15370=CARTESIAN_POINT('Ctrl Pts',(100.349869898682,1.57194408034395,-1.20417182322692));
#15371=CARTESIAN_POINT('Ctrl Pts',(100.349869898682,1.6203801336666,-1.14975844255616));
#15372=CARTESIAN_POINT('Ctrl Pts',(100.349869898682,1.6488575513763,-1.11776672432027));
#15373=CARTESIAN_POINT('Ctrl Pts',(100.349869898682,1.67621688115302,-1.08480813782164));
#15374=CARTESIAN_POINT('Ctrl Pts',(100.349869898682,1.7023860920606,-1.05090953536258));
#15375=CARTESIAN_POINT('Ctrl Pts',(100.349869898682,1.73605338905413,-1.00729819680577));
#15376=CARTESIAN_POINT('Ctrl Pts',(100.349869898682,1.76775143347122,-0.96213131021098));
#15377=CARTESIAN_POINT('Ctrl Pts',(100.349869898682,1.79747650045067,-0.91554685912618));
#15378=CARTESIAN_POINT('Ctrl Pts',(100.349869898682,1.80400780711786,-0.905311143386069));
#15379=CARTESIAN_POINT('Ctrl Pts',(100.349869898682,1.81043884326635,-0.895014695114847));
#15380=CARTESIAN_POINT('Ctrl Pts',(100.349869898682,1.81676859411639,-0.884661460495994));
#15381=CARTESIAN_POINT('Ctrl Pts',(100.349869898682,1.85453363415377,-0.822891206158915));
#15382=CARTESIAN_POINT('Ctrl Pts',(100.349869898682,1.88871158707573,-0.759078616801623));
#15383=CARTESIAN_POINT('Ctrl Pts',(100.349869898682,1.91935392695043,-0.693587452891148));
#15384=CARTESIAN_POINT('Ctrl Pts',(100.349869898682,1.95064136899357,-0.626717527044545));
#15385=CARTESIAN_POINT('Ctrl Pts',(100.349869898682,1.97824312877486,-0.558096935083375));
#15386=CARTESIAN_POINT('Ctrl Pts',(100.349869898682,2.00217647139197,-0.488072928118889));
#15387=CARTESIAN_POINT('Ctrl Pts',(100.349869898682,2.02656984762121,-0.416702958019421));
#15388=CARTESIAN_POINT('Ctrl Pts',(100.349869898682,2.04715283797167,-0.343874285935347));
#15389=CARTESIAN_POINT('Ctrl Pts',(100.349869898682,2.0638992034507,-0.269924895638561));
#15390=CARTESIAN_POINT('Ctrl Pts',(100.349869898682,2.06724025486549,-0.255171323265874));
#15391=CARTESIAN_POINT('Ctrl Pts',(100.349869898682,2.07042844291392,-0.240373072421388));
#15392=CARTESIAN_POINT('Ctrl Pts',(100.349869898682,2.07346332983987,-0.22553273542015));
#15393=CARTESIAN_POINT('Ctrl Pts',(100.349869898682,2.07629732325714,-0.211674750461271));
#15394=CARTESIAN_POINT('Ctrl Pts',(100.349869898682,2.07899763861465,-0.197780066263574));
#15395=CARTESIAN_POINT('Ctrl Pts',(100.349869898682,2.08156385697012,-0.183850777550955));
#15396=CARTESIAN_POINT('Ctrl Pts',(100.349869898682,2.08418234040323,-0.169637796940341));
#15397=CARTESIAN_POINT('Ctrl Pts',(100.349869898682,2.08665986231497,-0.155395799266646));
#15398=CARTESIAN_POINT('Ctrl Pts',(100.349869898682,2.08899516018094,-0.141135229261458));
#15399=CARTESIAN_POINT('Ctrl Pts',(100.349869898682,2.10153910007024,-0.064535265060426));
#15400=CARTESIAN_POINT('Ctrl Pts',(100.349869898682,2.1099963385427,0.0126694023299449));
#15401=CARTESIAN_POINT('Ctrl Pts',(100.349869898682,2.11437309453932,0.0901070091513077));
#15402=CARTESIAN_POINT('Ctrl Pts',(100.349869898682,2.11878252606939,0.168122741669996));
#15403=CARTESIAN_POINT('Ctrl Pts',(100.349869898682,2.11905064378886,0.246375886230533));
#15404=CARTESIAN_POINT('Ctrl Pts',(100.349869898682,2.115135354418,0.324505766001785));
#15405=CARTESIAN_POINT('Ctrl Pts',(100.349869898682,2.11414398385949,0.344288636489207));
#15406=CARTESIAN_POINT('Ctrl Pts',(100.349869898682,2.11288414907923,0.364063658710017));
#15407=CARTESIAN_POINT('Ctrl Pts',(100.349869898682,2.11135463994526,0.383825055241076));
#15408=CARTESIAN_POINT('Ctrl Pts',(100.349869898682,2.11020352169231,0.398697607320423));
#15409=CARTESIAN_POINT('Ctrl Pts',(100.349869898682,2.108900401199,0.413552658108748));
#15410=CARTESIAN_POINT('Ctrl Pts',(100.349869898682,2.1074453999023,0.428386817866731));
#15411=CARTESIAN_POINT('Ctrl Pts',(100.349869898682,2.09968291124947,0.507527638604876));
#15412=CARTESIAN_POINT('Ctrl Pts',(100.349869898682,2.08760086542093,0.586080887213785));
#15413=CARTESIAN_POINT('Ctrl Pts',(100.349869898682,2.07117840523179,0.66367273374298));
#15414=CARTESIAN_POINT('Ctrl Pts',(100.349869898682,2.05490267436583,0.740571322441432));
#15415=CARTESIAN_POINT('Ctrl Pts',(100.349869898682,2.03436391310446,0.816526640041535));
#15416=CARTESIAN_POINT('Ctrl Pts',(100.349869898682,2.0094914935604,0.891179159993237));
#15417=CARTESIAN_POINT('Ctrl Pts',(100.349869898682,2.0030758752601,0.910435110236341));
#15418=CARTESIAN_POINT('Ctrl Pts',(100.349869898682,1.99637165302178,0.929604358635609));
#15419=CARTESIAN_POINT('Ctrl Pts',(100.349869898682,1.98937704260618,0.948680653513806));
#15420=CARTESIAN_POINT('Origin',(100.349869898682,0.,0.));
#15421=CARTESIAN_POINT('Origin',(33.1926516271063,0.,0.));
#15422=CARTESIAN_POINT('',(33.4926516271063,-5.13007994755883E-16,4.18902817623056));
#15423=CARTESIAN_POINT('Origin',(33.4926516271063,0.,0.));
#15424=CARTESIAN_POINT('',(33.1926516271063,-5.49747398730303E-16,4.48902817623056));
#15425=CARTESIAN_POINT('Origin',(33.1926516271063,-5.13007994755883E-16,
4.18902817623056));
#15426=CARTESIAN_POINT('Origin',(33.1926516271063,0.,0.));
#15427=CARTESIAN_POINT('Origin',(32.5726008112287,0.,0.));
#15428=CARTESIAN_POINT('',(31.6525499953511,-5.49747398730303E-16,4.48902817623056));
#15429=CARTESIAN_POINT('',(32.5726008112287,-5.49747398730304E-16,4.48902817623056));
#15430=CARTESIAN_POINT('Origin',(31.6525499953511,0.,0.));
#15431=CARTESIAN_POINT('Origin',(33.4926516271063,0.,-2.21164758166987));
#15432=CARTESIAN_POINT('Origin',(31.3525499953512,0.,0.));
#15433=CARTESIAN_POINT('',(31.6525499953511,-7.4821050118432E-16,6.1096023907077));
#15434=CARTESIAN_POINT('Origin',(31.6525499953511,0.,0.));
#15435=CARTESIAN_POINT('',(31.3524613125654,-7.84949903553507E-16,6.40960237759997));
#15436=CARTESIAN_POINT('Origin',(31.3525499953512,-7.4821050118432E-16,
6.1096023907077));
#15437=CARTESIAN_POINT('Origin',(31.3524613125654,-7.84949903553507E-16,
0.));
#15438=CARTESIAN_POINT('Origin',(31.0318089645314,0.,0.));
#15439=CARTESIAN_POINT('',(30.7109792509259,-7.84926680813535E-16,6.40941274953751));
#15440=CARTESIAN_POINT('',(31.0318089645314,-7.84938295393988E-16,6.40950758978419));
#15441=CARTESIAN_POINT('Origin',(30.7109792509259,-7.84926680813535E-16,
0.));
#15442=CARTESIAN_POINT('Origin',(31.6525499953511,0.,-4.48902817623056));
#15443=CARTESIAN_POINT('Origin',(30.7110679337117,0.,0.));
#15444=CARTESIAN_POINT('',(30.4110679337117,-7.48187278444348E-16,6.10941276264524));
#15445=CARTESIAN_POINT('Origin',(30.7110679337117,-7.48187278444348E-16,
6.10941276264524));
#15446=CARTESIAN_POINT('Origin',(30.4110679337117,0.,0.));
#15447=CARTESIAN_POINT('Origin',(30.4110679337117,0.,-6.40932409296331));
#15448=CARTESIAN_POINT('',(30.4110679337117,-2.70848713173399E-16,2.21164758166987));
#15449=CARTESIAN_POINT('Origin',(30.4110679337117,0.,0.));
#15450=CARTESIAN_POINT('Origin',(28.3729800631879,0.,0.));
#15451=CARTESIAN_POINT('',(28.6729800631879,-7.48102635692981E-16,6.1087216021292));
#15452=CARTESIAN_POINT('Origin',(28.6729800631879,0.,0.));
#15453=CARTESIAN_POINT('',(28.3728913804021,-7.84842038062168E-16,6.40872158902147));
#15454=CARTESIAN_POINT('Origin',(28.3729800631879,-7.48102635692982E-16,
6.1087216021292));
#15455=CARTESIAN_POINT('Origin',(28.3728913804021,-7.84842038062168E-16,
0.));
#15456=CARTESIAN_POINT('Origin',(28.2136282688352,0.,0.));
#15457=CARTESIAN_POINT('',(28.0541877916966,-7.84830500451046E-16,6.40862737727707));
#15458=CARTESIAN_POINT('',(28.2136282688352,-7.84836272467075E-16,6.40867450936473));
#15459=CARTESIAN_POINT('Origin',(28.0541877916966,-7.84830500451046E-16,
0.));
#15460=CARTESIAN_POINT('Origin',(28.6729800631879,0.,0.));
#15461=CARTESIAN_POINT('',(28.6729800631879,-2.70848713173399E-16,2.21164758166987));
#15462=CARTESIAN_POINT('Origin',(28.6729800631879,0.,0.));
#15463=CARTESIAN_POINT('Origin',(28.0542764744824,0.,0.));
#15464=CARTESIAN_POINT('Origin',(28.0542764744824,-7.4809109808186E-16,
6.1086273903848));
#15465=CARTESIAN_POINT('Origin',(25.1947388265965,0.,0.));
#15466=CARTESIAN_POINT('',(25.1946501438108,-7.84726980332233E-16,6.40778207135796));
#15467=CARTESIAN_POINT('Origin',(25.1947388265965,-7.47987577963046E-16,
6.10778208446569));
#15468=CARTESIAN_POINT('Origin',(25.1946501438108,-7.84726980332233E-16,
0.));
#15469=CARTESIAN_POINT('Origin',(25.0105689136245,0.,0.));
#15470=CARTESIAN_POINT('',(24.8263103178667,-7.84713645805033E-16,6.40767318668028));
#15471=CARTESIAN_POINT('',(25.0105689136245,-7.847203162791E-16,6.40772765523458));
#15472=CARTESIAN_POINT('Origin',(24.8263103178667,-7.84713645805033E-16,
0.));
#15473=CARTESIAN_POINT('Origin',(24.8263990006525,0.,0.));
#15474=CARTESIAN_POINT('',(24.5263990006525,-7.47974243435846E-16,6.10767319978801));
#15475=CARTESIAN_POINT('Origin',(24.8263990006525,-7.47974243435846E-16,
6.10767319978801));
#15476=CARTESIAN_POINT('Origin',(24.5263990006525,0.,0.));
#15477=CARTESIAN_POINT('Origin',(24.5263990006525,0.,-6.40758453010608));
#15478=CARTESIAN_POINT('',(24.5263990006525,-2.70848713173399E-16,2.21164758166987));
#15479=CARTESIAN_POINT('Origin',(24.5263990006525,0.,0.));
#15480=CARTESIAN_POINT('Origin',(22.4730782633311,0.,0.));
#15481=CARTESIAN_POINT('',(22.7730782633312,-7.47889049228833E-16,6.1069775362949));
#15482=CARTESIAN_POINT('Origin',(22.7730782633312,0.,0.));
#15483=CARTESIAN_POINT('',(22.4729895805454,-7.8462845159802E-16,6.40697752318717));
#15484=CARTESIAN_POINT('Origin',(22.4730782633311,-7.47889049228834E-16,
6.1069775362949));
#15485=CARTESIAN_POINT('Origin',(22.4729895805454,-7.8462845159802E-16,
0.));
#15486=CARTESIAN_POINT('Origin',(22.2310089528171,0.,0.));
#15487=CARTESIAN_POINT('',(21.9888509595172,-7.84610924957793E-16,6.40683440730886));
#15488=CARTESIAN_POINT('',(22.2310089528171,-7.84619691488374E-16,6.40690599146347));
#15489=CARTESIAN_POINT('Origin',(21.9888509595172,-7.84610924957793E-16,
0.));
#15490=CARTESIAN_POINT('Origin',(22.7730782633312,0.,-2.21164758166987));
#15491=CARTESIAN_POINT('',(22.7730782633312,-2.70848713173399E-16,2.21164758166987));
#15492=CARTESIAN_POINT('Origin',(22.7730782633312,0.,0.));
#15493=CARTESIAN_POINT('Origin',(21.9889396423029,0.,0.));
#15494=CARTESIAN_POINT('',(21.688939642303,-7.47871522588606E-16,6.10683442041659));
#15495=CARTESIAN_POINT('Origin',(21.9889396423029,-7.47871522588606E-16,
6.10683442041659));
#15496=CARTESIAN_POINT('Origin',(21.688939642303,0.,0.));
#15497=CARTESIAN_POINT('Origin',(21.688939642303,0.,-6.40674575073467));
#15498=CARTESIAN_POINT('',(21.688939642303,-5.41697426346798E-16,4.42329516333974));
#15499=CARTESIAN_POINT('Origin',(21.688939642303,0.,0.));
#15500=CARTESIAN_POINT('Origin',(21.1989257366328,0.,0.));
#15501=CARTESIAN_POINT('',(21.1989257366328,-5.41697426346798E-16,4.42329516333974));
#15502=CARTESIAN_POINT('Origin',(21.1989257366328,0.,0.));
#15503=CARTESIAN_POINT('',(20.8989257366328,-5.04958022372377E-16,4.12329516333974));
#15504=CARTESIAN_POINT('Origin',(21.1989257366328,-5.04958022372377E-16,
4.12329516333974));
#15505=CARTESIAN_POINT('Origin',(20.8989257366328,0.,0.));
#15506=CARTESIAN_POINT('Origin',(20.8989257366328,0.,-4.42329516333974));
#15507=CARTESIAN_POINT('Origin',(21.2939326894679,0.,0.));
#15508=CARTESIAN_POINT('',(21.2939326894679,-5.41697426346798E-16,4.42329516333974));
#15509=CARTESIAN_POINT('Origin',(23.6497386319918,0.,0.));
#15510=CARTESIAN_POINT('',(23.6497386319918,-2.70848713173399E-16,2.21164758166987));
#15511=CARTESIAN_POINT('Origin',(29.5420239984498,0.,0.));
#15512=CARTESIAN_POINT('',(29.5420239984498,-2.70848713173399E-16,2.21164758166987));
#28034=UNCERTAINTY_MEASURE_WITH_UNIT(LENGTH_MEASURE(0.01),#28056,
'DISTANCE_ACCURACY_VALUE',
'Maximum model space distance between geometric entities at asserted c
onnectivities');
#28043=UNCERTAINTY_MEASURE_WITH_UNIT(LENGTH_MEASURE(0.01),#28056,
'DISTANCE_ACCURACY_VALUE',
'Maximum model space distance between geometric entities at asserted c
onnectivities');
#28046=(
GEOMETRIC_REPRESENTATION_CONTEXT(3)
GLOBAL_UNCERTAINTY_ASSIGNED_CONTEXT((#28034))
GLOBAL_UNIT_ASSIGNED_CONTEXT((#28056,#28058,#28059))
REPRESENTATION_CONTEXT('','3D')
);
#28055=(
GEOMETRIC_REPRESENTATION_CONTEXT(3)
GLOBAL_UNCERTAINTY_ASSIGNED_CONTEXT((#28043))
GLOBAL_UNIT_ASSIGNED_CONTEXT((#28056,#28058,#28059))
REPRESENTATION_CONTEXT('','3D')
);
#28056=(
LENGTH_UNIT()
NAMED_UNIT(*)
SI_UNIT(.MILLI.,.METRE.)
);
#28058=(
NAMED_UNIT(*)
PLANE_ANGLE_UNIT()
SI_UNIT($,.RADIAN.)
);
#28059=(
NAMED_UNIT(*)
SI_UNIT($,.STERADIAN.)
SOLID_ANGLE_UNIT()
);
#28062=SHAPE_DEFINITION_REPRESENTATION(#28073,#28094);
#28073=PRODUCT_DEFINITION_SHAPE('',$,#28106);
#28094=SHAPE_REPRESENTATION('',(#3851),#28046);
#28103=PRODUCT_DEFINITION_CONTEXT('part definition',#28138,'design');
#28106=PRODUCT_DEFINITION('Shaft','Shaft',#28117,#28103);
#28117=PRODUCT_DEFINITION_FORMATION('',$,#28142);
#28138=APPLICATION_CONTEXT(
'Core Data for Automotive Mechanical Design Process');
#28139=PRODUCT_CONTEXT('part definition',#28138,'mechanical');
#28142=PRODUCT('Shaft','Shaft',$,(#28139));
#28152=PRESENTATION_STYLE_ASSIGNMENT((#28155));
#28155=SURFACE_STYLE_USAGE(.BOTH.,#28158);
#28158=SURFACE_SIDE_STYLE('',(#28161));
#28161=SURFACE_STYLE_FILL_AREA(#28164);
#28164=FILL_AREA_STYLE('Opaque(160,160,160)',(#28167));
#28167=FILL_AREA_STYLE_COLOUR('Opaque(160,160,160)',#28170);
#28170=COLOUR_RGB('Opaque(160,160,160)', 0.66274510, 0.83137255, 0.94901961);
ENDSEC;
END-ISO-10303-21;
